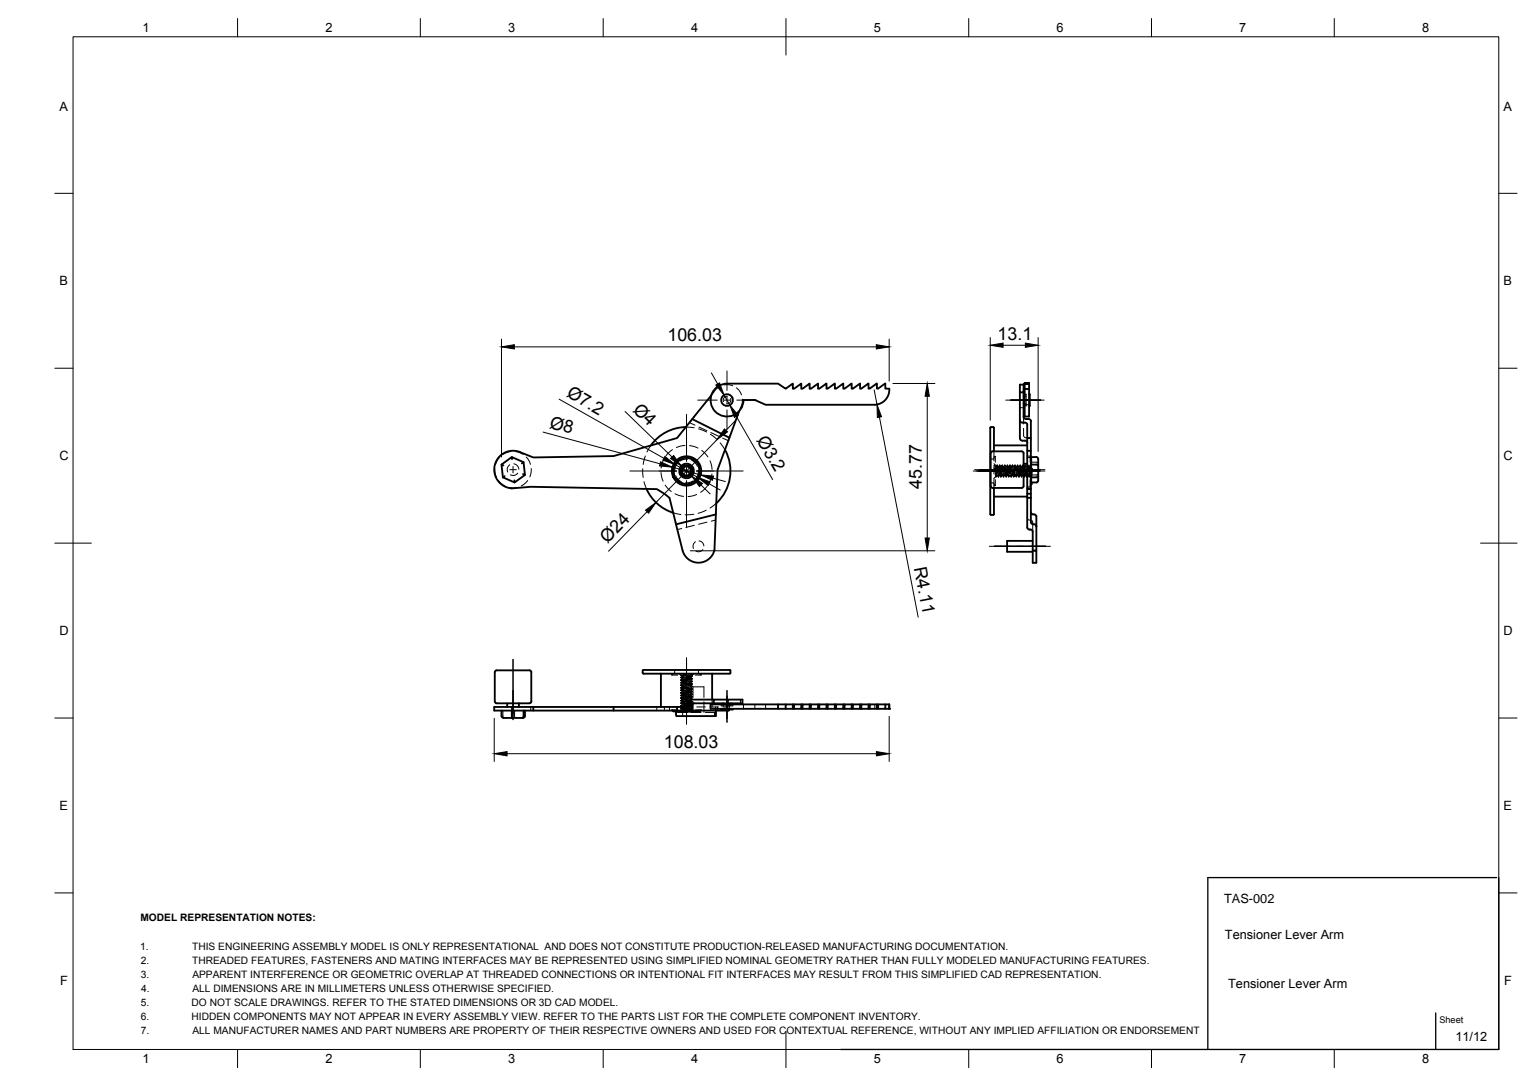
ISO-10303-21;
HEADER;
/* Generated by software containing ST-Developer
 * from STEP Tools, Inc. (www.steptools.com) 
 */

FILE_DESCRIPTION(
/* description */ ('STEP AP214'),
/* implementation_level */ '2;1');

FILE_NAME(
/* name */ 'Tensioner Lever Arm.step',
/* time_stamp */ '2026-11-04T19:38:14-08:00',
/* author */ (''),
/* organization */ (''),
/* preprocessor_version */ 'ST-DEVELOPER v20.2',
/* originating_system */ 'Autodesk Translation Framework v15.17.0.0',
/* authorisation */ '');

FILE_SCHEMA (('AUTOMOTIVE_DESIGN { 1 0 10303 214 3 1 1 }'));
ENDSEC;

DATA;
#10=MECHANICAL_DESIGN_GEOMETRIC_PRESENTATION_REPRESENTATION('',(#478),#36668);
#51=ORIENTED_CLOSED_SHELL('',*,#17801,.F.);
#52=BREP_WITH_VOIDS('Body1',#17802,(#51));
#136=(
BOUNDED_CURVE()
B_SPLINE_CURVE(2,(#34733,#34734,#34735,#34736,#34737,#34738,#34739),
 .UNSPECIFIED.,.F.,.F.)
B_SPLINE_CURVE_WITH_KNOTS((3,2,2,3),(0.964285714285714,0.976190476190476,
0.988095238095238,1.),.UNSPECIFIED.)
CURVE()
GEOMETRIC_REPRESENTATION_ITEM()
RATIONAL_B_SPLINE_CURVE((1.,0.866025403784439,1.,0.866025403784439,1.,0.866025403784439,
1.))
REPRESENTATION_ITEM('')
);
#137=(
BOUNDED_CURVE()
B_SPLINE_CURVE(2,(#34742,#34743,#34744,#34745,#34746,#34747,#34748),
 .UNSPECIFIED.,.F.,.F.)
B_SPLINE_CURVE_WITH_KNOTS((3,2,2,3),(0.964285714285714,0.976190476190476,
0.988095238095238,1.),.UNSPECIFIED.)
CURVE()
GEOMETRIC_REPRESENTATION_ITEM()
RATIONAL_B_SPLINE_CURVE((1.,0.866025403784439,1.,0.866025403784439,1.,0.866025403784439,
1.))
REPRESENTATION_ITEM('')
);
#138=(
BOUNDED_CURVE()
B_SPLINE_CURVE(2,(#34753,#34754,#34755,#34756,#34757,#34758,#34759,#34760,
#34761,#34762,#34763,#34764,#34765),.UNSPECIFIED.,.F.,.F.)
B_SPLINE_CURVE_WITH_KNOTS((3,2,2,2,2,2,3),(0.892857142857143,0.904761904761905,
0.916666666666667,0.928571428571429,0.94047619047619,0.952380952380952,
0.964285714285714),.UNSPECIFIED.)
CURVE()
GEOMETRIC_REPRESENTATION_ITEM()
RATIONAL_B_SPLINE_CURVE((1.,0.866025403784439,1.,0.866025403784439,1.,0.866025403784439,
1.,0.866025403784439,1.,0.866025403784439,1.,0.866025403784439,1.))
REPRESENTATION_ITEM('')
);
#139=(
BOUNDED_CURVE()
B_SPLINE_CURVE(2,(#34766,#34767,#34768,#34769,#34770,#34771,#34772,#34773,
#34774,#34775,#34776,#34777,#34778),.UNSPECIFIED.,.F.,.F.)
B_SPLINE_CURVE_WITH_KNOTS((3,2,2,2,2,2,3),(0.892857142857143,0.904761904761905,
0.916666666666667,0.928571428571429,0.94047619047619,0.952380952380952,
0.964285714285714),.UNSPECIFIED.)
CURVE()
GEOMETRIC_REPRESENTATION_ITEM()
RATIONAL_B_SPLINE_CURVE((1.,0.866025403784439,1.,0.866025403784439,1.,0.866025403784439,
1.,0.866025403784439,1.,0.866025403784439,1.,0.866025403784439,1.))
REPRESENTATION_ITEM('')
);
#140=(
BOUNDED_CURVE()
B_SPLINE_CURVE(2,(#34783,#34784,#34785,#34786,#34787,#34788,#34789,#34790,
#34791,#34792,#34793,#34794,#34795),.UNSPECIFIED.,.F.,.F.)
B_SPLINE_CURVE_WITH_KNOTS((3,2,2,2,2,2,3),(0.821428571428572,0.833333333333333,
0.845238095238095,0.857142857142857,0.869047619047619,0.880952380952381,
0.892857142857143),.UNSPECIFIED.)
CURVE()
GEOMETRIC_REPRESENTATION_ITEM()
RATIONAL_B_SPLINE_CURVE((1.,0.866025403784439,1.,0.866025403784439,1.,0.866025403784439,
1.,0.866025403784439,1.,0.866025403784439,1.,0.866025403784439,1.))
REPRESENTATION_ITEM('')
);
#141=(
BOUNDED_CURVE()
B_SPLINE_CURVE(2,(#34796,#34797,#34798,#34799,#34800,#34801,#34802,#34803,
#34804,#34805,#34806,#34807,#34808),.UNSPECIFIED.,.F.,.F.)
B_SPLINE_CURVE_WITH_KNOTS((3,2,2,2,2,2,3),(0.821428571428572,0.833333333333333,
0.845238095238095,0.857142857142857,0.869047619047619,0.880952380952381,
0.892857142857143),.UNSPECIFIED.)
CURVE()
GEOMETRIC_REPRESENTATION_ITEM()
RATIONAL_B_SPLINE_CURVE((1.,0.866025403784439,1.,0.866025403784439,1.,0.866025403784439,
1.,0.866025403784439,1.,0.866025403784439,1.,0.866025403784439,1.))
REPRESENTATION_ITEM('')
);
#142=(
BOUNDED_CURVE()
B_SPLINE_CURVE(2,(#34813,#34814,#34815,#34816,#34817,#34818,#34819,#34820,
#34821,#34822,#34823,#34824,#34825),.UNSPECIFIED.,.F.,.F.)
B_SPLINE_CURVE_WITH_KNOTS((3,2,2,2,2,2,3),(0.75,0.761904761904762,0.773809523809524,
0.785714285714286,0.797619047619048,0.809523809523809,0.821428571428572),
 .UNSPECIFIED.)
CURVE()
GEOMETRIC_REPRESENTATION_ITEM()
RATIONAL_B_SPLINE_CURVE((1.,0.866025403784439,1.,0.866025403784439,1.,0.866025403784439,
1.,0.866025403784439,1.,0.866025403784439,1.,0.866025403784439,1.))
REPRESENTATION_ITEM('')
);
#143=(
BOUNDED_CURVE()
B_SPLINE_CURVE(2,(#34826,#34827,#34828,#34829,#34830,#34831,#34832,#34833,
#34834,#34835,#34836,#34837,#34838),.UNSPECIFIED.,.F.,.F.)
B_SPLINE_CURVE_WITH_KNOTS((3,2,2,2,2,2,3),(0.75,0.761904761904762,0.773809523809524,
0.785714285714286,0.797619047619048,0.809523809523809,0.821428571428572),
 .UNSPECIFIED.)
CURVE()
GEOMETRIC_REPRESENTATION_ITEM()
RATIONAL_B_SPLINE_CURVE((1.,0.866025403784439,1.,0.866025403784439,1.,0.866025403784439,
1.,0.866025403784439,1.,0.866025403784439,1.,0.866025403784439,1.))
REPRESENTATION_ITEM('')
);
#144=(
BOUNDED_CURVE()
B_SPLINE_CURVE(2,(#34843,#34844,#34845,#34846,#34847,#34848,#34849,#34850,
#34851,#34852,#34853,#34854,#34855),.UNSPECIFIED.,.F.,.F.)
B_SPLINE_CURVE_WITH_KNOTS((3,2,2,2,2,2,3),(0.678571428571429,0.690476190476191,
0.702380952380952,0.714285714285714,0.726190476190476,0.738095238095238,
0.75),.UNSPECIFIED.)
CURVE()
GEOMETRIC_REPRESENTATION_ITEM()
RATIONAL_B_SPLINE_CURVE((1.,0.866025403784439,1.,0.866025403784439,1.,0.866025403784439,
1.,0.866025403784439,1.,0.866025403784439,1.,0.866025403784439,1.))
REPRESENTATION_ITEM('')
);
#145=(
BOUNDED_CURVE()
B_SPLINE_CURVE(2,(#34856,#34857,#34858,#34859,#34860,#34861,#34862,#34863,
#34864,#34865,#34866,#34867,#34868),.UNSPECIFIED.,.F.,.F.)
B_SPLINE_CURVE_WITH_KNOTS((3,2,2,2,2,2,3),(0.678571428571429,0.690476190476191,
0.702380952380952,0.714285714285714,0.726190476190476,0.738095238095238,
0.75),.UNSPECIFIED.)
CURVE()
GEOMETRIC_REPRESENTATION_ITEM()
RATIONAL_B_SPLINE_CURVE((1.,0.866025403784439,1.,0.866025403784439,1.,0.866025403784439,
1.,0.866025403784439,1.,0.866025403784439,1.,0.866025403784439,1.))
REPRESENTATION_ITEM('')
);
#146=(
BOUNDED_CURVE()
B_SPLINE_CURVE(2,(#34873,#34874,#34875,#34876,#34877,#34878,#34879,#34880,
#34881,#34882,#34883,#34884,#34885),.UNSPECIFIED.,.F.,.F.)
B_SPLINE_CURVE_WITH_KNOTS((3,2,2,2,2,2,3),(0.607142857142857,0.619047619047619,
0.630952380952381,0.642857142857143,0.654761904761905,0.666666666666667,
0.678571428571429),.UNSPECIFIED.)
CURVE()
GEOMETRIC_REPRESENTATION_ITEM()
RATIONAL_B_SPLINE_CURVE((1.,0.866025403784439,1.,0.866025403784439,1.,0.866025403784439,
1.,0.866025403784439,1.,0.866025403784439,1.,0.866025403784439,1.))
REPRESENTATION_ITEM('')
);
#147=(
BOUNDED_CURVE()
B_SPLINE_CURVE(2,(#34886,#34887,#34888,#34889,#34890,#34891,#34892,#34893,
#34894,#34895,#34896,#34897,#34898),.UNSPECIFIED.,.F.,.F.)
B_SPLINE_CURVE_WITH_KNOTS((3,2,2,2,2,2,3),(0.607142857142857,0.619047619047619,
0.630952380952381,0.642857142857143,0.654761904761905,0.666666666666667,
0.678571428571429),.UNSPECIFIED.)
CURVE()
GEOMETRIC_REPRESENTATION_ITEM()
RATIONAL_B_SPLINE_CURVE((1.,0.866025403784439,1.,0.866025403784439,1.,0.866025403784439,
1.,0.866025403784439,1.,0.866025403784439,1.,0.866025403784439,1.))
REPRESENTATION_ITEM('')
);
#148=(
BOUNDED_CURVE()
B_SPLINE_CURVE(2,(#34903,#34904,#34905,#34906,#34907,#34908,#34909,#34910,
#34911,#34912,#34913,#34914,#34915),.UNSPECIFIED.,.F.,.F.)
B_SPLINE_CURVE_WITH_KNOTS((3,2,2,2,2,2,3),(0.535714285714286,0.547619047619048,
0.55952380952381,0.571428571428571,0.583333333333333,0.595238095238095,
0.607142857142857),.UNSPECIFIED.)
CURVE()
GEOMETRIC_REPRESENTATION_ITEM()
RATIONAL_B_SPLINE_CURVE((1.,0.866025403784439,1.,0.866025403784439,1.,0.866025403784439,
1.,0.866025403784439,1.,0.866025403784439,1.,0.866025403784439,1.))
REPRESENTATION_ITEM('')
);
#149=(
BOUNDED_CURVE()
B_SPLINE_CURVE(2,(#34916,#34917,#34918,#34919,#34920,#34921,#34922,#34923,
#34924,#34925,#34926,#34927,#34928),.UNSPECIFIED.,.F.,.F.)
B_SPLINE_CURVE_WITH_KNOTS((3,2,2,2,2,2,3),(0.535714285714286,0.547619047619048,
0.55952380952381,0.571428571428571,0.583333333333333,0.595238095238095,
0.607142857142857),.UNSPECIFIED.)
CURVE()
GEOMETRIC_REPRESENTATION_ITEM()
RATIONAL_B_SPLINE_CURVE((1.,0.866025403784439,1.,0.866025403784439,1.,0.866025403784439,
1.,0.866025403784439,1.,0.866025403784439,1.,0.866025403784439,1.))
REPRESENTATION_ITEM('')
);
#150=(
BOUNDED_CURVE()
B_SPLINE_CURVE(2,(#34933,#34934,#34935,#34936,#34937,#34938,#34939,#34940,
#34941,#34942,#34943,#34944,#34945),.UNSPECIFIED.,.F.,.F.)
B_SPLINE_CURVE_WITH_KNOTS((3,2,2,2,2,2,3),(0.464285714285714,0.476190476190476,
0.488095238095238,0.5,0.511904761904762,0.523809523809524,0.535714285714286),
 .UNSPECIFIED.)
CURVE()
GEOMETRIC_REPRESENTATION_ITEM()
RATIONAL_B_SPLINE_CURVE((1.,0.866025403784439,1.,0.866025403784439,1.,0.866025403784439,
1.,0.866025403784439,1.,0.866025403784439,1.,0.866025403784439,1.))
REPRESENTATION_ITEM('')
);
#151=(
BOUNDED_CURVE()
B_SPLINE_CURVE(2,(#34946,#34947,#34948,#34949,#34950,#34951,#34952,#34953,
#34954,#34955,#34956,#34957,#34958),.UNSPECIFIED.,.F.,.F.)
B_SPLINE_CURVE_WITH_KNOTS((3,2,2,2,2,2,3),(0.464285714285714,0.476190476190476,
0.488095238095238,0.5,0.511904761904762,0.523809523809524,0.535714285714286),
 .UNSPECIFIED.)
CURVE()
GEOMETRIC_REPRESENTATION_ITEM()
RATIONAL_B_SPLINE_CURVE((1.,0.866025403784439,1.,0.866025403784439,1.,0.866025403784439,
1.,0.866025403784439,1.,0.866025403784439,1.,0.866025403784439,1.))
REPRESENTATION_ITEM('')
);
#152=(
BOUNDED_CURVE()
B_SPLINE_CURVE(2,(#34963,#34964,#34965,#34966,#34967,#34968,#34969,#34970,
#34971,#34972,#34973,#34974,#34975),.UNSPECIFIED.,.F.,.F.)
B_SPLINE_CURVE_WITH_KNOTS((3,2,2,2,2,2,3),(0.392857142857143,0.404761904761905,
0.416666666666667,0.428571428571428,0.44047619047619,0.452380952380952,
0.464285714285714),.UNSPECIFIED.)
CURVE()
GEOMETRIC_REPRESENTATION_ITEM()
RATIONAL_B_SPLINE_CURVE((1.,0.866025403784439,1.,0.866025403784439,1.,0.866025403784439,
1.,0.866025403784439,1.,0.866025403784439,1.,0.866025403784439,1.))
REPRESENTATION_ITEM('')
);
#153=(
BOUNDED_CURVE()
B_SPLINE_CURVE(2,(#34976,#34977,#34978,#34979,#34980,#34981,#34982,#34983,
#34984,#34985,#34986,#34987,#34988),.UNSPECIFIED.,.F.,.F.)
B_SPLINE_CURVE_WITH_KNOTS((3,2,2,2,2,2,3),(0.392857142857143,0.404761904761905,
0.416666666666667,0.428571428571428,0.44047619047619,0.452380952380952,
0.464285714285714),.UNSPECIFIED.)
CURVE()
GEOMETRIC_REPRESENTATION_ITEM()
RATIONAL_B_SPLINE_CURVE((1.,0.866025403784439,1.,0.866025403784439,1.,0.866025403784439,
1.,0.866025403784439,1.,0.866025403784439,1.,0.866025403784439,1.))
REPRESENTATION_ITEM('')
);
#154=(
BOUNDED_CURVE()
B_SPLINE_CURVE(2,(#34993,#34994,#34995,#34996,#34997,#34998,#34999,#35000,
#35001,#35002,#35003,#35004,#35005),.UNSPECIFIED.,.F.,.F.)
B_SPLINE_CURVE_WITH_KNOTS((3,2,2,2,2,2,3),(0.321428571428572,0.333333333333334,
0.345238095238096,0.357142857142857,0.369047619047619,0.380952380952381,
0.392857142857143),.UNSPECIFIED.)
CURVE()
GEOMETRIC_REPRESENTATION_ITEM()
RATIONAL_B_SPLINE_CURVE((1.,0.866025403784439,1.,0.866025403784439,1.,0.866025403784439,
1.,0.866025403784439,1.,0.866025403784439,1.,0.866025403784439,1.))
REPRESENTATION_ITEM('')
);
#155=(
BOUNDED_CURVE()
B_SPLINE_CURVE(2,(#35006,#35007,#35008,#35009,#35010,#35011,#35012,#35013,
#35014,#35015,#35016,#35017,#35018),.UNSPECIFIED.,.F.,.F.)
B_SPLINE_CURVE_WITH_KNOTS((3,2,2,2,2,2,3),(0.321428571428572,0.333333333333334,
0.345238095238096,0.357142857142857,0.369047619047619,0.380952380952381,
0.392857142857143),.UNSPECIFIED.)
CURVE()
GEOMETRIC_REPRESENTATION_ITEM()
RATIONAL_B_SPLINE_CURVE((1.,0.866025403784439,1.,0.866025403784439,1.,0.866025403784439,
1.,0.866025403784439,1.,0.866025403784439,1.,0.866025403784439,1.))
REPRESENTATION_ITEM('')
);
#156=(
BOUNDED_CURVE()
B_SPLINE_CURVE(2,(#35023,#35024,#35025,#35026,#35027,#35028,#35029,#35030,
#35031,#35032,#35033,#35034,#35035),.UNSPECIFIED.,.F.,.F.)
B_SPLINE_CURVE_WITH_KNOTS((3,2,2,2,2,2,3),(0.25,0.261904761904762,0.273809523809524,
0.285714285714286,0.297619047619048,0.309523809523809,0.321428571428572),
 .UNSPECIFIED.)
CURVE()
GEOMETRIC_REPRESENTATION_ITEM()
RATIONAL_B_SPLINE_CURVE((1.,0.866025403784439,1.,0.866025403784439,1.,0.866025403784439,
1.,0.866025403784439,1.,0.866025403784439,1.,0.866025403784439,1.))
REPRESENTATION_ITEM('')
);
#157=(
BOUNDED_CURVE()
B_SPLINE_CURVE(2,(#35036,#35037,#35038,#35039,#35040,#35041,#35042,#35043,
#35044,#35045,#35046,#35047,#35048),.UNSPECIFIED.,.F.,.F.)
B_SPLINE_CURVE_WITH_KNOTS((3,2,2,2,2,2,3),(0.25,0.261904761904762,0.273809523809524,
0.285714285714286,0.297619047619048,0.309523809523809,0.321428571428572),
 .UNSPECIFIED.)
CURVE()
GEOMETRIC_REPRESENTATION_ITEM()
RATIONAL_B_SPLINE_CURVE((1.,0.866025403784439,1.,0.866025403784439,1.,0.866025403784439,
1.,0.866025403784439,1.,0.866025403784439,1.,0.866025403784439,1.))
REPRESENTATION_ITEM('')
);
#158=(
BOUNDED_CURVE()
B_SPLINE_CURVE(2,(#35053,#35054,#35055,#35056,#35057,#35058,#35059,#35060,
#35061,#35062,#35063,#35064,#35065),.UNSPECIFIED.,.F.,.F.)
B_SPLINE_CURVE_WITH_KNOTS((3,2,2,2,2,2,3),(0.178571428571428,0.19047619047619,
0.202380952380952,0.214285714285714,0.226190476190476,0.238095238095238,
0.25),.UNSPECIFIED.)
CURVE()
GEOMETRIC_REPRESENTATION_ITEM()
RATIONAL_B_SPLINE_CURVE((1.,0.866025403784439,1.,0.866025403784439,1.,0.866025403784439,
1.,0.866025403784439,1.,0.866025403784439,1.,0.866025403784439,1.))
REPRESENTATION_ITEM('')
);
#159=(
BOUNDED_CURVE()
B_SPLINE_CURVE(2,(#35066,#35067,#35068,#35069,#35070,#35071,#35072,#35073,
#35074,#35075,#35076,#35077,#35078),.UNSPECIFIED.,.F.,.F.)
B_SPLINE_CURVE_WITH_KNOTS((3,2,2,2,2,2,3),(0.178571428571428,0.19047619047619,
0.202380952380952,0.214285714285714,0.226190476190476,0.238095238095238,
0.25),.UNSPECIFIED.)
CURVE()
GEOMETRIC_REPRESENTATION_ITEM()
RATIONAL_B_SPLINE_CURVE((1.,0.866025403784439,1.,0.866025403784439,1.,0.866025403784439,
1.,0.866025403784439,1.,0.866025403784439,1.,0.866025403784439,1.))
REPRESENTATION_ITEM('')
);
#160=(
BOUNDED_CURVE()
B_SPLINE_CURVE(2,(#35083,#35084,#35085,#35086,#35087,#35088,#35089,#35090,
#35091,#35092,#35093,#35094,#35095),.UNSPECIFIED.,.F.,.F.)
B_SPLINE_CURVE_WITH_KNOTS((3,2,2,2,2,2,3),(0.107142857142857,0.119047619047619,
0.130952380952381,0.142857142857143,0.154761904761905,0.166666666666667,
0.178571428571428),.UNSPECIFIED.)
CURVE()
GEOMETRIC_REPRESENTATION_ITEM()
RATIONAL_B_SPLINE_CURVE((1.,0.866025403784439,1.,0.866025403784439,1.,0.866025403784439,
1.,0.866025403784439,1.,0.866025403784439,1.,0.866025403784439,1.))
REPRESENTATION_ITEM('')
);
#161=(
BOUNDED_CURVE()
B_SPLINE_CURVE(2,(#35096,#35097,#35098,#35099,#35100,#35101,#35102,#35103,
#35104,#35105,#35106,#35107,#35108),.UNSPECIFIED.,.F.,.F.)
B_SPLINE_CURVE_WITH_KNOTS((3,2,2,2,2,2,3),(0.107142857142857,0.119047619047619,
0.130952380952381,0.142857142857143,0.154761904761905,0.166666666666667,
0.178571428571428),.UNSPECIFIED.)
CURVE()
GEOMETRIC_REPRESENTATION_ITEM()
RATIONAL_B_SPLINE_CURVE((1.,0.866025403784439,1.,0.866025403784439,1.,0.866025403784439,
1.,0.866025403784439,1.,0.866025403784439,1.,0.866025403784439,1.))
REPRESENTATION_ITEM('')
);
#162=(
BOUNDED_CURVE()
B_SPLINE_CURVE(2,(#35114,#35115,#35116,#35117,#35118,#35119,#35120),
 .UNSPECIFIED.,.F.,.F.)
B_SPLINE_CURVE_WITH_KNOTS((3,2,2,3),(0.,0.0119047619047619,0.0238095238095238,
0.0357142857142857),.UNSPECIFIED.)
CURVE()
GEOMETRIC_REPRESENTATION_ITEM()
RATIONAL_B_SPLINE_CURVE((1.,0.866025403784439,1.,0.866025403784439,1.,0.866025403784439,
1.))
REPRESENTATION_ITEM('')
);
#163=(
BOUNDED_CURVE()
B_SPLINE_CURVE(2,(#35123,#35124,#35125,#35126,#35127,#35128,#35129),
 .UNSPECIFIED.,.F.,.F.)
B_SPLINE_CURVE_WITH_KNOTS((3,2,2,3),(0.,0.0119047619047619,0.0238095238095238,
0.0357142857142857),.UNSPECIFIED.)
CURVE()
GEOMETRIC_REPRESENTATION_ITEM()
RATIONAL_B_SPLINE_CURVE((1.,0.866025403784439,1.,0.866025403784439,1.,0.866025403784439,
1.))
REPRESENTATION_ITEM('')
);
#164=(
BOUNDED_CURVE()
B_SPLINE_CURVE(2,(#35193,#35194,#35195,#35196,#35197,#35198,#35199,#35200,
#35201,#35202,#35203,#35204,#35205),.UNSPECIFIED.,.F.,.F.)
B_SPLINE_CURVE_WITH_KNOTS((3,2,2,2,2,2,3),(0.,0.0119047619047619,0.0238095238095238,
0.0357142857142857,0.0476190476190476,0.0595238095238095,0.0626545676342116),
 .UNSPECIFIED.)
CURVE()
GEOMETRIC_REPRESENTATION_ITEM()
RATIONAL_B_SPLINE_CURVE((1.,0.866025403784439,1.,0.866025403784439,1.,0.866025403784439,
1.,0.866025403784439,1.,0.866025403784439,1.,0.964766867490064,0.948065212760667))
REPRESENTATION_ITEM('')
);
#165=(
BOUNDED_CURVE()
B_SPLINE_CURVE(2,(#35549,#35550,#35551,#35552,#35553,#35554,#35555,#35556,
#35557,#35558,#35559,#35560,#35561),.UNSPECIFIED.,.F.,.F.)
B_SPLINE_CURVE_WITH_KNOTS((3,2,2,2,2,2,3),(0.0357142857142857,0.0476190476190476,
0.0595238095238095,0.0714285714285714,0.0833333333333333,0.0952380952380952,
0.107142857142857),.UNSPECIFIED.)
CURVE()
GEOMETRIC_REPRESENTATION_ITEM()
RATIONAL_B_SPLINE_CURVE((1.,0.866025403784439,1.,0.866025403784439,1.,0.866025403784439,
1.,0.866025403784439,1.,0.866025403784439,1.,0.866025403784439,1.))
REPRESENTATION_ITEM('')
);
#166=(
BOUNDED_CURVE()
B_SPLINE_CURVE(2,(#35600,#35601,#35602,#35603,#35604,#35605,#35606,#35607,
#35608,#35609,#35610,#35611,#35612),.UNSPECIFIED.,.F.,.F.)
B_SPLINE_CURVE_WITH_KNOTS((3,2,2,2,2,2,3),(0.0357142857142857,0.0476190476190476,
0.0595238095238095,0.0714285714285714,0.0833333333333333,0.0952380952380952,
0.107142857142857),.UNSPECIFIED.)
CURVE()
GEOMETRIC_REPRESENTATION_ITEM()
RATIONAL_B_SPLINE_CURVE((1.,0.866025403784439,1.,0.866025403784439,1.,0.866025403784439,
1.,0.866025403784439,1.,0.866025403784439,1.,0.866025403784439,1.))
REPRESENTATION_ITEM('')
);
#167=(
BOUNDED_CURVE()
B_SPLINE_CURVE(2,(#35989,#35990,#35991,#35992,#35993,#35994,#35995),
 .UNSPECIFIED.,.F.,.F.)
B_SPLINE_CURVE_WITH_KNOTS((3,2,2,3),(0.96944370253851,0.976190476190476,
0.988095238095238,1.),.UNSPECIFIED.)
CURVE()
GEOMETRIC_REPRESENTATION_ITEM()
RATIONAL_B_SPLINE_CURVE((0.934205814715249,0.924072712834481,1.,0.866025403784439,
1.,0.866025403784439,1.))
REPRESENTATION_ITEM('')
);
#189=CONICAL_SURFACE('',#19172,4.,0.785398163397449);
#190=CONICAL_SURFACE('',#19250,1.6,0.78539816339745);
#191=CONICAL_SURFACE('',#19252,2.,0.785398163397445);
#192=CONICAL_SURFACE('',#19253,3.6,0.785398163397445);
#230=TOROIDAL_SURFACE('',#19215,11.8,0.2);
#231=TOROIDAL_SURFACE('',#19220,11.8,0.2);
#232=TOROIDAL_SURFACE('',#19225,3.45,0.2);
#233=TOROIDAL_SURFACE('',#19230,3.45,0.2);
#234=TOROIDAL_SURFACE('',#19260,4.5,0.5);
#235=TOROIDAL_SURFACE('',#19264,4.5,0.5);
#357=B_SPLINE_CURVE_WITH_KNOTS('',3,(#33774,#33775,#33776,#33777,#33778,
#33779,#33780,#33781,#33782,#33783,#33784,#33785,#33786,#33787,#33788,#33789,
#33790,#33791,#33792,#33793,#33794,#33795),.UNSPECIFIED.,.F.,.F.,(4,2,2,
2,2,2,2,2,2,2,4),(13.142711462932,13.1579818167511,13.2217062873234,13.2838063508681,
13.3455231362043,13.4092932791525,13.4706620157354,13.5344323685447,13.5973377391588,
13.657787218639,13.7194997062356),.UNSPECIFIED.);
#358=B_SPLINE_CURVE_WITH_KNOTS('',3,(#33800,#33801,#33802,#33803,#33804,
#33805,#33806,#33807,#33808,#33809,#33810,#33811,#33812,#33813,#33814,#33815,
#33816,#33817,#33818,#33819,#33820,#33821,#33822,#33823,#33824,#33825,#33826,
#33827,#33828,#33829,#33830,#33831,#33832,#33833,#33834,#33835),
 .UNSPECIFIED.,.F.,.F.,(4,2,2,2,2,2,2,2,2,2,2,2,2,2,2,2,2,4),(0.,0.0359582530012615,
0.0731837666941684,0.137235112949865,0.198838631694034,0.261200010699037,
0.32504770195871,0.386000749088701,0.44904001871335,0.513045713500326,0.574549640221195,
0.638459422251555,0.700373110277162,0.762611164523284,0.826498988256686,
0.887523750164669,0.950449850339167,1.01090153686108),.UNSPECIFIED.);
#359=B_SPLINE_CURVE_WITH_KNOTS('',3,(#33836,#33837,#33838,#33839,#33840,
#33841,#33842,#33843,#33844,#33845,#33846,#33847,#33848,#33849,#33850,#33851,
#33852,#33853,#33854,#33855,#33856,#33857,#33858,#33859,#33860,#33861,#33862,
#33863,#33864,#33865,#33866,#33867,#33868,#33869,#33870,#33871),
 .UNSPECIFIED.,.F.,.F.,(4,2,2,2,2,2,2,2,2,2,2,2,2,2,2,2,2,4),(12.1323404141985,
12.1556573917594,12.2200847211504,12.2820653373017,12.3447227235141,12.4083318674643,
12.4695568071821,12.5333442349376,12.5960689705528,12.6570830861283,12.7215467187269,
12.7835529410482,12.8457066305132,12.9093617916751,12.9706262125415,13.0343352675459,
13.0971204251574,13.142711462932),.UNSPECIFIED.);
#360=B_SPLINE_CURVE_WITH_KNOTS('',3,(#33876,#33877,#33878,#33879,#33880,
#33881,#33882,#33883,#33884,#33885,#33886,#33887,#33888,#33889,#33890,#33891,
#33892,#33893,#33894,#33895,#33896,#33897,#33898,#33899,#33900,#33901,#33902,
#33903,#33904,#33905,#33906,#33907,#33908,#33909,#33910,#33911,#33912,#33913),
 .UNSPECIFIED.,.F.,.F.,(4,2,2,2,2,2,2,2,2,2,2,2,2,2,2,2,2,2,4),(1.01090153686108,
1.01432125508311,1.07572564016303,1.13952547317396,1.20189435909138,1.26404402197446,
1.32865534671711,1.38984758335372,1.45271798203398,1.51661625113869,1.57780436811715,
1.64131392739509,1.70396013741204,1.76584688882252,1.83017529548686,1.89140309254637,
1.95401157225196,2.01781915854794,2.02253426878796),.UNSPECIFIED.);
#361=B_SPLINE_CURVE_WITH_KNOTS('',3,(#33914,#33915,#33916,#33917,#33918,
#33919,#33920,#33921,#33922,#33923,#33924,#33925,#33926,#33927,#33928,#33929,
#33930,#33931,#33932,#33933,#33934,#33935,#33936,#33937,#33938,#33939,#33940,
#33941,#33942,#33943,#33944,#33945,#33946,#33947,#33948,#33949),
 .UNSPECIFIED.,.F.,.F.,(4,2,2,2,2,2,2,2,2,2,2,2,2,2,2,2,2,4),(11.1214864347725,
11.1534488115465,11.2174503566185,11.2790374548038,11.3425714444984,11.4057227010986,
11.4666734207028,11.5305054568745,11.5929885337885,11.6543942371259,11.7185819722754,
11.7803406867599,11.843382214289,11.9067390545548,11.9678030898047,12.0316809910961,
12.0943838071615,12.1323404141985),.UNSPECIFIED.);
#362=B_SPLINE_CURVE_WITH_KNOTS('',3,(#33954,#33955,#33956,#33957,#33958,
#33959,#33960,#33961,#33962,#33963,#33964,#33965,#33966,#33967,#33968,#33969,
#33970,#33971,#33972,#33973,#33974,#33975,#33976,#33977,#33978,#33979,#33980,
#33981,#33982,#33983,#33984,#33985,#33986,#33987,#33988,#33989),
 .UNSPECIFIED.,.F.,.F.,(4,2,2,2,2,2,2,2,2,2,2,2,2,2,2,2,2,4),(2.02253426878796,
2.07880223700639,2.14206634117737,2.20511331401215,2.26678551297205,2.33088212000521,
2.39225776527954,2.45465411191018,2.51842320109549,2.57930873182499,2.64237446317126,
2.70592714775301,2.76743537711405,2.83135393252775,2.89298050251894,2.95521750681276,
3.01899659602717,3.03218372263281),.UNSPECIFIED.);
#363=B_SPLINE_CURVE_WITH_KNOTS('',3,(#33990,#33991,#33992,#33993,#33994,
#33995,#33996,#33997,#33998,#33999,#34000,#34001,#34002,#34003,#34004,#34005,
#34006,#34007,#34008,#34009,#34010,#34011,#34012,#34013,#34014,#34015,#34016,
#34017,#34018,#34019,#34020,#34021,#34022,#34023,#34024,#34025),
 .UNSPECIFIED.,.F.,.F.,(4,2,2,2,2,2,2,2,2,2,2,2,2,2,2,2,2,4),(10.1102829969334,
10.1512710656532,10.2150405861368,10.2764168243332,10.3402833928885,10.4031768398644,
10.464210597169,10.5280949109509,10.5902986361653,10.6522671409988,10.716138589806,
10.7776067824405,10.8417158948343,10.9047115085251,10.9656552090866,11.0294904215152,
11.0918061543416,11.1214864347725),.UNSPECIFIED.);
#364=B_SPLINE_CURVE_WITH_KNOTS('',3,(#34030,#34031,#34032,#34033,#34034,
#34035,#34036,#34037,#34038,#34039,#34040,#34041,#34042,#34043,#34044,#34045,
#34046,#34047,#34048,#34049,#34050,#34051,#34052,#34053,#34054,#34055,#34056,
#34057,#34058,#34059,#34060,#34061,#34062,#34063,#34064,#34065),
 .UNSPECIFIED.,.F.,.F.,(4,2,2,2,2,2,2,2,2,2,2,2,2,2,2,2,2,4),(3.03218372263281,
3.07988992137784,3.14280768521512,3.20694447876217,3.26834173965761,3.33213864733873,
3.39410160796508,3.45623492856705,3.52006950765413,3.581065702496,3.643889407597,
3.70770538153846,3.76901632572646,3.83271726992244,3.89517799562774,3.95723784182379,
4.02175232938853,4.04294907391778),.UNSPECIFIED.);
#365=B_SPLINE_CURVE_WITH_KNOTS('',3,(#34066,#34067,#34068,#34069,#34070,
#34071,#34072,#34073,#34074,#34075,#34076,#34077,#34078,#34079,#34080,#34081,
#34082,#34083,#34084,#34085,#34086,#34087,#34088,#34089,#34090,#34091,#34092,
#34093,#34094,#34095,#34096,#34097,#34098,#34099,#34100,#34101),
 .UNSPECIFIED.,.F.,.F.,(4,2,2,2,2,2,2,2,2,2,2,2,2,2,2,2,2,4),(9.09888760056311,
9.1486061892843,9.21185845597294,9.27284452328484,9.3366736185903,9.39926683177369,
9.46054865914562,9.52485851951026,9.58672926579225,9.6494821976632,9.71297048300282,
9.77413960104805,9.8380482486443,9.90089339572085,9.96211589511406,10.0266983935914,
10.0888222946518,10.1102829969334),.UNSPECIFIED.);
#366=B_SPLINE_CURVE_WITH_KNOTS('',3,(#34106,#34107,#34108,#34109,#34110,
#34111,#34112,#34113,#34114,#34115,#34116,#34117,#34118,#34119,#34120,#34121,
#34122,#34123,#34124,#34125,#34126,#34127,#34128,#34129,#34130,#34131,#34132,
#34133,#34134,#34135,#34136,#34137,#34138,#34139,#34140,#34141),
 .UNSPECIFIED.,.F.,.F.,(4,2,2,2,2,2,2,2,2,2,2,2,2,2,2,2,2,4),(4.04294907391778,
4.08295248441981,4.14573340606041,4.20960220268779,4.27071419165295,4.33414048671887,
4.3969237015339,4.45873747459545,4.52298680052707,4.58426283261112,4.64679908242436,
4.71059608911083,4.77154071334328,4.83473784914837,4.89796160798484,4.95957841423839,
5.02361460467017,5.05338907499331),.UNSPECIFIED.);
#367=B_SPLINE_CURVE_WITH_KNOTS('',3,(#34142,#34143,#34144,#34145,#34146,
#34147,#34148,#34149,#34150,#34151,#34152,#34153,#34154,#34155,#34156,#34157,
#34158,#34159,#34160,#34161,#34162,#34163,#34164,#34165,#34166,#34167,#34168,
#34169,#34170,#34171,#34172,#34173,#34174,#34175,#34176,#34177),
 .UNSPECIFIED.,.F.,.F.,(4,2,2,2,2,2,2,2,2,2,2,2,2,2,2,2,2,4),(8.08870409001179,
8.14726255440374,8.21018942134961,8.27112892082392,8.33494956046087,8.3971931878043,
8.45891604108485,8.52283831070216,8.58435148775943,8.64805373114709,8.7111177098161,
8.77202855807641,8.83582950764207,8.89822120139655,8.9596733109505,9.02376220375112,
9.08542860886895,9.09888760056311),.UNSPECIFIED.);
#368=B_SPLINE_CURVE_WITH_KNOTS('',3,(#34182,#34183,#34184,#34185,#34186,
#34187,#34188,#34189,#34190,#34191,#34192,#34193,#34194,#34195,#34196,#34197,
#34198,#34199,#34200,#34201,#34202,#34203,#34204,#34205,#34206,#34207,#34208,
#34209,#34210,#34211,#34212,#34213,#34214,#34215,#34216,#34217),
 .UNSPECIFIED.,.F.,.F.,(4,2,2,2,2,2,2,2,2,2,2,2,2,2,2,2,2,4),(5.05338907499331,
5.08507620655147,5.14741861117407,5.21119465800221,5.27207967609426,5.33509582780477,
5.39885641679272,5.46032770589982,5.52420548109823,5.58595101557381,5.64815344503229,
5.71195588741959,5.77288385429669,5.83577070173323,5.90013604798391,5.96151561074328,
6.02529220384508,6.06339547208752),.UNSPECIFIED.);
#369=B_SPLINE_CURVE_WITH_KNOTS('',3,(#34218,#34219,#34220,#34221,#34222,
#34223,#34224,#34225,#34226,#34227,#34228,#34229,#34230,#34231,#34232,#34233,
#34234,#34235,#34236,#34237,#34238,#34239,#34240,#34241,#34242,#34243,#34244,
#34245,#34246,#34247,#34248,#34249,#34250,#34251,#34252,#34253,#34254,#34255),
 .UNSPECIFIED.,.F.,.F.,(4,2,2,2,2,2,2,2,2,2,2,2,2,2,2,2,2,2,4),(7.07669856726943,
7.07954003474363,7.1434735852899,7.20628315126754,7.26756956135512,7.33211069661312,
7.39419805791722,7.45679558005713,7.52052067995683,7.58185584046079,7.64572141384328,
7.70856576164337,7.76962609572472,7.83351139916469,7.89566314676714,7.95773731224237,
8.02154988815528,8.08296333620691,8.08870409001179),.UNSPECIFIED.);
#370=B_SPLINE_CURVE_WITH_KNOTS('',3,(#34260,#34261,#34262,#34263,#34264,
#34265,#34266,#34267,#34268,#34269,#34270,#34271,#34272,#34273,#34274,#34275,
#34276,#34277,#34278,#34279,#34280,#34281,#34282,#34283,#34284,#34285,#34286,
#34287,#34288,#34289,#34290,#34291,#34292,#34293,#34294,#34295),
 .UNSPECIFIED.,.F.,.F.,(4,2,2,2,2,2,2,2,2,2,2,2,2,2,2,2,2,4),(6.06339547208752,
6.08739865938769,6.14951759655391,6.21339102568026,6.27445189976627,6.3372644413378,
6.40111747590033,6.46242451331744,6.52611972557013,6.58876676321737,6.65082781566915,
6.71534028879468,6.77664248685867,6.83942599924069,6.90335733851185,6.96448924397403,
7.02753578823382,7.07536902408054),.UNSPECIFIED.);
#371=B_SPLINE_CURVE_WITH_KNOTS('',3,(#34296,#34297,#34298,#34299,#34300,
#34301,#34302,#34303,#34304,#34305,#34306,#34307,#34308,#34309,#34310,#34311,
#34312,#34313,#34314,#34315,#34316,#34317,#34318,#34319,#34320,#34321,#34322,
#34323,#34324,#34325,#34326,#34327,#34328,#34329,#34330,#34331),
 .UNSPECIFIED.,.F.,.F.,(4,2,2,2,2,2,2,2,2,2,2,2,2,2,2,2,2,4),(6.06541653120124,
6.07677442400661,6.140635558073,6.20302675441035,6.26461868394941,6.32870208754262,
6.39036582549154,6.45377413212297,6.5170133202156,6.57801697113455,6.64188924343672,
6.70446387260813,6.76584913304758,6.83013508929954,6.89198582955554,6.95493147688094,
7.01839062339183,7.07669856726943),.UNSPECIFIED.);
#372=B_SPLINE_CURVE_WITH_KNOTS('',3,(#34336,#34337,#34338,#34339,#34340,
#34341,#34342,#34343,#34344,#34345,#34346,#34347,#34348,#34349,#34350,#34351,
#34352,#34353,#34354,#34355,#34356,#34357,#34358,#34359,#34360,#34361,#34362,
#34363,#34364,#34365,#34366,#34367,#34368,#34369,#34370,#34371),
 .UNSPECIFIED.,.F.,.F.,(4,2,2,2,2,2,2,2,2,2,2,2,2,2,2,2,2,4),(7.07536902408054,
7.08855245102283,7.15246092273268,7.21482540085779,7.27657501529124,7.34062459821103,
7.402258864083,7.46593663852235,7.52913183820682,7.59014144323236,7.6540402424552,
7.7165647897316,7.77806368679493,7.84229209213344,7.90409104519249,7.96726276848113,
8.03065710497116,8.08707212644807),.UNSPECIFIED.);
#373=B_SPLINE_CURVE_WITH_KNOTS('',3,(#34372,#34373,#34374,#34375,#34376,
#34377,#34378,#34379,#34380,#34381,#34382,#34383,#34384,#34385,#34386,#34387,
#34388,#34389,#34390,#34391,#34392,#34393,#34394,#34395,#34396,#34397,#34398,
#34399,#34400,#34401,#34402,#34403,#34404,#34405,#34406,#34407),
 .UNSPECIFIED.,.F.,.F.,(4,2,2,2,2,2,2,2,2,2,2,2,2,2,2,2,2,4),(5.05358007064663,
5.07526698797775,5.13742262368034,5.20203867290101,5.26327685292802,5.32615387985161,
5.39008500223115,5.45128337214047,5.51423293972763,5.57526080610153,5.63915760440498,
5.70141990187991,5.76331389421934,5.82725008327323,5.88877883217346,5.95274084875297,
6.01580899199089,6.06541653120124),.UNSPECIFIED.);
#374=B_SPLINE_CURVE_WITH_KNOTS('',3,(#34412,#34413,#34414,#34415,#34416,
#34417,#34418,#34419,#34420,#34421,#34422,#34423,#34424,#34425,#34426,#34427,
#34428,#34429,#34430,#34431,#34432,#34433,#34434,#34435,#34436,#34437,#34438,
#34439,#34440,#34441,#34442,#34443,#34444,#34445,#34446,#34447,#34448,#34449),
 .UNSPECIFIED.,.F.,.F.,(4,2,2,2,2,2,2,2,2,2,2,2,2,2,2,2,2,2,4),(8.08707212644807,
8.09176525665677,8.15570300420656,8.2184404959072,8.27979205065832,8.34425311543039,
8.40626742353619,8.46903842955182,8.53267905944031,8.59399344981126,8.65802246642909,
8.72102276848788,8.78233953906217,8.84708446711847,8.90936257261165,8.97185664997878,
9.03578847048786,9.0973198504176,9.10077482354646),.UNSPECIFIED.);
#375=B_SPLINE_CURVE_WITH_KNOTS('',3,(#34450,#34451,#34452,#34453,#34454,
#34455,#34456,#34457,#34458,#34459,#34460,#34461,#34462,#34463,#34464,#34465,
#34466,#34467,#34468,#34469,#34470,#34471,#34472,#34473,#34474,#34475,#34476,
#34477,#34478,#34479,#34480,#34481,#34482,#34483,#34484,#34485),
 .UNSPECIFIED.,.F.,.F.,(4,2,2,2,2,2,2,2,2,2,2,2,2,2,2,2,2,4),(4.04194870124897,
4.07186646906384,4.1342195762872,4.19808356758159,4.25905380820392,4.32208652116032,
4.38619220152751,4.44769467094645,4.51160206611549,4.57357977415333,4.63581766762807,
4.69972829162907,4.76078357675388,4.82371100529867,4.88760423328709,4.94901258493515,
5.01281576269777,5.05358007064663),.UNSPECIFIED.);
#376=B_SPLINE_CURVE_WITH_KNOTS('',3,(#34490,#34491,#34492,#34493,#34494,
#34495,#34496,#34497,#34498,#34499,#34500,#34501,#34502,#34503,#34504,#34505,
#34506,#34507,#34508,#34509,#34510,#34511,#34512,#34513,#34514,#34515,#34516,
#34517,#34518,#34519,#34520,#34521,#34522,#34523,#34524,#34525),
 .UNSPECIFIED.,.F.,.F.,(4,2,2,2,2,2,2,2,2,2,2,2,2,2,2,2,2,4),(9.10077482354646,
9.16132248678141,9.22437885995756,9.28552855679668,9.34954759714026,9.41191457245069,
9.47395340314661,9.53799567643849,9.59962706543561,9.6637604846617,9.72693064242749,
9.78800913033544,9.85198827170404,9.91447921930853,9.97620780906414,10.0403923367931,
10.1021540483061,10.1138813028186),.UNSPECIFIED.);
#377=B_SPLINE_CURVE_WITH_KNOTS('',3,(#34526,#34527,#34528,#34529,#34530,
#34531,#34532,#34533,#34534,#34535,#34536,#34537,#34538,#34539,#34540,#34541,
#34542,#34543,#34544,#34545,#34546,#34547,#34548,#34549,#34550,#34551,#34552,
#34553,#34554,#34555,#34556,#34557,#34558,#34559,#34560,#34561),
 .UNSPECIFIED.,.F.,.F.,(4,2,2,2,2,2,2,2,2,2,2,2,2,2,2,2,2,4),(3.03058177228639,
3.06878888879999,3.13153509824144,3.19544728706079,3.25654971334623,3.31994938600095,
3.38299624598465,3.4447952445736,3.50902532068632,3.57044982999391,3.63297336418729,
3.69683682410905,3.75781984354876,3.821011153871,3.88454527977345,3.94616971252482,
4.01021045952113,4.04194870124897),.UNSPECIFIED.);
#378=B_SPLINE_CURVE_WITH_KNOTS('',3,(#34566,#34567,#34568,#34569,#34570,
#34571,#34572,#34573,#34574,#34575,#34576,#34577,#34578,#34579,#34580,#34581,
#34582,#34583,#34584,#34585,#34586,#34587,#34588,#34589,#34590,#34591,#34592,
#34593,#34594,#34595,#34596,#34597,#34598,#34599,#34600,#34601),
 .UNSPECIFIED.,.F.,.F.,(4,2,2,2,2,2,2,2,2,2,2,2,2,2,2,2,2,4),(10.1138813028186,
10.1657257783372,10.2290626094574,10.2901697019842,10.354155562403,10.416825378446,
10.4783374500112,10.5427199165038,10.6046642836855,10.6677630192165,10.7313158447778,
10.7925589963334,10.8566014704575,10.9195020342268,10.9809047381247,11.0455381116102,
11.1077150533666,11.1275070958942),.UNSPECIFIED.);
#379=B_SPLINE_CURVE_WITH_KNOTS('',3,(#34602,#34603,#34604,#34605,#34606,
#34607,#34608,#34609,#34610,#34611,#34612,#34613,#34614,#34615,#34616,#34617,
#34618,#34619,#34620,#34621,#34622,#34623,#34624,#34625,#34626,#34627,#34628,
#34629,#34630,#34631,#34632,#34633,#34634,#34635,#34636,#34637),
 .UNSPECIFIED.,.F.,.F.,(4,2,2,2,2,2,2,2,2,2,2,2,2,2,2,2,2,4),(2.01959218604488,
2.06541546347494,2.12825385027516,2.19265393585692,2.25399031389628,2.31772144326577,
2.37983677511548,2.44191320609392,2.50575994370993,2.5668051915514,2.62957581345711,
2.69340170507181,2.75467017069393,2.81832480001291,2.88099397655741,2.94301771886783,
3.00749040232631,3.03058177228639),.UNSPECIFIED.);
#380=B_SPLINE_CURVE_WITH_KNOTS('',3,(#34642,#34643,#34644,#34645,#34646,
#34647,#34648,#34649,#34650,#34651,#34652,#34653,#34654,#34655,#34656,#34657,
#34658,#34659,#34660,#34661,#34662,#34663,#34664,#34665,#34666,#34667,#34668,
#34669,#34670,#34671,#34672,#34673,#34674,#34675,#34676,#34677),
 .UNSPECIFIED.,.F.,.F.,(4,2,2,2,2,2,2,2,2,2,2,2,2,2,2,2,2,4),(11.1275070958942,
11.1704537304032,11.2342688483924,11.2956910839699,11.3596585420614,11.4225901153166,
11.4837561576735,11.5477438342631,11.6099809376208,11.6721838169566,11.7360824974812,
11.7975793132747,11.862033730474,11.9250424842215,11.9860793785899,12.0499980505855,
12.1123215932317,12.1402573446881),.UNSPECIFIED.);
#381=B_SPLINE_CURVE_WITH_KNOTS('',3,(#34678,#34679,#34680,#34681,#34682,
#34683,#34684,#34685,#34686,#34687,#34688,#34689,#34690,#34691,#34692,#34693,
#34694,#34695,#34696,#34697,#34698,#34699,#34700,#34701,#34702,#34703,#34704,
#34705,#34706,#34707,#34708,#34709,#34710,#34711,#34712,#34713),
 .UNSPECIFIED.,.F.,.F.,(4,2,2,2,2,2,2,2,2,2,2,2,2,2,2,2,2,4),(1.01041293968269,
1.06459532413738,1.12773186594428,1.1909758101729,1.25253688832545,1.31651426807939,
1.37796756271407,1.4402543169856,1.50399348106341,1.56484253694405,1.62780397062662,
1.69159377589592,1.75301550684636,1.81684104028362,1.87858830448784,1.94074155682194,
2.00451236612964,2.01959218604488),.UNSPECIFIED.);
#382=B_SPLINE_CURVE_WITH_KNOTS('',3,(#34720,#34721,#34722,#34723,#34724,
#34725,#34726,#34727),.UNSPECIFIED.,.F.,.F.,(4,2,2,4),(13.151979181519,
13.1772505756377,13.2268757105544,13.2769541484665),.UNSPECIFIED.);
#383=B_SPLINE_CURVE_WITH_KNOTS('',3,(#35563,#35564,#35565,#35566,#35567,
#35568,#35569,#35570,#35571,#35572,#35573,#35574,#35575,#35576,#35577,#35578,
#35579,#35580,#35581,#35582,#35583,#35584,#35585,#35586,#35587,#35588,#35589,
#35590,#35591,#35592,#35593,#35594,#35595,#35596,#35597,#35598),
 .UNSPECIFIED.,.F.,.F.,(4,2,2,2,2,2,2,2,2,2,2,2,2,2,2,2,2,4),(12.1402573446881,
12.1741660806478,12.2381689628595,12.2997603383981,12.3636114787066,12.4267523742039,
12.4877509879086,12.5516454501077,12.6141119167696,12.6756763354339,12.7398406522336,
12.8015803756614,12.8648977514758,12.9282223899383,12.9892859123381,13.0532037605178,
13.1158669759719,13.151979181519),.UNSPECIFIED.);
#384=B_SPLINE_CURVE_WITH_KNOTS('',3,(#35952,#35953,#35954,#35955,#35956,
#35957,#35958,#35959,#35960,#35961,#35962,#35963,#35964,#35965,#35966,#35967,
#35968,#35969,#35970,#35971,#35972,#35973,#35974,#35975,#35976,#35977,#35978,
#35979,#35980,#35981,#35982,#35983,#35984,#35985,#35986,#35987),
 .UNSPECIFIED.,.F.,.F.,(4,2,2,2,2,2,2,2,2,2,2,2,2,2,2,2,2,4),(0.,0.062854565099621,
0.126484087138076,0.188938677080355,0.250931183419829,0.315374552221337,
0.376541583571281,0.439254841233545,0.503075030045385,0.564126285197331,
0.62748646183889,0.690277756336167,0.752029883476157,0.8162141093586,0.877470009247812,
0.939944443819231,1.00369893667666,1.01041293968269),.UNSPECIFIED.);
#415=(
BOUNDED_SURFACE()
B_SPLINE_SURFACE(1,2,((#35210,#35211,#35212,#35213,#35214,#35215,#35216,
#35217,#35218,#35219,#35220,#35221,#35222,#35223,#35224,#35225,#35226,#35227,
#35228,#35229,#35230,#35231,#35232,#35233,#35234,#35235,#35236,#35237,#35238,
#35239,#35240,#35241,#35242,#35243,#35244,#35245,#35246,#35247,#35248,#35249,
#35250,#35251,#35252,#35253,#35254,#35255,#35256,#35257,#35258,#35259,#35260,
#35261,#35262,#35263,#35264,#35265,#35266,#35267,#35268,#35269,#35270,#35271,
#35272,#35273,#35274,#35275,#35276,#35277,#35278,#35279,#35280,#35281,#35282,
#35283,#35284,#35285,#35286,#35287,#35288,#35289,#35290,#35291,#35292,#35293,
#35294,#35295,#35296,#35297,#35298,#35299,#35300,#35301,#35302,#35303,#35304,
#35305,#35306,#35307,#35308,#35309,#35310,#35311,#35312,#35313,#35314,#35315,
#35316,#35317,#35318,#35319,#35320,#35321,#35322,#35323,#35324,#35325,#35326,
#35327,#35328,#35329,#35330,#35331,#35332,#35333,#35334,#35335,#35336,#35337,
#35338,#35339,#35340,#35341,#35342,#35343,#35344,#35345,#35346,#35347,#35348,
#35349,#35350,#35351,#35352,#35353,#35354,#35355,#35356,#35357,#35358,#35359,
#35360,#35361,#35362,#35363,#35364,#35365,#35366,#35367,#35368,#35369,#35370,
#35371,#35372,#35373,#35374,#35375,#35376,#35377,#35378),(#35379,#35380,
#35381,#35382,#35383,#35384,#35385,#35386,#35387,#35388,#35389,#35390,#35391,
#35392,#35393,#35394,#35395,#35396,#35397,#35398,#35399,#35400,#35401,#35402,
#35403,#35404,#35405,#35406,#35407,#35408,#35409,#35410,#35411,#35412,#35413,
#35414,#35415,#35416,#35417,#35418,#35419,#35420,#35421,#35422,#35423,#35424,
#35425,#35426,#35427,#35428,#35429,#35430,#35431,#35432,#35433,#35434,#35435,
#35436,#35437,#35438,#35439,#35440,#35441,#35442,#35443,#35444,#35445,#35446,
#35447,#35448,#35449,#35450,#35451,#35452,#35453,#35454,#35455,#35456,#35457,
#35458,#35459,#35460,#35461,#35462,#35463,#35464,#35465,#35466,#35467,#35468,
#35469,#35470,#35471,#35472,#35473,#35474,#35475,#35476,#35477,#35478,#35479,
#35480,#35481,#35482,#35483,#35484,#35485,#35486,#35487,#35488,#35489,#35490,
#35491,#35492,#35493,#35494,#35495,#35496,#35497,#35498,#35499,#35500,#35501,
#35502,#35503,#35504,#35505,#35506,#35507,#35508,#35509,#35510,#35511,#35512,
#35513,#35514,#35515,#35516,#35517,#35518,#35519,#35520,#35521,#35522,#35523,
#35524,#35525,#35526,#35527,#35528,#35529,#35530,#35531,#35532,#35533,#35534,
#35535,#35536,#35537,#35538,#35539,#35540,#35541,#35542,#35543,#35544,#35545,
#35546,#35547)),.UNSPECIFIED.,.F.,.F.,.F.)
B_SPLINE_SURFACE_WITH_KNOTS((2,2),(3,2,2,2,2,2,2,2,2,2,2,2,2,2,2,2,2,2,
2,2,2,2,2,2,2,2,2,2,2,2,2,2,2,2,2,2,2,2,2,2,2,2,2,2,2,2,2,2,2,2,2,2,2,2,
2,2,2,2,2,2,2,2,2,2,2,2,2,2,2,2,2,2,2,2,2,2,2,2,2,2,2,2,2,2,3),(0.,1.),
(0.,0.0119047619047619,0.0238095238095238,0.0357142857142857,0.0476190476190476,
0.0595238095238095,0.0714285714285714,0.0833333333333333,0.0952380952380952,
0.107142857142857,0.119047619047619,0.130952380952381,0.142857142857143,
0.154761904761905,0.166666666666667,0.178571428571428,0.19047619047619,
0.202380952380952,0.214285714285714,0.226190476190476,0.238095238095238,
0.25,0.261904761904762,0.273809523809524,0.285714285714286,0.297619047619048,
0.309523809523809,0.321428571428572,0.333333333333334,0.345238095238096,
0.357142857142857,0.369047619047619,0.380952380952381,0.392857142857143,
0.404761904761905,0.416666666666667,0.428571428571428,0.44047619047619,
0.452380952380952,0.464285714285714,0.476190476190476,0.488095238095238,
0.5,0.511904761904762,0.523809523809524,0.535714285714286,0.547619047619048,
0.55952380952381,0.571428571428571,0.583333333333333,0.595238095238095,
0.607142857142857,0.619047619047619,0.630952380952381,0.642857142857143,
0.654761904761905,0.666666666666667,0.678571428571429,0.690476190476191,
0.702380952380952,0.714285714285714,0.726190476190476,0.738095238095238,
0.75,0.761904761904762,0.773809523809524,0.785714285714286,0.797619047619048,
0.809523809523809,0.821428571428572,0.833333333333333,0.845238095238095,
0.857142857142857,0.869047619047619,0.880952380952381,0.892857142857143,
0.904761904761905,0.916666666666667,0.928571428571429,0.94047619047619,
0.952380952380952,0.964285714285714,0.976190476190476,0.988095238095238,
1.),.UNSPECIFIED.)
GEOMETRIC_REPRESENTATION_ITEM()
RATIONAL_B_SPLINE_SURFACE(((1.,0.866025403784439,1.,0.866025403784439,1.,
0.866025403784439,1.,0.866025403784439,1.,0.866025403784439,1.,0.866025403784439,
1.,0.866025403784439,1.,0.866025403784439,1.,0.866025403784439,1.,0.866025403784439,
1.,0.866025403784439,1.,0.866025403784439,1.,0.866025403784439,1.,0.866025403784439,
1.,0.866025403784439,1.,0.866025403784439,1.,0.866025403784439,1.,0.866025403784439,
1.,0.866025403784439,1.,0.866025403784439,1.,0.866025403784439,1.,0.866025403784439,
1.,0.866025403784439,1.,0.866025403784439,1.,0.866025403784439,1.,0.866025403784439,
1.,0.866025403784439,1.,0.866025403784439,1.,0.866025403784439,1.,0.866025403784439,
1.,0.866025403784439,1.,0.866025403784439,1.,0.866025403784439,1.,0.866025403784439,
1.,0.866025403784439,1.,0.866025403784439,1.,0.866025403784439,1.,0.866025403784439,
1.,0.866025403784439,1.,0.866025403784439,1.,0.866025403784439,1.,0.866025403784439,
1.,0.866025403784439,1.,0.866025403784439,1.,0.866025403784439,1.,0.866025403784439,
1.,0.866025403784439,1.,0.866025403784439,1.,0.866025403784439,1.,0.866025403784439,
1.,0.866025403784439,1.,0.866025403784439,1.,0.866025403784439,1.,0.866025403784439,
1.,0.866025403784439,1.,0.866025403784439,1.,0.866025403784439,1.,0.866025403784439,
1.,0.866025403784439,1.,0.866025403784439,1.,0.866025403784439,1.,0.866025403784439,
1.,0.866025403784439,1.,0.866025403784439,1.,0.866025403784439,1.,0.866025403784439,
1.,0.866025403784439,1.,0.866025403784439,1.,0.866025403784439,1.,0.866025403784439,
1.,0.866025403784439,1.,0.866025403784439,1.,0.866025403784439,1.,0.866025403784439,
1.,0.866025403784439,1.,0.866025403784439,1.,0.866025403784439,1.,0.866025403784439,
1.,0.866025403784439,1.,0.866025403784439,1.,0.866025403784439,1.,0.866025403784439,
1.,0.866025403784439,1.,0.866025403784439,1.),(1.,0.866025403784439,1.,
0.866025403784439,1.,0.866025403784439,1.,0.866025403784439,1.,0.866025403784439,
1.,0.866025403784439,1.,0.866025403784439,1.,0.866025403784439,1.,0.866025403784439,
1.,0.866025403784439,1.,0.866025403784439,1.,0.866025403784439,1.,0.866025403784439,
1.,0.866025403784439,1.,0.866025403784439,1.,0.866025403784439,1.,0.866025403784439,
1.,0.866025403784439,1.,0.866025403784439,1.,0.866025403784439,1.,0.866025403784439,
1.,0.866025403784439,1.,0.866025403784439,1.,0.866025403784439,1.,0.866025403784439,
1.,0.866025403784439,1.,0.866025403784439,1.,0.866025403784439,1.,0.866025403784439,
1.,0.866025403784439,1.,0.866025403784439,1.,0.866025403784439,1.,0.866025403784439,
1.,0.866025403784439,1.,0.866025403784439,1.,0.866025403784439,1.,0.866025403784439,
1.,0.866025403784439,1.,0.866025403784439,1.,0.866025403784439,1.,0.866025403784439,
1.,0.866025403784439,1.,0.866025403784439,1.,0.866025403784439,1.,0.866025403784439,
1.,0.866025403784439,1.,0.866025403784439,1.,0.866025403784439,1.,0.866025403784439,
1.,0.866025403784439,1.,0.866025403784439,1.,0.866025403784439,1.,0.866025403784439,
1.,0.866025403784439,1.,0.866025403784439,1.,0.866025403784439,1.,0.866025403784439,
1.,0.866025403784439,1.,0.866025403784439,1.,0.866025403784439,1.,0.866025403784439,
1.,0.866025403784439,1.,0.866025403784439,1.,0.866025403784439,1.,0.866025403784439,
1.,0.866025403784439,1.,0.866025403784439,1.,0.866025403784439,1.,0.866025403784439,
1.,0.866025403784439,1.,0.866025403784439,1.,0.866025403784439,1.,0.866025403784439,
1.,0.866025403784439,1.,0.866025403784439,1.,0.866025403784439,1.,0.866025403784439,
1.,0.866025403784439,1.,0.866025403784439,1.,0.866025403784439,1.,0.866025403784439,
1.,0.866025403784439,1.,0.866025403784439,1.,0.866025403784439,1.)))
REPRESENTATION_ITEM('')
SURFACE()
);
#416=(
BOUNDED_SURFACE()
B_SPLINE_SURFACE(1,2,((#35613,#35614,#35615,#35616,#35617,#35618,#35619,
#35620,#35621,#35622,#35623,#35624,#35625,#35626,#35627,#35628,#35629,#35630,
#35631,#35632,#35633,#35634,#35635,#35636,#35637,#35638,#35639,#35640,#35641,
#35642,#35643,#35644,#35645,#35646,#35647,#35648,#35649,#35650,#35651,#35652,
#35653,#35654,#35655,#35656,#35657,#35658,#35659,#35660,#35661,#35662,#35663,
#35664,#35665,#35666,#35667,#35668,#35669,#35670,#35671,#35672,#35673,#35674,
#35675,#35676,#35677,#35678,#35679,#35680,#35681,#35682,#35683,#35684,#35685,
#35686,#35687,#35688,#35689,#35690,#35691,#35692,#35693,#35694,#35695,#35696,
#35697,#35698,#35699,#35700,#35701,#35702,#35703,#35704,#35705,#35706,#35707,
#35708,#35709,#35710,#35711,#35712,#35713,#35714,#35715,#35716,#35717,#35718,
#35719,#35720,#35721,#35722,#35723,#35724,#35725,#35726,#35727,#35728,#35729,
#35730,#35731,#35732,#35733,#35734,#35735,#35736,#35737,#35738,#35739,#35740,
#35741,#35742,#35743,#35744,#35745,#35746,#35747,#35748,#35749,#35750,#35751,
#35752,#35753,#35754,#35755,#35756,#35757,#35758,#35759,#35760,#35761,#35762,
#35763,#35764,#35765,#35766,#35767,#35768,#35769,#35770,#35771,#35772,#35773,
#35774,#35775,#35776,#35777,#35778,#35779,#35780,#35781),(#35782,#35783,
#35784,#35785,#35786,#35787,#35788,#35789,#35790,#35791,#35792,#35793,#35794,
#35795,#35796,#35797,#35798,#35799,#35800,#35801,#35802,#35803,#35804,#35805,
#35806,#35807,#35808,#35809,#35810,#35811,#35812,#35813,#35814,#35815,#35816,
#35817,#35818,#35819,#35820,#35821,#35822,#35823,#35824,#35825,#35826,#35827,
#35828,#35829,#35830,#35831,#35832,#35833,#35834,#35835,#35836,#35837,#35838,
#35839,#35840,#35841,#35842,#35843,#35844,#35845,#35846,#35847,#35848,#35849,
#35850,#35851,#35852,#35853,#35854,#35855,#35856,#35857,#35858,#35859,#35860,
#35861,#35862,#35863,#35864,#35865,#35866,#35867,#35868,#35869,#35870,#35871,
#35872,#35873,#35874,#35875,#35876,#35877,#35878,#35879,#35880,#35881,#35882,
#35883,#35884,#35885,#35886,#35887,#35888,#35889,#35890,#35891,#35892,#35893,
#35894,#35895,#35896,#35897,#35898,#35899,#35900,#35901,#35902,#35903,#35904,
#35905,#35906,#35907,#35908,#35909,#35910,#35911,#35912,#35913,#35914,#35915,
#35916,#35917,#35918,#35919,#35920,#35921,#35922,#35923,#35924,#35925,#35926,
#35927,#35928,#35929,#35930,#35931,#35932,#35933,#35934,#35935,#35936,#35937,
#35938,#35939,#35940,#35941,#35942,#35943,#35944,#35945,#35946,#35947,#35948,
#35949,#35950)),.UNSPECIFIED.,.F.,.F.,.F.)
B_SPLINE_SURFACE_WITH_KNOTS((2,2),(3,2,2,2,2,2,2,2,2,2,2,2,2,2,2,2,2,2,
2,2,2,2,2,2,2,2,2,2,2,2,2,2,2,2,2,2,2,2,2,2,2,2,2,2,2,2,2,2,2,2,2,2,2,2,
2,2,2,2,2,2,2,2,2,2,2,2,2,2,2,2,2,2,2,2,2,2,2,2,2,2,2,2,2,2,3),(0.,1.),
(0.,0.0119047619047619,0.0238095238095238,0.0357142857142857,0.0476190476190476,
0.0595238095238095,0.0714285714285714,0.0833333333333333,0.0952380952380952,
0.107142857142857,0.119047619047619,0.130952380952381,0.142857142857143,
0.154761904761905,0.166666666666667,0.178571428571428,0.19047619047619,
0.202380952380952,0.214285714285714,0.226190476190476,0.238095238095238,
0.25,0.261904761904762,0.273809523809524,0.285714285714286,0.297619047619048,
0.309523809523809,0.321428571428572,0.333333333333334,0.345238095238096,
0.357142857142857,0.369047619047619,0.380952380952381,0.392857142857143,
0.404761904761905,0.416666666666667,0.428571428571428,0.44047619047619,
0.452380952380952,0.464285714285714,0.476190476190476,0.488095238095238,
0.5,0.511904761904762,0.523809523809524,0.535714285714286,0.547619047619048,
0.55952380952381,0.571428571428571,0.583333333333333,0.595238095238095,
0.607142857142857,0.619047619047619,0.630952380952381,0.642857142857143,
0.654761904761905,0.666666666666667,0.678571428571429,0.690476190476191,
0.702380952380952,0.714285714285714,0.726190476190476,0.738095238095238,
0.75,0.761904761904762,0.773809523809524,0.785714285714286,0.797619047619048,
0.809523809523809,0.821428571428572,0.833333333333333,0.845238095238095,
0.857142857142857,0.869047619047619,0.880952380952381,0.892857142857143,
0.904761904761905,0.916666666666667,0.928571428571429,0.94047619047619,
0.952380952380952,0.964285714285714,0.976190476190476,0.988095238095238,
1.),.UNSPECIFIED.)
GEOMETRIC_REPRESENTATION_ITEM()
RATIONAL_B_SPLINE_SURFACE(((1.,0.866025403784439,1.,0.866025403784439,1.,
0.866025403784439,1.,0.866025403784439,1.,0.866025403784439,1.,0.866025403784439,
1.,0.866025403784439,1.,0.866025403784439,1.,0.866025403784439,1.,0.866025403784439,
1.,0.866025403784439,1.,0.866025403784439,1.,0.866025403784439,1.,0.866025403784439,
1.,0.866025403784439,1.,0.866025403784439,1.,0.866025403784439,1.,0.866025403784439,
1.,0.866025403784439,1.,0.866025403784439,1.,0.866025403784439,1.,0.866025403784439,
1.,0.866025403784439,1.,0.866025403784439,1.,0.866025403784439,1.,0.866025403784439,
1.,0.866025403784439,1.,0.866025403784439,1.,0.866025403784439,1.,0.866025403784439,
1.,0.866025403784439,1.,0.866025403784439,1.,0.866025403784439,1.,0.866025403784439,
1.,0.866025403784439,1.,0.866025403784439,1.,0.866025403784439,1.,0.866025403784439,
1.,0.866025403784439,1.,0.866025403784439,1.,0.866025403784439,1.,0.866025403784439,
1.,0.866025403784439,1.,0.866025403784439,1.,0.866025403784439,1.,0.866025403784439,
1.,0.866025403784439,1.,0.866025403784439,1.,0.866025403784439,1.,0.866025403784439,
1.,0.866025403784439,1.,0.866025403784439,1.,0.866025403784439,1.,0.866025403784439,
1.,0.866025403784439,1.,0.866025403784439,1.,0.866025403784439,1.,0.866025403784439,
1.,0.866025403784439,1.,0.866025403784439,1.,0.866025403784439,1.,0.866025403784439,
1.,0.866025403784439,1.,0.866025403784439,1.,0.866025403784439,1.,0.866025403784439,
1.,0.866025403784439,1.,0.866025403784439,1.,0.866025403784439,1.,0.866025403784439,
1.,0.866025403784439,1.,0.866025403784439,1.,0.866025403784439,1.,0.866025403784439,
1.,0.866025403784439,1.,0.866025403784439,1.,0.866025403784439,1.,0.866025403784439,
1.,0.866025403784439,1.,0.866025403784439,1.,0.866025403784439,1.,0.866025403784439,
1.,0.866025403784439,1.,0.866025403784439,1.),(1.,0.866025403784439,1.,
0.866025403784439,1.,0.866025403784439,1.,0.866025403784439,1.,0.866025403784439,
1.,0.866025403784439,1.,0.866025403784439,1.,0.866025403784439,1.,0.866025403784439,
1.,0.866025403784439,1.,0.866025403784439,1.,0.866025403784439,1.,0.866025403784439,
1.,0.866025403784439,1.,0.866025403784439,1.,0.866025403784439,1.,0.866025403784439,
1.,0.866025403784439,1.,0.866025403784439,1.,0.866025403784439,1.,0.866025403784439,
1.,0.866025403784439,1.,0.866025403784439,1.,0.866025403784439,1.,0.866025403784439,
1.,0.866025403784439,1.,0.866025403784439,1.,0.866025403784439,1.,0.866025403784439,
1.,0.866025403784439,1.,0.866025403784439,1.,0.866025403784439,1.,0.866025403784439,
1.,0.866025403784439,1.,0.866025403784439,1.,0.866025403784439,1.,0.866025403784439,
1.,0.866025403784439,1.,0.866025403784439,1.,0.866025403784439,1.,0.866025403784439,
1.,0.866025403784439,1.,0.866025403784439,1.,0.866025403784439,1.,0.866025403784439,
1.,0.866025403784439,1.,0.866025403784439,1.,0.866025403784439,1.,0.866025403784439,
1.,0.866025403784439,1.,0.866025403784439,1.,0.866025403784439,1.,0.866025403784439,
1.,0.866025403784439,1.,0.866025403784439,1.,0.866025403784439,1.,0.866025403784439,
1.,0.866025403784439,1.,0.866025403784439,1.,0.866025403784439,1.,0.866025403784439,
1.,0.866025403784439,1.,0.866025403784439,1.,0.866025403784439,1.,0.866025403784439,
1.,0.866025403784439,1.,0.866025403784439,1.,0.866025403784439,1.,0.866025403784439,
1.,0.866025403784439,1.,0.866025403784439,1.,0.866025403784439,1.,0.866025403784439,
1.,0.866025403784439,1.,0.866025403784439,1.,0.866025403784439,1.,0.866025403784439,
1.,0.866025403784439,1.,0.866025403784439,1.,0.866025403784439,1.,0.866025403784439,
1.,0.866025403784439,1.,0.866025403784439,1.,0.866025403784439,1.)))
REPRESENTATION_ITEM('')
SURFACE()
);
#432=ELLIPSE('',#19299,0.715693849834519,0.699999999997075);
#433=ELLIPSE('',#19300,0.715693849836967,0.699999999999567);
#434=ELLIPSE('',#19301,0.720792014405194,0.700000000003498);
#435=ELLIPSE('',#19302,0.720792014401284,0.699999999999729);
#436=ELLIPSE('',#19304,0.704512458806093,0.699999999997662);
#437=ELLIPSE('',#19305,0.70237579871988,0.699999999997508);
#438=ELLIPSE('',#19306,0.702375798725131,0.700000000002555);
#439=ELLIPSE('',#19307,0.704512458813107,0.700000000004563);
#440=ELLIPSE('',#19309,0.624754966914843,0.599999999999018);
#441=ELLIPSE('',#19310,0.624754966916465,0.600000000000533);
#442=ELLIPSE('',#19311,0.624754966913492,0.599999999997754);
#443=ELLIPSE('',#19312,0.624754966919923,0.600000000003613);
#444=ELLIPSE('',#19339,0.577350269188758,0.49999999999938);
#445=ELLIPSE('',#19340,0.577350269187932,0.499999999998527);
#446=ELLIPSE('',#19342,0.577350269187005,0.499999999997962);
#447=ELLIPSE('',#19344,0.577350269188423,0.499999999999111);
#448=ELLIPSE('',#19346,0.577350269189091,0.499999999999555);
#449=ELLIPSE('',#19348,0.577350269191436,0.500000000001306);
#458=SHAPE_REPRESENTATION_RELATIONSHIP('SRR','None',#36714,#468);
#468=ADVANCED_BREP_SHAPE_REPRESENTATION('',(#52),#36666);
#478=STYLED_ITEM('',(#36770),#52);
#710=CYLINDRICAL_SURFACE('',#19175,4.);
#711=CYLINDRICAL_SURFACE('',#19176,1.6);
#712=CYLINDRICAL_SURFACE('',#19178,1.6);
#713=CYLINDRICAL_SURFACE('',#19179,1.6);
#714=CYLINDRICAL_SURFACE('',#19180,1.6);
#715=CYLINDRICAL_SURFACE('',#19181,1.6);
#716=CYLINDRICAL_SURFACE('',#19182,1.6);
#717=CYLINDRICAL_SURFACE('',#19183,1.6);
#718=CYLINDRICAL_SURFACE('',#19184,1.6);
#719=CYLINDRICAL_SURFACE('',#19185,1.6);
#720=CYLINDRICAL_SURFACE('',#19186,1.6);
#721=CYLINDRICAL_SURFACE('',#19187,1.6);
#722=CYLINDRICAL_SURFACE('',#19188,1.6);
#723=CYLINDRICAL_SURFACE('',#19189,1.6);
#724=CYLINDRICAL_SURFACE('',#19190,1.6);
#725=CYLINDRICAL_SURFACE('',#19192,1.22111388750008);
#726=CYLINDRICAL_SURFACE('',#19193,1.22111388750008);
#727=CYLINDRICAL_SURFACE('',#19194,1.22111388750008);
#728=CYLINDRICAL_SURFACE('',#19195,1.22111388750008);
#729=CYLINDRICAL_SURFACE('',#19196,1.22111388750008);
#730=CYLINDRICAL_SURFACE('',#19197,1.22111388750008);
#731=CYLINDRICAL_SURFACE('',#19198,1.22111388750008);
#732=CYLINDRICAL_SURFACE('',#19199,1.22111388750008);
#733=CYLINDRICAL_SURFACE('',#19200,1.22111388750008);
#734=CYLINDRICAL_SURFACE('',#19201,1.22111388750008);
#735=CYLINDRICAL_SURFACE('',#19202,1.22111388750008);
#736=CYLINDRICAL_SURFACE('',#19203,1.22111388750008);
#737=CYLINDRICAL_SURFACE('',#19204,1.22111388750008);
#738=CYLINDRICAL_SURFACE('',#19205,1.22111388750008);
#739=CYLINDRICAL_SURFACE('',#19206,1.60000000000001);
#740=CYLINDRICAL_SURFACE('',#19209,1.49172584788676);
#741=CYLINDRICAL_SURFACE('',#19212,1.04190416256385);
#742=CYLINDRICAL_SURFACE('',#19235,3.25);
#743=CYLINDRICAL_SURFACE('',#19236,12.);
#744=CYLINDRICAL_SURFACE('',#19242,1.59999999999981);
#745=CYLINDRICAL_SURFACE('',#19245,1.22111388750008);
#746=CYLINDRICAL_SURFACE('',#19248,1.59999999999981);
#747=CYLINDRICAL_SURFACE('',#19258,1.6);
#748=CYLINDRICAL_SURFACE('',#19268,5.);
#749=CYLINDRICAL_SURFACE('',#19269,7.);
#750=CYLINDRICAL_SURFACE('',#19271,4.22087352428905);
#751=CYLINDRICAL_SURFACE('',#19274,1.6);
#752=CYLINDRICAL_SURFACE('',#19279,4.5);
#753=CYLINDRICAL_SURFACE('',#19294,5.14310210370206);
#754=CYLINDRICAL_SURFACE('',#19317,0.699999999999999);
#755=CYLINDRICAL_SURFACE('',#19318,0.699999999999999);
#756=CYLINDRICAL_SURFACE('',#19319,0.7);
#757=CYLINDRICAL_SURFACE('',#19320,0.7);
#758=CYLINDRICAL_SURFACE('',#19325,0.599999999999998);
#759=CYLINDRICAL_SURFACE('',#19326,0.599999999999998);
#760=CYLINDRICAL_SURFACE('',#19327,0.599999999999998);
#761=CYLINDRICAL_SURFACE('',#19328,0.599999999999998);
#762=CYLINDRICAL_SURFACE('',#19338,0.499999999999999);
#763=CYLINDRICAL_SURFACE('',#19341,0.500000000000004);
#764=CYLINDRICAL_SURFACE('',#19343,0.500000000000005);
#765=CYLINDRICAL_SURFACE('',#19345,0.500000000000005);
#766=CYLINDRICAL_SURFACE('',#19347,0.500000000000004);
#767=CYLINDRICAL_SURFACE('',#19349,0.499999999999999);
#768=CYLINDRICAL_SURFACE('',#19350,4.);
#769=CYLINDRICAL_SURFACE('',#19353,1.6);
#770=CYLINDRICAL_SURFACE('',#19356,4.50000000000007);
#771=CYLINDRICAL_SURFACE('',#19397,4.11168229960152);
#956=FACE_BOUND('',#3399,.T.);
#957=FACE_BOUND('',#3440,.T.);
#958=FACE_BOUND('',#3442,.T.);
#959=FACE_BOUND('',#3444,.T.);
#960=FACE_BOUND('',#3456,.T.);
#961=FACE_BOUND('',#3466,.T.);
#962=FACE_BOUND('',#3467,.T.);
#963=FACE_BOUND('',#3470,.T.);
#964=FACE_BOUND('',#3471,.T.);
#965=FACE_BOUND('',#3488,.T.);
#966=FACE_BOUND('',#3497,.T.);
#967=FACE_BOUND('',#3503,.T.);
#968=FACE_BOUND('',#3520,.T.);
#969=FACE_BOUND('',#3566,.T.);
#970=FACE_BOUND('',#3568,.T.);
#1456=CIRCLE('',#19170,4.);
#1457=CIRCLE('',#19171,3.6);
#1458=CIRCLE('',#19173,4.);
#1459=CIRCLE('',#19174,4.);
#1460=CIRCLE('',#19177,1.6);
#1461=CIRCLE('',#19191,1.6);
#1462=CIRCLE('',#19207,1.60000000000001);
#1463=CIRCLE('',#19208,1.6);
#1464=CIRCLE('',#19210,1.49172584788676);
#1465=CIRCLE('',#19211,1.49172584788676);
#1466=CIRCLE('',#19213,1.04190416256385);
#1467=CIRCLE('',#19214,1.04190416256385);
#1468=CIRCLE('',#19216,11.8);
#1469=CIRCLE('',#19217,0.2);
#1470=CIRCLE('',#19218,12.);
#1471=CIRCLE('',#19219,12.);
#1472=CIRCLE('',#19221,12.);
#1473=CIRCLE('',#19222,12.);
#1474=CIRCLE('',#19223,0.2);
#1475=CIRCLE('',#19224,11.8);
#1476=CIRCLE('',#19226,3.25);
#1477=CIRCLE('',#19227,3.25);
#1478=CIRCLE('',#19228,0.2);
#1479=CIRCLE('',#19229,3.45);
#1480=CIRCLE('',#19231,3.45);
#1481=CIRCLE('',#19232,0.2);
#1482=CIRCLE('',#19233,3.25);
#1483=CIRCLE('',#19234,3.25);
#1484=CIRCLE('',#19239,7.);
#1485=CIRCLE('',#19241,2.);
#1486=CIRCLE('',#19243,1.6);
#1487=CIRCLE('',#19244,1.6);
#1488=CIRCLE('',#19249,1.6);
#1489=CIRCLE('',#19251,2.);
#1490=CIRCLE('',#19254,4.);
#1491=CIRCLE('',#19255,4.);
#1492=CIRCLE('',#19256,3.6);
#1493=CIRCLE('',#19261,5.);
#1494=CIRCLE('',#19262,0.5);
#1495=CIRCLE('',#19263,4.5);
#1496=CIRCLE('',#19265,4.5);
#1497=CIRCLE('',#19266,0.5);
#1498=CIRCLE('',#19267,5.);
#1499=CIRCLE('',#19270,7.);
#1500=CIRCLE('',#19272,4.22087352428905);
#1501=CIRCLE('',#19273,4.22087352428905);
#1502=CIRCLE('',#19275,1.6);
#1503=CIRCLE('',#19276,1.6);
#1504=CIRCLE('',#19278,5.14310210370206);
#1505=CIRCLE('',#19280,4.5);
#1506=CIRCLE('',#19281,4.5);
#1507=CIRCLE('',#19283,5.14310210370206);
#1508=CIRCLE('',#19284,4.);
#1509=CIRCLE('',#19286,0.599999999999998);
#1510=CIRCLE('',#19287,0.599999999999998);
#1511=CIRCLE('',#19288,0.599999999999998);
#1512=CIRCLE('',#19289,0.599999999999998);
#1513=CIRCLE('',#19352,1.60000000000001);
#1514=CIRCLE('',#19354,1.6);
#1515=CIRCLE('',#19357,4.50000000000007);
#1516=CIRCLE('',#19358,4.50000000000007);
#1517=CIRCLE('',#19398,4.11168229960152);
#1518=CIRCLE('',#19399,4.11168229960152);
#2287=FACE_OUTER_BOUND('',#3398,.T.);
#2288=FACE_OUTER_BOUND('',#3400,.T.);
#2289=FACE_OUTER_BOUND('',#3401,.T.);
#2290=FACE_OUTER_BOUND('',#3402,.T.);
#2291=FACE_OUTER_BOUND('',#3403,.T.);
#2292=FACE_OUTER_BOUND('',#3404,.T.);
#2293=FACE_OUTER_BOUND('',#3405,.T.);
#2294=FACE_OUTER_BOUND('',#3406,.T.);
#2295=FACE_OUTER_BOUND('',#3407,.T.);
#2296=FACE_OUTER_BOUND('',#3408,.T.);
#2297=FACE_OUTER_BOUND('',#3409,.T.);
#2298=FACE_OUTER_BOUND('',#3410,.T.);
#2299=FACE_OUTER_BOUND('',#3411,.T.);
#2300=FACE_OUTER_BOUND('',#3412,.T.);
#2301=FACE_OUTER_BOUND('',#3413,.T.);
#2302=FACE_OUTER_BOUND('',#3414,.T.);
#2303=FACE_OUTER_BOUND('',#3415,.T.);
#2304=FACE_OUTER_BOUND('',#3416,.T.);
#2305=FACE_OUTER_BOUND('',#3417,.T.);
#2306=FACE_OUTER_BOUND('',#3418,.T.);
#2307=FACE_OUTER_BOUND('',#3419,.T.);
#2308=FACE_OUTER_BOUND('',#3420,.T.);
#2309=FACE_OUTER_BOUND('',#3421,.T.);
#2310=FACE_OUTER_BOUND('',#3422,.T.);
#2311=FACE_OUTER_BOUND('',#3423,.T.);
#2312=FACE_OUTER_BOUND('',#3424,.T.);
#2313=FACE_OUTER_BOUND('',#3425,.T.);
#2314=FACE_OUTER_BOUND('',#3426,.T.);
#2315=FACE_OUTER_BOUND('',#3427,.T.);
#2316=FACE_OUTER_BOUND('',#3428,.T.);
#2317=FACE_OUTER_BOUND('',#3429,.T.);
#2318=FACE_OUTER_BOUND('',#3430,.T.);
#2319=FACE_OUTER_BOUND('',#3431,.T.);
#2320=FACE_OUTER_BOUND('',#3432,.T.);
#2321=FACE_OUTER_BOUND('',#3433,.T.);
#2322=FACE_OUTER_BOUND('',#3434,.T.);
#2323=FACE_OUTER_BOUND('',#3435,.T.);
#2324=FACE_OUTER_BOUND('',#3436,.T.);
#2325=FACE_OUTER_BOUND('',#3437,.T.);
#2326=FACE_OUTER_BOUND('',#3438,.T.);
#2327=FACE_OUTER_BOUND('',#3439,.T.);
#2328=FACE_OUTER_BOUND('',#3441,.T.);
#2329=FACE_OUTER_BOUND('',#3443,.T.);
#2330=FACE_OUTER_BOUND('',#3445,.T.);
#2331=FACE_OUTER_BOUND('',#3446,.T.);
#2332=FACE_OUTER_BOUND('',#3447,.T.);
#2333=FACE_OUTER_BOUND('',#3448,.T.);
#2334=FACE_OUTER_BOUND('',#3449,.T.);
#2335=FACE_OUTER_BOUND('',#3450,.T.);
#2336=FACE_OUTER_BOUND('',#3451,.T.);
#2337=FACE_OUTER_BOUND('',#3452,.T.);
#2338=FACE_OUTER_BOUND('',#3453,.T.);
#2339=FACE_OUTER_BOUND('',#3454,.T.);
#2340=FACE_OUTER_BOUND('',#3455,.T.);
#2341=FACE_OUTER_BOUND('',#3457,.T.);
#2342=FACE_OUTER_BOUND('',#3458,.T.);
#2343=FACE_OUTER_BOUND('',#3459,.T.);
#2344=FACE_OUTER_BOUND('',#3460,.T.);
#2345=FACE_OUTER_BOUND('',#3461,.T.);
#2346=FACE_OUTER_BOUND('',#3462,.T.);
#2347=FACE_OUTER_BOUND('',#3463,.T.);
#2348=FACE_OUTER_BOUND('',#3464,.T.);
#2349=FACE_OUTER_BOUND('',#3465,.T.);
#2350=FACE_OUTER_BOUND('',#3468,.T.);
#2351=FACE_OUTER_BOUND('',#3469,.T.);
#2352=FACE_OUTER_BOUND('',#3472,.T.);
#2353=FACE_OUTER_BOUND('',#3473,.T.);
#2354=FACE_OUTER_BOUND('',#3474,.T.);
#2355=FACE_OUTER_BOUND('',#3475,.T.);
#2356=FACE_OUTER_BOUND('',#3476,.T.);
#2357=FACE_OUTER_BOUND('',#3477,.T.);
#2358=FACE_OUTER_BOUND('',#3478,.T.);
#2359=FACE_OUTER_BOUND('',#3479,.T.);
#2360=FACE_OUTER_BOUND('',#3480,.T.);
#2361=FACE_OUTER_BOUND('',#3481,.T.);
#2362=FACE_OUTER_BOUND('',#3482,.T.);
#2363=FACE_OUTER_BOUND('',#3483,.T.);
#2364=FACE_OUTER_BOUND('',#3484,.T.);
#2365=FACE_OUTER_BOUND('',#3485,.T.);
#2366=FACE_OUTER_BOUND('',#3486,.T.);
#2367=FACE_OUTER_BOUND('',#3487,.T.);
#2368=FACE_OUTER_BOUND('',#3489,.T.);
#2369=FACE_OUTER_BOUND('',#3490,.T.);
#2370=FACE_OUTER_BOUND('',#3491,.T.);
#2371=FACE_OUTER_BOUND('',#3492,.T.);
#2372=FACE_OUTER_BOUND('',#3493,.T.);
#2373=FACE_OUTER_BOUND('',#3494,.T.);
#2374=FACE_OUTER_BOUND('',#3495,.T.);
#2375=FACE_OUTER_BOUND('',#3496,.T.);
#2376=FACE_OUTER_BOUND('',#3498,.T.);
#2377=FACE_OUTER_BOUND('',#3499,.T.);
#2378=FACE_OUTER_BOUND('',#3500,.T.);
#2379=FACE_OUTER_BOUND('',#3501,.T.);
#2380=FACE_OUTER_BOUND('',#3502,.T.);
#2381=FACE_OUTER_BOUND('',#3504,.T.);
#2382=FACE_OUTER_BOUND('',#3505,.T.);
#2383=FACE_OUTER_BOUND('',#3506,.T.);
#2384=FACE_OUTER_BOUND('',#3507,.T.);
#2385=FACE_OUTER_BOUND('',#3508,.T.);
#2386=FACE_OUTER_BOUND('',#3509,.T.);
#2387=FACE_OUTER_BOUND('',#3510,.T.);
#2388=FACE_OUTER_BOUND('',#3511,.T.);
#2389=FACE_OUTER_BOUND('',#3512,.T.);
#2390=FACE_OUTER_BOUND('',#3513,.T.);
#2391=FACE_OUTER_BOUND('',#3514,.T.);
#2392=FACE_OUTER_BOUND('',#3515,.T.);
#2393=FACE_OUTER_BOUND('',#3516,.T.);
#2394=FACE_OUTER_BOUND('',#3517,.T.);
#2395=FACE_OUTER_BOUND('',#3518,.T.);
#2396=FACE_OUTER_BOUND('',#3519,.T.);
#2397=FACE_OUTER_BOUND('',#3521,.T.);
#2398=FACE_OUTER_BOUND('',#3522,.T.);
#2399=FACE_OUTER_BOUND('',#3523,.T.);
#2400=FACE_OUTER_BOUND('',#3524,.T.);
#2401=FACE_OUTER_BOUND('',#3525,.T.);
#2402=FACE_OUTER_BOUND('',#3526,.T.);
#2403=FACE_OUTER_BOUND('',#3527,.T.);
#2404=FACE_OUTER_BOUND('',#3528,.T.);
#2405=FACE_OUTER_BOUND('',#3529,.T.);
#2406=FACE_OUTER_BOUND('',#3530,.T.);
#2407=FACE_OUTER_BOUND('',#3531,.T.);
#2408=FACE_OUTER_BOUND('',#3532,.T.);
#2409=FACE_OUTER_BOUND('',#3533,.T.);
#2410=FACE_OUTER_BOUND('',#3534,.T.);
#2411=FACE_OUTER_BOUND('',#3535,.T.);
#2412=FACE_OUTER_BOUND('',#3536,.T.);
#2413=FACE_OUTER_BOUND('',#3537,.T.);
#2414=FACE_OUTER_BOUND('',#3538,.T.);
#2415=FACE_OUTER_BOUND('',#3539,.T.);
#2416=FACE_OUTER_BOUND('',#3540,.T.);
#2417=FACE_OUTER_BOUND('',#3541,.T.);
#2418=FACE_OUTER_BOUND('',#3542,.T.);
#2419=FACE_OUTER_BOUND('',#3543,.T.);
#2420=FACE_OUTER_BOUND('',#3544,.T.);
#2421=FACE_OUTER_BOUND('',#3545,.T.);
#2422=FACE_OUTER_BOUND('',#3546,.T.);
#2423=FACE_OUTER_BOUND('',#3547,.T.);
#2424=FACE_OUTER_BOUND('',#3548,.T.);
#2425=FACE_OUTER_BOUND('',#3549,.T.);
#2426=FACE_OUTER_BOUND('',#3550,.T.);
#2427=FACE_OUTER_BOUND('',#3551,.T.);
#2428=FACE_OUTER_BOUND('',#3552,.T.);
#2429=FACE_OUTER_BOUND('',#3553,.T.);
#2430=FACE_OUTER_BOUND('',#3554,.T.);
#2431=FACE_OUTER_BOUND('',#3555,.T.);
#2432=FACE_OUTER_BOUND('',#3556,.T.);
#2433=FACE_OUTER_BOUND('',#3557,.T.);
#2434=FACE_OUTER_BOUND('',#3558,.T.);
#2435=FACE_OUTER_BOUND('',#3559,.T.);
#2436=FACE_OUTER_BOUND('',#3560,.T.);
#2437=FACE_OUTER_BOUND('',#3561,.T.);
#2438=FACE_OUTER_BOUND('',#3562,.T.);
#2439=FACE_OUTER_BOUND('',#3563,.T.);
#2440=FACE_OUTER_BOUND('',#3564,.T.);
#2441=FACE_OUTER_BOUND('',#3565,.T.);
#2442=FACE_OUTER_BOUND('',#3567,.T.);
#2443=FACE_OUTER_BOUND('',#3569,.T.);
#3398=EDGE_LOOP('',(#15432));
#3399=EDGE_LOOP('',(#15433));
#3400=EDGE_LOOP('',(#15434,#15435,#15436,#15437,#15438));
#3401=EDGE_LOOP('',(#15439,#15440,#15441,#15442,#15443));
#3402=EDGE_LOOP('',(#15444,#15445,#15446,#15447));
#3403=EDGE_LOOP('',(#15448,#15449,#15450,#15451));
#3404=EDGE_LOOP('',(#15452,#15453,#15454,#15455));
#3405=EDGE_LOOP('',(#15456,#15457,#15458,#15459));
#3406=EDGE_LOOP('',(#15460,#15461,#15462,#15463));
#3407=EDGE_LOOP('',(#15464,#15465,#15466,#15467));
#3408=EDGE_LOOP('',(#15468,#15469,#15470,#15471));
#3409=EDGE_LOOP('',(#15472,#15473,#15474,#15475));
#3410=EDGE_LOOP('',(#15476,#15477,#15478,#15479));
#3411=EDGE_LOOP('',(#15480,#15481,#15482,#15483));
#3412=EDGE_LOOP('',(#15484,#15485,#15486,#15487));
#3413=EDGE_LOOP('',(#15488,#15489,#15490,#15491));
#3414=EDGE_LOOP('',(#15492,#15493,#15494,#15495));
#3415=EDGE_LOOP('',(#15496,#15497,#15498));
#3416=EDGE_LOOP('',(#15499,#15500,#15501,#15502));
#3417=EDGE_LOOP('',(#15503,#15504,#15505,#15506));
#3418=EDGE_LOOP('',(#15507,#15508,#15509,#15510));
#3419=EDGE_LOOP('',(#15511,#15512,#15513,#15514));
#3420=EDGE_LOOP('',(#15515,#15516,#15517,#15518));
#3421=EDGE_LOOP('',(#15519,#15520,#15521,#15522));
#3422=EDGE_LOOP('',(#15523,#15524,#15525,#15526));
#3423=EDGE_LOOP('',(#15527,#15528,#15529,#15530));
#3424=EDGE_LOOP('',(#15531,#15532,#15533,#15534));
#3425=EDGE_LOOP('',(#15535,#15536,#15537,#15538));
#3426=EDGE_LOOP('',(#15539,#15540,#15541,#15542));
#3427=EDGE_LOOP('',(#15543,#15544,#15545,#15546));
#3428=EDGE_LOOP('',(#15547,#15548,#15549,#15550));
#3429=EDGE_LOOP('',(#15551,#15552,#15553,#15554));
#3430=EDGE_LOOP('',(#15555,#15556,#15557,#15558));
#3431=EDGE_LOOP('',(#15559,#15560,#15561,#15562));
#3432=EDGE_LOOP('',(#15563,#15564,#15565,#15566));
#3433=EDGE_LOOP('',(#15567,#15568,#15569,#15570,#15571));
#3434=EDGE_LOOP('',(#15572,#15573,#15574,#15575,#15576));
#3435=EDGE_LOOP('',(#15577,#15578,#15579,#15580,#15581));
#3436=EDGE_LOOP('',(#15582,#15583,#15584,#15585,#15586));
#3437=EDGE_LOOP('',(#15587,#15588,#15589,#15590,#15591,#15592));
#3438=EDGE_LOOP('',(#15593,#15594,#15595,#15596,#15597,#15598));
#3439=EDGE_LOOP('',(#15599));
#3440=EDGE_LOOP('',(#15600));
#3441=EDGE_LOOP('',(#15601));
#3442=EDGE_LOOP('',(#15602));
#3443=EDGE_LOOP('',(#15603));
#3444=EDGE_LOOP('',(#15604));
#3445=EDGE_LOOP('',(#15605,#15606,#15607,#15608));
#3446=EDGE_LOOP('',(#15609,#15610,#15611,#15612,#15613,#15614,#15615,#15616,
#15617,#15618,#15619,#15620,#15621,#15622,#15623,#15624,#15625,#15626,#15627,
#15628,#15629,#15630,#15631,#15632,#15633,#15634,#15635,#15636,#15637,#15638,
#15639,#15640));
#3447=EDGE_LOOP('',(#15641,#15642,#15643,#15644));
#3448=EDGE_LOOP('',(#15645,#15646,#15647,#15648,#15649,#15650,#15651,#15652,
#15653,#15654,#15655,#15656,#15657,#15658,#15659,#15660,#15661,#15662,#15663,
#15664,#15665,#15666,#15667,#15668,#15669,#15670,#15671,#15672,#15673,#15674,
#15675,#15676));
#3449=EDGE_LOOP('',(#15677,#15678,#15679,#15680,#15681));
#3450=EDGE_LOOP('',(#15682,#15683,#15684,#15685));
#3451=EDGE_LOOP('',(#15686,#15687,#15688));
#3452=EDGE_LOOP('',(#15689,#15690,#15691,#15692,#15693,#15694));
#3453=EDGE_LOOP('',(#15695,#15696,#15697,#15698,#15699));
#3454=EDGE_LOOP('',(#15700,#15701,#15702,#15703,#15704));
#3455=EDGE_LOOP('',(#15705));
#3456=EDGE_LOOP('',(#15706));
#3457=EDGE_LOOP('',(#15707,#15708,#15709,#15710));
#3458=EDGE_LOOP('',(#15711));
#3459=EDGE_LOOP('',(#15712,#15713,#15714,#15715));
#3460=EDGE_LOOP('',(#15716,#15717,#15718,#15719));
#3461=EDGE_LOOP('',(#15720,#15721,#15722,#15723));
#3462=EDGE_LOOP('',(#15724,#15725,#15726,#15727));
#3463=EDGE_LOOP('',(#15728,#15729,#15730,#15731));
#3464=EDGE_LOOP('',(#15732,#15733,#15734,#15735));
#3465=EDGE_LOOP('',(#15736,#15737,#15738,#15739,#15740,#15741,#15742,#15743,
#15744,#15745,#15746,#15747,#15748,#15749));
#3466=EDGE_LOOP('',(#15750));
#3467=EDGE_LOOP('',(#15751));
#3468=EDGE_LOOP('',(#15752,#15753,#15754,#15755));
#3469=EDGE_LOOP('',(#15756,#15757,#15758,#15759,#15760,#15761,#15762,#15763,
#15764,#15765,#15766,#15767,#15768,#15769));
#3470=EDGE_LOOP('',(#15770));
#3471=EDGE_LOOP('',(#15771,#15772,#15773,#15774,#15775,#15776));
#3472=EDGE_LOOP('',(#15777,#15778,#15779,#15780,#15781,#15782,#15783,#15784,
#15785,#15786,#15787,#15788));
#3473=EDGE_LOOP('',(#15789,#15790,#15791,#15792));
#3474=EDGE_LOOP('',(#15793,#15794,#15795,#15796));
#3475=EDGE_LOOP('',(#15797,#15798,#15799,#15800));
#3476=EDGE_LOOP('',(#15801,#15802,#15803,#15804));
#3477=EDGE_LOOP('',(#15805,#15806,#15807,#15808));
#3478=EDGE_LOOP('',(#15809,#15810,#15811,#15812));
#3479=EDGE_LOOP('',(#15813,#15814,#15815,#15816));
#3480=EDGE_LOOP('',(#15817,#15818,#15819,#15820));
#3481=EDGE_LOOP('',(#15821,#15822,#15823,#15824,#15825,#15826,#15827,#15828,
#15829,#15830,#15831,#15832));
#3482=EDGE_LOOP('',(#15833,#15834,#15835,#15836,#15837,#15838,#15839,#15840,
#15841,#15842,#15843,#15844));
#3483=EDGE_LOOP('',(#15845,#15846,#15847,#15848,#15849,#15850,#15851,#15852,
#15853,#15854,#15855,#15856));
#3484=EDGE_LOOP('',(#15857,#15858,#15859,#15860));
#3485=EDGE_LOOP('',(#15861,#15862,#15863,#15864));
#3486=EDGE_LOOP('',(#15865,#15866,#15867,#15868));
#3487=EDGE_LOOP('',(#15869,#15870,#15871,#15872));
#3488=EDGE_LOOP('',(#15873));
#3489=EDGE_LOOP('',(#15874,#15875,#15876,#15877));
#3490=EDGE_LOOP('',(#15878,#15879,#15880,#15881));
#3491=EDGE_LOOP('',(#15882,#15883,#15884,#15885));
#3492=EDGE_LOOP('',(#15886,#15887,#15888,#15889));
#3493=EDGE_LOOP('',(#15890,#15891,#15892,#15893));
#3494=EDGE_LOOP('',(#15894,#15895,#15896,#15897));
#3495=EDGE_LOOP('',(#15898,#15899,#15900,#15901));
#3496=EDGE_LOOP('',(#15902,#15903,#15904,#15905));
#3497=EDGE_LOOP('',(#15906));
#3498=EDGE_LOOP('',(#15907,#15908,#15909,#15910));
#3499=EDGE_LOOP('',(#15911,#15912,#15913,#15914));
#3500=EDGE_LOOP('',(#15915,#15916,#15917,#15918));
#3501=EDGE_LOOP('',(#15919,#15920,#15921,#15922));
#3502=EDGE_LOOP('',(#15923));
#3503=EDGE_LOOP('',(#15924));
#3504=EDGE_LOOP('',(#15925));
#3505=EDGE_LOOP('',(#15926,#15927,#15928,#15929));
#3506=EDGE_LOOP('',(#15930,#15931,#15932,#15933));
#3507=EDGE_LOOP('',(#15934,#15935,#15936,#15937));
#3508=EDGE_LOOP('',(#15938,#15939,#15940,#15941));
#3509=EDGE_LOOP('',(#15942,#15943,#15944,#15945));
#3510=EDGE_LOOP('',(#15946,#15947,#15948,#15949));
#3511=EDGE_LOOP('',(#15950,#15951,#15952,#15953,#15954,#15955));
#3512=EDGE_LOOP('',(#15956,#15957,#15958,#15959));
#3513=EDGE_LOOP('',(#15960,#15961,#15962,#15963));
#3514=EDGE_LOOP('',(#15964,#15965,#15966,#15967));
#3515=EDGE_LOOP('',(#15968,#15969,#15970,#15971));
#3516=EDGE_LOOP('',(#15972,#15973,#15974,#15975));
#3517=EDGE_LOOP('',(#15976,#15977,#15978,#15979));
#3518=EDGE_LOOP('',(#15980,#15981,#15982,#15983,#15984));
#3519=EDGE_LOOP('',(#15985));
#3520=EDGE_LOOP('',(#15986));
#3521=EDGE_LOOP('',(#15987,#15988,#15989,#15990));
#3522=EDGE_LOOP('',(#15991,#15992,#15993,#15994));
#3523=EDGE_LOOP('',(#15995,#15996,#15997,#15998));
#3524=EDGE_LOOP('',(#15999,#16000,#16001,#16002));
#3525=EDGE_LOOP('',(#16003,#16004,#16005,#16006));
#3526=EDGE_LOOP('',(#16007,#16008,#16009,#16010));
#3527=EDGE_LOOP('',(#16011,#16012,#16013,#16014));
#3528=EDGE_LOOP('',(#16015,#16016,#16017,#16018));
#3529=EDGE_LOOP('',(#16019,#16020,#16021,#16022));
#3530=EDGE_LOOP('',(#16023,#16024,#16025,#16026));
#3531=EDGE_LOOP('',(#16027,#16028,#16029,#16030));
#3532=EDGE_LOOP('',(#16031,#16032,#16033,#16034));
#3533=EDGE_LOOP('',(#16035,#16036,#16037,#16038));
#3534=EDGE_LOOP('',(#16039,#16040,#16041,#16042));
#3535=EDGE_LOOP('',(#16043,#16044,#16045,#16046));
#3536=EDGE_LOOP('',(#16047,#16048,#16049,#16050));
#3537=EDGE_LOOP('',(#16051,#16052,#16053,#16054));
#3538=EDGE_LOOP('',(#16055,#16056,#16057,#16058));
#3539=EDGE_LOOP('',(#16059,#16060,#16061,#16062));
#3540=EDGE_LOOP('',(#16063,#16064,#16065,#16066));
#3541=EDGE_LOOP('',(#16067,#16068,#16069,#16070));
#3542=EDGE_LOOP('',(#16071,#16072,#16073,#16074));
#3543=EDGE_LOOP('',(#16075,#16076,#16077,#16078));
#3544=EDGE_LOOP('',(#16079,#16080,#16081,#16082));
#3545=EDGE_LOOP('',(#16083,#16084,#16085,#16086));
#3546=EDGE_LOOP('',(#16087,#16088,#16089,#16090));
#3547=EDGE_LOOP('',(#16091,#16092,#16093,#16094));
#3548=EDGE_LOOP('',(#16095,#16096,#16097,#16098));
#3549=EDGE_LOOP('',(#16099,#16100,#16101,#16102));
#3550=EDGE_LOOP('',(#16103,#16104,#16105,#16106));
#3551=EDGE_LOOP('',(#16107,#16108,#16109,#16110));
#3552=EDGE_LOOP('',(#16111,#16112,#16113,#16114));
#3553=EDGE_LOOP('',(#16115,#16116,#16117,#16118));
#3554=EDGE_LOOP('',(#16119,#16120,#16121,#16122));
#3555=EDGE_LOOP('',(#16123,#16124,#16125,#16126));
#3556=EDGE_LOOP('',(#16127,#16128,#16129,#16130));
#3557=EDGE_LOOP('',(#16131,#16132,#16133,#16134));
#3558=EDGE_LOOP('',(#16135,#16136,#16137,#16138));
#3559=EDGE_LOOP('',(#16139,#16140,#16141,#16142));
#3560=EDGE_LOOP('',(#16143,#16144,#16145,#16146));
#3561=EDGE_LOOP('',(#16147,#16148,#16149,#16150));
#3562=EDGE_LOOP('',(#16151,#16152,#16153,#16154));
#3563=EDGE_LOOP('',(#16155,#16156,#16157,#16158));
#3564=EDGE_LOOP('',(#16159,#16160,#16161,#16162));
#3565=EDGE_LOOP('',(#16163,#16164,#16165,#16166,#16167,#16168,#16169,#16170,
#16171,#16172,#16173,#16174,#16175,#16176,#16177,#16178,#16179,#16180,#16181,
#16182,#16183,#16184,#16185,#16186,#16187,#16188,#16189,#16190,#16191,#16192,
#16193,#16194,#16195,#16196,#16197,#16198,#16199,#16200,#16201,#16202,#16203,
#16204,#16205));
#3566=EDGE_LOOP('',(#16206));
#3567=EDGE_LOOP('',(#16207,#16208,#16209,#16210,#16211,#16212,#16213,#16214,
#16215,#16216,#16217,#16218,#16219,#16220,#16221,#16222,#16223,#16224,#16225,
#16226,#16227,#16228,#16229,#16230,#16231,#16232,#16233,#16234,#16235,#16236,
#16237,#16238,#16239,#16240,#16241,#16242,#16243,#16244,#16245,#16246,#16247,
#16248,#16249));
#3568=EDGE_LOOP('',(#16250));
#3569=EDGE_LOOP('',(#16251));
#4999=LINE('',#33763,#6709);
#5000=LINE('',#33765,#6710);
#5001=LINE('',#33769,#6711);
#5002=LINE('',#33771,#6712);
#5003=LINE('',#33799,#6713);
#5004=LINE('',#33875,#6714);
#5005=LINE('',#33953,#6715);
#5006=LINE('',#34029,#6716);
#5007=LINE('',#34105,#6717);
#5008=LINE('',#34181,#6718);
#5009=LINE('',#34259,#6719);
#5010=LINE('',#34335,#6720);
#5011=LINE('',#34411,#6721);
#5012=LINE('',#34489,#6722);
#5013=LINE('',#34565,#6723);
#5014=LINE('',#34641,#6724);
#5015=LINE('',#34717,#6725);
#5016=LINE('',#34731,#6726);
#5017=LINE('',#34741,#6727);
#5018=LINE('',#34752,#6728);
#5019=LINE('',#34782,#6729);
#5020=LINE('',#34812,#6730);
#5021=LINE('',#34842,#6731);
#5022=LINE('',#34872,#6732);
#5023=LINE('',#34902,#6733);
#5024=LINE('',#34932,#6734);
#5025=LINE('',#34962,#6735);
#5026=LINE('',#34992,#6736);
#5027=LINE('',#35022,#6737);
#5028=LINE('',#35052,#6738);
#5029=LINE('',#35082,#6739);
#5030=LINE('',#35112,#6740);
#5031=LINE('',#35122,#6741);
#5032=LINE('',#35134,#6742);
#5033=LINE('',#35140,#6743);
#5034=LINE('',#35146,#6744);
#5035=LINE('',#35181,#6745);
#5036=LINE('',#35183,#6746);
#5037=LINE('',#35209,#6747);
#5038=LINE('',#35548,#6748);
#5039=LINE('',#35562,#6749);
#5040=LINE('',#35951,#6750);
#5041=LINE('',#35996,#6751);
#5042=LINE('',#35998,#6752);
#5043=LINE('',#36004,#6753);
#5044=LINE('',#36007,#6754);
#5045=LINE('',#36014,#6755);
#5046=LINE('',#36032,#6756);
#5047=LINE('',#36036,#6757);
#5048=LINE('',#36042,#6758);
#5049=LINE('',#36045,#6759);
#5050=LINE('',#36050,#6760);
#5051=LINE('',#36055,#6761);
#5052=LINE('',#36057,#6762);
#5053=LINE('',#36059,#6763);
#5054=LINE('',#36061,#6764);
#5055=LINE('',#36063,#6765);
#5056=LINE('',#36065,#6766);
#5057=LINE('',#36067,#6767);
#5058=LINE('',#36071,#6768);
#5059=LINE('',#36073,#6769);
#5060=LINE('',#36075,#6770);
#5061=LINE('',#36077,#6771);
#5062=LINE('',#36079,#6772);
#5063=LINE('',#36080,#6773);
#5064=LINE('',#36086,#6774);
#5065=LINE('',#36089,#6775);
#5066=LINE('',#36093,#6776);
#5067=LINE('',#36095,#6777);
#5068=LINE('',#36097,#6778);
#5069=LINE('',#36099,#6779);
#5070=LINE('',#36101,#6780);
#5071=LINE('',#36103,#6781);
#5072=LINE('',#36105,#6782);
#5073=LINE('',#36107,#6783);
#5074=LINE('',#36109,#6784);
#5075=LINE('',#36113,#6785);
#5076=LINE('',#36115,#6786);
#5077=LINE('',#36117,#6787);
#5078=LINE('',#36118,#6788);
#5079=LINE('',#36123,#6789);
#5080=LINE('',#36125,#6790);
#5081=LINE('',#36127,#6791);
#5082=LINE('',#36129,#6792);
#5083=LINE('',#36131,#6793);
#5084=LINE('',#36132,#6794);
#5085=LINE('',#36135,#6795);
#5086=LINE('',#36139,#6796);
#5087=LINE('',#36141,#6797);
#5088=LINE('',#36145,#6798);
#5089=LINE('',#36148,#6799);
#5090=LINE('',#36150,#6800);
#5091=LINE('',#36152,#6801);
#5092=LINE('',#36154,#6802);
#5093=LINE('',#36156,#6803);
#5094=LINE('',#36158,#6804);
#5095=LINE('',#36160,#6805);
#5096=LINE('',#36162,#6806);
#5097=LINE('',#36164,#6807);
#5098=LINE('',#36169,#6808);
#5099=LINE('',#36172,#6809);
#5100=LINE('',#36174,#6810);
#5101=LINE('',#36178,#6811);
#5102=LINE('',#36183,#6812);
#5103=LINE('',#36185,#6813);
#5104=LINE('',#36189,#6814);
#5105=LINE('',#36192,#6815);
#5106=LINE('',#36194,#6816);
#5107=LINE('',#36199,#6817);
#5108=LINE('',#36202,#6818);
#5109=LINE('',#36204,#6819);
#5110=LINE('',#36208,#6820);
#5111=LINE('',#36212,#6821);
#5112=LINE('',#36214,#6822);
#5113=LINE('',#36215,#6823);
#5114=LINE('',#36217,#6824);
#5115=LINE('',#36218,#6825);
#5116=LINE('',#36220,#6826);
#5117=LINE('',#36226,#6827);
#5118=LINE('',#36228,#6828);
#5119=LINE('',#36229,#6829);
#5120=LINE('',#36231,#6830);
#5121=LINE('',#36232,#6831);
#5122=LINE('',#36234,#6832);
#5123=LINE('',#36243,#6833);
#5124=LINE('',#36245,#6834);
#5125=LINE('',#36246,#6835);
#5126=LINE('',#36249,#6836);
#5127=LINE('',#36250,#6837);
#5128=LINE('',#36253,#6838);
#5129=LINE('',#36254,#6839);
#5130=LINE('',#36257,#6840);
#5131=LINE('',#36258,#6841);
#5132=LINE('',#36261,#6842);
#5133=LINE('',#36262,#6843);
#5134=LINE('',#36264,#6844);
#5135=LINE('',#36268,#6845);
#5136=LINE('',#36270,#6846);
#5137=LINE('',#36272,#6847);
#5138=LINE('',#36274,#6848);
#5139=LINE('',#36276,#6849);
#5140=LINE('',#36277,#6850);
#5141=LINE('',#36291,#6851);
#5142=LINE('',#36297,#6852);
#5143=LINE('',#36302,#6853);
#5144=LINE('',#36304,#6854);
#5145=LINE('',#36306,#6855);
#5146=LINE('',#36307,#6856);
#5147=LINE('',#36312,#6857);
#5148=LINE('',#36316,#6858);
#5149=LINE('',#36318,#6859);
#5150=LINE('',#36319,#6860);
#5151=LINE('',#36322,#6861);
#5152=LINE('',#36324,#6862);
#5153=LINE('',#36325,#6863);
#5154=LINE('',#36328,#6864);
#5155=LINE('',#36330,#6865);
#5156=LINE('',#36331,#6866);
#5157=LINE('',#36334,#6867);
#5158=LINE('',#36336,#6868);
#5159=LINE('',#36337,#6869);
#5160=LINE('',#36340,#6870);
#5161=LINE('',#36342,#6871);
#5162=LINE('',#36343,#6872);
#5163=LINE('',#36346,#6873);
#5164=LINE('',#36348,#6874);
#5165=LINE('',#36349,#6875);
#5166=LINE('',#36352,#6876);
#5167=LINE('',#36354,#6877);
#5168=LINE('',#36355,#6878);
#5169=LINE('',#36358,#6879);
#5170=LINE('',#36360,#6880);
#5171=LINE('',#36361,#6881);
#5172=LINE('',#36364,#6882);
#5173=LINE('',#36366,#6883);
#5174=LINE('',#36367,#6884);
#5175=LINE('',#36370,#6885);
#5176=LINE('',#36372,#6886);
#5177=LINE('',#36373,#6887);
#5178=LINE('',#36376,#6888);
#5179=LINE('',#36378,#6889);
#5180=LINE('',#36379,#6890);
#5181=LINE('',#36382,#6891);
#5182=LINE('',#36384,#6892);
#5183=LINE('',#36385,#6893);
#5184=LINE('',#36388,#6894);
#5185=LINE('',#36390,#6895);
#5186=LINE('',#36391,#6896);
#5187=LINE('',#36394,#6897);
#5188=LINE('',#36396,#6898);
#5189=LINE('',#36397,#6899);
#5190=LINE('',#36400,#6900);
#5191=LINE('',#36402,#6901);
#5192=LINE('',#36403,#6902);
#5193=LINE('',#36406,#6903);
#5194=LINE('',#36408,#6904);
#5195=LINE('',#36409,#6905);
#5196=LINE('',#36412,#6906);
#5197=LINE('',#36414,#6907);
#5198=LINE('',#36415,#6908);
#5199=LINE('',#36418,#6909);
#5200=LINE('',#36420,#6910);
#5201=LINE('',#36421,#6911);
#5202=LINE('',#36424,#6912);
#5203=LINE('',#36426,#6913);
#5204=LINE('',#36427,#6914);
#5205=LINE('',#36430,#6915);
#5206=LINE('',#36432,#6916);
#5207=LINE('',#36433,#6917);
#5208=LINE('',#36436,#6918);
#5209=LINE('',#36438,#6919);
#5210=LINE('',#36439,#6920);
#5211=LINE('',#36442,#6921);
#5212=LINE('',#36444,#6922);
#5213=LINE('',#36445,#6923);
#5214=LINE('',#36448,#6924);
#5215=LINE('',#36450,#6925);
#5216=LINE('',#36451,#6926);
#5217=LINE('',#36454,#6927);
#5218=LINE('',#36456,#6928);
#5219=LINE('',#36457,#6929);
#5220=LINE('',#36460,#6930);
#5221=LINE('',#36462,#6931);
#5222=LINE('',#36463,#6932);
#5223=LINE('',#36466,#6933);
#5224=LINE('',#36468,#6934);
#5225=LINE('',#36469,#6935);
#5226=LINE('',#36472,#6936);
#5227=LINE('',#36474,#6937);
#5228=LINE('',#36475,#6938);
#5229=LINE('',#36478,#6939);
#5230=LINE('',#36480,#6940);
#5231=LINE('',#36481,#6941);
#5232=LINE('',#36484,#6942);
#5233=LINE('',#36486,#6943);
#5234=LINE('',#36487,#6944);
#5235=LINE('',#36490,#6945);
#5236=LINE('',#36492,#6946);
#5237=LINE('',#36493,#6947);
#5238=LINE('',#36496,#6948);
#5239=LINE('',#36498,#6949);
#5240=LINE('',#36499,#6950);
#5241=LINE('',#36502,#6951);
#5242=LINE('',#36504,#6952);
#5243=LINE('',#36505,#6953);
#5244=LINE('',#36508,#6954);
#5245=LINE('',#36510,#6955);
#5246=LINE('',#36511,#6956);
#5247=LINE('',#36514,#6957);
#5248=LINE('',#36516,#6958);
#5249=LINE('',#36517,#6959);
#5250=LINE('',#36520,#6960);
#5251=LINE('',#36522,#6961);
#5252=LINE('',#36523,#6962);
#5253=LINE('',#36526,#6963);
#5254=LINE('',#36528,#6964);
#5255=LINE('',#36529,#6965);
#5256=LINE('',#36532,#6966);
#5257=LINE('',#36534,#6967);
#5258=LINE('',#36535,#6968);
#5259=LINE('',#36538,#6969);
#5260=LINE('',#36540,#6970);
#5261=LINE('',#36541,#6971);
#5262=LINE('',#36547,#6972);
#5263=LINE('',#36550,#6973);
#5264=LINE('',#36552,#6974);
#5265=LINE('',#36553,#6975);
#5266=LINE('',#36555,#6976);
#5267=LINE('',#36556,#6977);
#6709=VECTOR('',#23371,4.);
#6710=VECTOR('',#23374,4.);
#6711=VECTOR('',#23377,1.6);
#6712=VECTOR('',#23378,1000.);
#6713=VECTOR('',#23383,1.6);
#6714=VECTOR('',#23386,1.6);
#6715=VECTOR('',#23389,1.6);
#6716=VECTOR('',#23392,1.6);
#6717=VECTOR('',#23395,1.6);
#6718=VECTOR('',#23398,1.6);
#6719=VECTOR('',#23401,1.6);
#6720=VECTOR('',#23404,1.6);
#6721=VECTOR('',#23407,1.6);
#6722=VECTOR('',#23410,1.6);
#6723=VECTOR('',#23413,1.6);
#6724=VECTOR('',#23416,1.6);
#6725=VECTOR('',#23419,1.6);
#6726=VECTOR('',#23424,1.22111388750008);
#6727=VECTOR('',#23425,1000.);
#6728=VECTOR('',#23428,1.22111388750008);
#6729=VECTOR('',#23431,1.22111388750008);
#6730=VECTOR('',#23434,1.22111388750008);
#6731=VECTOR('',#23437,1.22111388750008);
#6732=VECTOR('',#23440,1.22111388750008);
#6733=VECTOR('',#23443,1.22111388750008);
#6734=VECTOR('',#23446,1.22111388750008);
#6735=VECTOR('',#23449,1.22111388750008);
#6736=VECTOR('',#23452,1.22111388750008);
#6737=VECTOR('',#23455,1.22111388750008);
#6738=VECTOR('',#23458,1.22111388750008);
#6739=VECTOR('',#23461,1.22111388750008);
#6740=VECTOR('',#23464,1.22111388750008);
#6741=VECTOR('',#23465,1000.);
#6742=VECTOR('',#23470,1.60000000000001);
#6743=VECTOR('',#23477,1.49172584788676);
#6744=VECTOR('',#23484,1.04190416256385);
#6745=VECTOR('',#23529,3.25);
#6746=VECTOR('',#23532,12.);
#6747=VECTOR('',#23549,1000.);
#6748=VECTOR('',#23550,1000.);
#6749=VECTOR('',#23551,1000.);
#6750=VECTOR('',#23554,1000.);
#6751=VECTOR('',#23555,1000.);
#6752=VECTOR('',#23558,1000.);
#6753=VECTOR('',#23567,1.6);
#6754=VECTOR('',#23572,2.);
#6755=VECTOR('',#23579,3.6);
#6756=VECTOR('',#23606,5.);
#6757=VECTOR('',#23611,7.);
#6758=VECTOR('',#23616,1000.);
#6759=VECTOR('',#23619,1000.);
#6760=VECTOR('',#23624,1.6);
#6761=VECTOR('',#23629,1000.);
#6762=VECTOR('',#23630,1000.);
#6763=VECTOR('',#23631,1000.);
#6764=VECTOR('',#23632,1000.);
#6765=VECTOR('',#23633,1000.);
#6766=VECTOR('',#23634,1000.);
#6767=VECTOR('',#23635,1000.);
#6768=VECTOR('',#23638,1000.);
#6769=VECTOR('',#23639,1000.);
#6770=VECTOR('',#23640,1000.);
#6771=VECTOR('',#23641,1000.);
#6772=VECTOR('',#23642,1000.);
#6773=VECTOR('',#23643,1000.);
#6774=VECTOR('',#23648,1000.);
#6775=VECTOR('',#23651,1000.);
#6776=VECTOR('',#23654,1000.);
#6777=VECTOR('',#23655,1000.);
#6778=VECTOR('',#23656,1000.);
#6779=VECTOR('',#23657,1000.);
#6780=VECTOR('',#23658,1000.);
#6781=VECTOR('',#23659,1000.);
#6782=VECTOR('',#23660,1000.);
#6783=VECTOR('',#23661,1000.);
#6784=VECTOR('',#23662,1000.);
#6785=VECTOR('',#23665,1000.);
#6786=VECTOR('',#23666,1000.);
#6787=VECTOR('',#23667,1000.);
#6788=VECTOR('',#23668,1000.);
#6789=VECTOR('',#23671,1000.);
#6790=VECTOR('',#23672,1000.);
#6791=VECTOR('',#23673,1000.);
#6792=VECTOR('',#23674,1000.);
#6793=VECTOR('',#23675,1000.);
#6794=VECTOR('',#23676,1000.);
#6795=VECTOR('',#23679,1000.);
#6796=VECTOR('',#23682,1000.);
#6797=VECTOR('',#23685,1000.);
#6798=VECTOR('',#23688,1000.);
#6799=VECTOR('',#23691,1000.);
#6800=VECTOR('',#23694,1000.);
#6801=VECTOR('',#23697,1000.);
#6802=VECTOR('',#23700,1000.);
#6803=VECTOR('',#23703,1000.);
#6804=VECTOR('',#23706,1000.);
#6805=VECTOR('',#23709,1000.);
#6806=VECTOR('',#23712,1000.);
#6807=VECTOR('',#23715,1000.);
#6808=VECTOR('',#23720,1000.);
#6809=VECTOR('',#23723,1000.);
#6810=VECTOR('',#23724,1000.);
#6811=VECTOR('',#23727,1000.);
#6812=VECTOR('',#23732,1000.);
#6813=VECTOR('',#23735,1000.);
#6814=VECTOR('',#23738,1000.);
#6815=VECTOR('',#23741,1000.);
#6816=VECTOR('',#23742,1000.);
#6817=VECTOR('',#23747,1000.);
#6818=VECTOR('',#23750,1000.);
#6819=VECTOR('',#23751,1000.);
#6820=VECTOR('',#23754,1000.);
#6821=VECTOR('',#23761,1000.);
#6822=VECTOR('',#23764,1000.);
#6823=VECTOR('',#23765,1000.);
#6824=VECTOR('',#23768,1000.);
#6825=VECTOR('',#23769,1000.);
#6826=VECTOR('',#23772,1000.);
#6827=VECTOR('',#23783,1000.);
#6828=VECTOR('',#23786,1000.);
#6829=VECTOR('',#23787,1000.);
#6830=VECTOR('',#23790,1000.);
#6831=VECTOR('',#23791,1000.);
#6832=VECTOR('',#23794,1000.);
#6833=VECTOR('',#23809,1000.);
#6834=VECTOR('',#23810,1000.);
#6835=VECTOR('',#23811,1000.);
#6836=VECTOR('',#23814,1000.);
#6837=VECTOR('',#23815,1000.);
#6838=VECTOR('',#23818,1000.);
#6839=VECTOR('',#23819,1000.);
#6840=VECTOR('',#23822,1000.);
#6841=VECTOR('',#23823,1000.);
#6842=VECTOR('',#23826,1000.);
#6843=VECTOR('',#23827,1000.);
#6844=VECTOR('',#23830,1000.);
#6845=VECTOR('',#23833,1000.);
#6846=VECTOR('',#23834,1000.);
#6847=VECTOR('',#23835,1000.);
#6848=VECTOR('',#23836,1000.);
#6849=VECTOR('',#23837,1000.);
#6850=VECTOR('',#23838,1000.);
#6851=VECTOR('',#23865,4.);
#6852=VECTOR('',#23872,1.6);
#6853=VECTOR('',#23877,1000.);
#6854=VECTOR('',#23878,1000.);
#6855=VECTOR('',#23879,1000.);
#6856=VECTOR('',#23880,1000.);
#6857=VECTOR('',#23885,1000.);
#6858=VECTOR('',#23890,1000.);
#6859=VECTOR('',#23891,1000.);
#6860=VECTOR('',#23892,1000.);
#6861=VECTOR('',#23895,1000.);
#6862=VECTOR('',#23896,1000.);
#6863=VECTOR('',#23897,1000.);
#6864=VECTOR('',#23900,1000.);
#6865=VECTOR('',#23901,1000.);
#6866=VECTOR('',#23902,1000.);
#6867=VECTOR('',#23905,1000.);
#6868=VECTOR('',#23906,1000.);
#6869=VECTOR('',#23907,1000.);
#6870=VECTOR('',#23910,1000.);
#6871=VECTOR('',#23911,1000.);
#6872=VECTOR('',#23912,1000.);
#6873=VECTOR('',#23915,1000.);
#6874=VECTOR('',#23916,1000.);
#6875=VECTOR('',#23917,1000.);
#6876=VECTOR('',#23920,1000.);
#6877=VECTOR('',#23921,1000.);
#6878=VECTOR('',#23922,1000.);
#6879=VECTOR('',#23925,1000.);
#6880=VECTOR('',#23926,1000.);
#6881=VECTOR('',#23927,1000.);
#6882=VECTOR('',#23930,1000.);
#6883=VECTOR('',#23931,1000.);
#6884=VECTOR('',#23932,1000.);
#6885=VECTOR('',#23935,1000.);
#6886=VECTOR('',#23936,1000.);
#6887=VECTOR('',#23937,1000.);
#6888=VECTOR('',#23940,1000.);
#6889=VECTOR('',#23941,1000.);
#6890=VECTOR('',#23942,1000.);
#6891=VECTOR('',#23945,1000.);
#6892=VECTOR('',#23946,1000.);
#6893=VECTOR('',#23947,1000.);
#6894=VECTOR('',#23950,1000.);
#6895=VECTOR('',#23951,1000.);
#6896=VECTOR('',#23952,1000.);
#6897=VECTOR('',#23955,1000.);
#6898=VECTOR('',#23956,1000.);
#6899=VECTOR('',#23957,1000.);
#6900=VECTOR('',#23960,1000.);
#6901=VECTOR('',#23961,1000.);
#6902=VECTOR('',#23962,1000.);
#6903=VECTOR('',#23965,1000.);
#6904=VECTOR('',#23966,1000.);
#6905=VECTOR('',#23967,1000.);
#6906=VECTOR('',#23970,1000.);
#6907=VECTOR('',#23971,1000.);
#6908=VECTOR('',#23972,1000.);
#6909=VECTOR('',#23975,1000.);
#6910=VECTOR('',#23976,1000.);
#6911=VECTOR('',#23977,1000.);
#6912=VECTOR('',#23980,1000.);
#6913=VECTOR('',#23981,1000.);
#6914=VECTOR('',#23982,1000.);
#6915=VECTOR('',#23985,1000.);
#6916=VECTOR('',#23986,1000.);
#6917=VECTOR('',#23987,1000.);
#6918=VECTOR('',#23990,1000.);
#6919=VECTOR('',#23991,1000.);
#6920=VECTOR('',#23992,1000.);
#6921=VECTOR('',#23995,1000.);
#6922=VECTOR('',#23996,1000.);
#6923=VECTOR('',#23997,1000.);
#6924=VECTOR('',#24000,1000.);
#6925=VECTOR('',#24001,1000.);
#6926=VECTOR('',#24002,1000.);
#6927=VECTOR('',#24005,1000.);
#6928=VECTOR('',#24006,1000.);
#6929=VECTOR('',#24007,1000.);
#6930=VECTOR('',#24010,1000.);
#6931=VECTOR('',#24011,1000.);
#6932=VECTOR('',#24012,1000.);
#6933=VECTOR('',#24015,1000.);
#6934=VECTOR('',#24016,1000.);
#6935=VECTOR('',#24017,1000.);
#6936=VECTOR('',#24020,1000.);
#6937=VECTOR('',#24021,1000.);
#6938=VECTOR('',#24022,1000.);
#6939=VECTOR('',#24025,1000.);
#6940=VECTOR('',#24026,1000.);
#6941=VECTOR('',#24027,1000.);
#6942=VECTOR('',#24030,1000.);
#6943=VECTOR('',#24031,1000.);
#6944=VECTOR('',#24032,1000.);
#6945=VECTOR('',#24035,1000.);
#6946=VECTOR('',#24036,1000.);
#6947=VECTOR('',#24037,1000.);
#6948=VECTOR('',#24040,1000.);
#6949=VECTOR('',#24041,1000.);
#6950=VECTOR('',#24042,1000.);
#6951=VECTOR('',#24045,1000.);
#6952=VECTOR('',#24046,1000.);
#6953=VECTOR('',#24047,1000.);
#6954=VECTOR('',#24050,1000.);
#6955=VECTOR('',#24051,1000.);
#6956=VECTOR('',#24052,1000.);
#6957=VECTOR('',#24055,1000.);
#6958=VECTOR('',#24056,1000.);
#6959=VECTOR('',#24057,1000.);
#6960=VECTOR('',#24060,1000.);
#6961=VECTOR('',#24061,1000.);
#6962=VECTOR('',#24062,1000.);
#6963=VECTOR('',#24065,1000.);
#6964=VECTOR('',#24066,1000.);
#6965=VECTOR('',#24067,1000.);
#6966=VECTOR('',#24070,1000.);
#6967=VECTOR('',#24071,1000.);
#6968=VECTOR('',#24072,1000.);
#6969=VECTOR('',#24075,1000.);
#6970=VECTOR('',#24076,1000.);
#6971=VECTOR('',#24077,1000.);
#6972=VECTOR('',#24084,1000.);
#6973=VECTOR('',#24087,1000.);
#6974=VECTOR('',#24088,1000.);
#6975=VECTOR('',#24089,1000.);
#6976=VECTOR('',#24092,1000.);
#6977=VECTOR('',#24093,1000.);
#8367=VERTEX_POINT('',#33754);
#8368=VERTEX_POINT('',#33756);
#8369=VERTEX_POINT('',#33759);
#8370=VERTEX_POINT('',#33760);
#8371=VERTEX_POINT('',#33767);
#8372=VERTEX_POINT('',#33768);
#8373=VERTEX_POINT('',#33770);
#8374=VERTEX_POINT('',#33772);
#8375=VERTEX_POINT('',#33797);
#8376=VERTEX_POINT('',#33798);
#8377=VERTEX_POINT('',#33873);
#8378=VERTEX_POINT('',#33874);
#8379=VERTEX_POINT('',#33951);
#8380=VERTEX_POINT('',#33952);
#8381=VERTEX_POINT('',#34027);
#8382=VERTEX_POINT('',#34028);
#8383=VERTEX_POINT('',#34103);
#8384=VERTEX_POINT('',#34104);
#8385=VERTEX_POINT('',#34179);
#8386=VERTEX_POINT('',#34180);
#8387=VERTEX_POINT('',#34257);
#8388=VERTEX_POINT('',#34258);
#8389=VERTEX_POINT('',#34333);
#8390=VERTEX_POINT('',#34334);
#8391=VERTEX_POINT('',#34409);
#8392=VERTEX_POINT('',#34410);
#8393=VERTEX_POINT('',#34487);
#8394=VERTEX_POINT('',#34488);
#8395=VERTEX_POINT('',#34563);
#8396=VERTEX_POINT('',#34564);
#8397=VERTEX_POINT('',#34639);
#8398=VERTEX_POINT('',#34640);
#8399=VERTEX_POINT('',#34715);
#8400=VERTEX_POINT('',#34716);
#8401=VERTEX_POINT('',#34718);
#8402=VERTEX_POINT('',#34729);
#8403=VERTEX_POINT('',#34730);
#8404=VERTEX_POINT('',#34732);
#8405=VERTEX_POINT('',#34740);
#8406=VERTEX_POINT('',#34750);
#8407=VERTEX_POINT('',#34751);
#8408=VERTEX_POINT('',#34780);
#8409=VERTEX_POINT('',#34781);
#8410=VERTEX_POINT('',#34810);
#8411=VERTEX_POINT('',#34811);
#8412=VERTEX_POINT('',#34840);
#8413=VERTEX_POINT('',#34841);
#8414=VERTEX_POINT('',#34870);
#8415=VERTEX_POINT('',#34871);
#8416=VERTEX_POINT('',#34900);
#8417=VERTEX_POINT('',#34901);
#8418=VERTEX_POINT('',#34930);
#8419=VERTEX_POINT('',#34931);
#8420=VERTEX_POINT('',#34960);
#8421=VERTEX_POINT('',#34961);
#8422=VERTEX_POINT('',#34990);
#8423=VERTEX_POINT('',#34991);
#8424=VERTEX_POINT('',#35020);
#8425=VERTEX_POINT('',#35021);
#8426=VERTEX_POINT('',#35050);
#8427=VERTEX_POINT('',#35051);
#8428=VERTEX_POINT('',#35080);
#8429=VERTEX_POINT('',#35081);
#8430=VERTEX_POINT('',#35110);
#8431=VERTEX_POINT('',#35111);
#8432=VERTEX_POINT('',#35113);
#8433=VERTEX_POINT('',#35121);
#8434=VERTEX_POINT('',#35131);
#8435=VERTEX_POINT('',#35133);
#8436=VERTEX_POINT('',#35137);
#8437=VERTEX_POINT('',#35139);
#8438=VERTEX_POINT('',#35143);
#8439=VERTEX_POINT('',#35145);
#8440=VERTEX_POINT('',#35149);
#8441=VERTEX_POINT('',#35151);
#8442=VERTEX_POINT('',#35153);
#8443=VERTEX_POINT('',#35157);
#8444=VERTEX_POINT('',#35158);
#8445=VERTEX_POINT('',#35161);
#8446=VERTEX_POINT('',#35165);
#8447=VERTEX_POINT('',#35166);
#8448=VERTEX_POINT('',#35169);
#8449=VERTEX_POINT('',#35173);
#8450=VERTEX_POINT('',#35175);
#8451=VERTEX_POINT('',#35177);
#8452=VERTEX_POINT('',#35186);
#8453=VERTEX_POINT('',#35189);
#8454=VERTEX_POINT('',#35192);
#8455=VERTEX_POINT('',#35206);
#8456=VERTEX_POINT('',#35988);
#8457=VERTEX_POINT('',#36003);
#8458=VERTEX_POINT('',#36009);
#8459=VERTEX_POINT('',#36010);
#8460=VERTEX_POINT('',#36013);
#8461=VERTEX_POINT('',#36020);
#8462=VERTEX_POINT('',#36022);
#8463=VERTEX_POINT('',#36026);
#8464=VERTEX_POINT('',#36028);
#8465=VERTEX_POINT('',#36034);
#8466=VERTEX_POINT('',#36038);
#8467=VERTEX_POINT('',#36039);
#8468=VERTEX_POINT('',#36041);
#8469=VERTEX_POINT('',#36043);
#8470=VERTEX_POINT('',#36047);
#8471=VERTEX_POINT('',#36049);
#8472=VERTEX_POINT('',#36053);
#8473=VERTEX_POINT('',#36054);
#8474=VERTEX_POINT('',#36056);
#8475=VERTEX_POINT('',#36058);
#8476=VERTEX_POINT('',#36060);
#8477=VERTEX_POINT('',#36062);
#8478=VERTEX_POINT('',#36064);
#8479=VERTEX_POINT('',#36066);
#8480=VERTEX_POINT('',#36068);
#8481=VERTEX_POINT('',#36070);
#8482=VERTEX_POINT('',#36072);
#8483=VERTEX_POINT('',#36074);
#8484=VERTEX_POINT('',#36076);
#8485=VERTEX_POINT('',#36078);
#8486=VERTEX_POINT('',#36082);
#8487=VERTEX_POINT('',#36083);
#8488=VERTEX_POINT('',#36085);
#8489=VERTEX_POINT('',#36087);
#8490=VERTEX_POINT('',#36091);
#8491=VERTEX_POINT('',#36092);
#8492=VERTEX_POINT('',#36094);
#8493=VERTEX_POINT('',#36096);
#8494=VERTEX_POINT('',#36098);
#8495=VERTEX_POINT('',#36100);
#8496=VERTEX_POINT('',#36102);
#8497=VERTEX_POINT('',#36104);
#8498=VERTEX_POINT('',#36106);
#8499=VERTEX_POINT('',#36108);
#8500=VERTEX_POINT('',#36110);
#8501=VERTEX_POINT('',#36112);
#8502=VERTEX_POINT('',#36114);
#8503=VERTEX_POINT('',#36116);
#8504=VERTEX_POINT('',#36119);
#8505=VERTEX_POINT('',#36121);
#8506=VERTEX_POINT('',#36122);
#8507=VERTEX_POINT('',#36124);
#8508=VERTEX_POINT('',#36126);
#8509=VERTEX_POINT('',#36128);
#8510=VERTEX_POINT('',#36130);
#8511=VERTEX_POINT('',#36134);
#8512=VERTEX_POINT('',#36136);
#8513=VERTEX_POINT('',#36138);
#8514=VERTEX_POINT('',#36142);
#8515=VERTEX_POINT('',#36144);
#8516=VERTEX_POINT('',#36146);
#8517=VERTEX_POINT('',#36166);
#8518=VERTEX_POINT('',#36168);
#8519=VERTEX_POINT('',#36170);
#8520=VERTEX_POINT('',#36173);
#8521=VERTEX_POINT('',#36175);
#8522=VERTEX_POINT('',#36177);
#8523=VERTEX_POINT('',#36181);
#8524=VERTEX_POINT('',#36182);
#8525=VERTEX_POINT('',#36186);
#8526=VERTEX_POINT('',#36188);
#8527=VERTEX_POINT('',#36190);
#8528=VERTEX_POINT('',#36193);
#8529=VERTEX_POINT('',#36197);
#8530=VERTEX_POINT('',#36198);
#8531=VERTEX_POINT('',#36200);
#8532=VERTEX_POINT('',#36203);
#8533=VERTEX_POINT('',#36205);
#8534=VERTEX_POINT('',#36207);
#8535=VERTEX_POINT('',#36242);
#8536=VERTEX_POINT('',#36244);
#8537=VERTEX_POINT('',#36248);
#8538=VERTEX_POINT('',#36252);
#8539=VERTEX_POINT('',#36256);
#8540=VERTEX_POINT('',#36260);
#8541=VERTEX_POINT('',#36266);
#8542=VERTEX_POINT('',#36267);
#8543=VERTEX_POINT('',#36269);
#8544=VERTEX_POINT('',#36271);
#8545=VERTEX_POINT('',#36273);
#8546=VERTEX_POINT('',#36275);
#8547=VERTEX_POINT('',#36293);
#8548=VERTEX_POINT('',#36296);
#8549=VERTEX_POINT('',#36300);
#8550=VERTEX_POINT('',#36301);
#8551=VERTEX_POINT('',#36303);
#8552=VERTEX_POINT('',#36305);
#8553=VERTEX_POINT('',#36309);
#8554=VERTEX_POINT('',#36311);
#8555=VERTEX_POINT('',#36315);
#8556=VERTEX_POINT('',#36317);
#8557=VERTEX_POINT('',#36321);
#8558=VERTEX_POINT('',#36323);
#8559=VERTEX_POINT('',#36327);
#8560=VERTEX_POINT('',#36329);
#8561=VERTEX_POINT('',#36333);
#8562=VERTEX_POINT('',#36335);
#8563=VERTEX_POINT('',#36339);
#8564=VERTEX_POINT('',#36341);
#8565=VERTEX_POINT('',#36345);
#8566=VERTEX_POINT('',#36347);
#8567=VERTEX_POINT('',#36351);
#8568=VERTEX_POINT('',#36353);
#8569=VERTEX_POINT('',#36357);
#8570=VERTEX_POINT('',#36359);
#8571=VERTEX_POINT('',#36363);
#8572=VERTEX_POINT('',#36365);
#8573=VERTEX_POINT('',#36369);
#8574=VERTEX_POINT('',#36371);
#8575=VERTEX_POINT('',#36375);
#8576=VERTEX_POINT('',#36377);
#8577=VERTEX_POINT('',#36381);
#8578=VERTEX_POINT('',#36383);
#8579=VERTEX_POINT('',#36387);
#8580=VERTEX_POINT('',#36389);
#8581=VERTEX_POINT('',#36393);
#8582=VERTEX_POINT('',#36395);
#8583=VERTEX_POINT('',#36399);
#8584=VERTEX_POINT('',#36401);
#8585=VERTEX_POINT('',#36405);
#8586=VERTEX_POINT('',#36407);
#8587=VERTEX_POINT('',#36411);
#8588=VERTEX_POINT('',#36413);
#8589=VERTEX_POINT('',#36417);
#8590=VERTEX_POINT('',#36419);
#8591=VERTEX_POINT('',#36423);
#8592=VERTEX_POINT('',#36425);
#8593=VERTEX_POINT('',#36429);
#8594=VERTEX_POINT('',#36431);
#8595=VERTEX_POINT('',#36435);
#8596=VERTEX_POINT('',#36437);
#8597=VERTEX_POINT('',#36441);
#8598=VERTEX_POINT('',#36443);
#8599=VERTEX_POINT('',#36447);
#8600=VERTEX_POINT('',#36449);
#8601=VERTEX_POINT('',#36453);
#8602=VERTEX_POINT('',#36455);
#8603=VERTEX_POINT('',#36459);
#8604=VERTEX_POINT('',#36461);
#8605=VERTEX_POINT('',#36465);
#8606=VERTEX_POINT('',#36467);
#8607=VERTEX_POINT('',#36471);
#8608=VERTEX_POINT('',#36473);
#8609=VERTEX_POINT('',#36477);
#8610=VERTEX_POINT('',#36479);
#8611=VERTEX_POINT('',#36483);
#8612=VERTEX_POINT('',#36485);
#8613=VERTEX_POINT('',#36489);
#8614=VERTEX_POINT('',#36491);
#8615=VERTEX_POINT('',#36495);
#8616=VERTEX_POINT('',#36497);
#8617=VERTEX_POINT('',#36501);
#8618=VERTEX_POINT('',#36503);
#8619=VERTEX_POINT('',#36507);
#8620=VERTEX_POINT('',#36509);
#8621=VERTEX_POINT('',#36513);
#8622=VERTEX_POINT('',#36515);
#8623=VERTEX_POINT('',#36519);
#8624=VERTEX_POINT('',#36521);
#8625=VERTEX_POINT('',#36525);
#8626=VERTEX_POINT('',#36527);
#8627=VERTEX_POINT('',#36531);
#8628=VERTEX_POINT('',#36533);
#8629=VERTEX_POINT('',#36537);
#8630=VERTEX_POINT('',#36539);
#8631=VERTEX_POINT('',#36543);
#8632=VERTEX_POINT('',#36545);
#8633=VERTEX_POINT('',#36549);
#8634=VERTEX_POINT('',#36551);
#10768=EDGE_CURVE('',#8367,#8367,#1456,.T.);
#10769=EDGE_CURVE('',#8368,#8368,#1457,.T.);
#10770=EDGE_CURVE('',#8369,#8370,#1458,.T.);
#10771=EDGE_CURVE('',#8370,#8369,#1459,.T.);
#10772=EDGE_CURVE('',#8370,#8368,#4999,.T.);
#10773=EDGE_CURVE('',#8367,#8369,#5000,.T.);
#10774=EDGE_CURVE('',#8371,#8372,#5001,.T.);
#10775=EDGE_CURVE('',#8372,#8373,#5002,.T.);
#10776=EDGE_CURVE('',#8373,#8374,#1460,.T.);
#10777=EDGE_CURVE('',#8371,#8374,#357,.T.);
#10778=EDGE_CURVE('',#8375,#8376,#5003,.T.);
#10779=EDGE_CURVE('',#8376,#8372,#358,.F.);
#10780=EDGE_CURVE('',#8375,#8371,#359,.T.);
#10781=EDGE_CURVE('',#8377,#8378,#5004,.T.);
#10782=EDGE_CURVE('',#8378,#8376,#360,.F.);
#10783=EDGE_CURVE('',#8377,#8375,#361,.T.);
#10784=EDGE_CURVE('',#8379,#8380,#5005,.T.);
#10785=EDGE_CURVE('',#8380,#8378,#362,.F.);
#10786=EDGE_CURVE('',#8379,#8377,#363,.T.);
#10787=EDGE_CURVE('',#8381,#8382,#5006,.T.);
#10788=EDGE_CURVE('',#8382,#8380,#364,.F.);
#10789=EDGE_CURVE('',#8381,#8379,#365,.T.);
#10790=EDGE_CURVE('',#8383,#8384,#5007,.T.);
#10791=EDGE_CURVE('',#8384,#8382,#366,.F.);
#10792=EDGE_CURVE('',#8383,#8381,#367,.T.);
#10793=EDGE_CURVE('',#8385,#8386,#5008,.T.);
#10794=EDGE_CURVE('',#8386,#8384,#368,.F.);
#10795=EDGE_CURVE('',#8385,#8383,#369,.T.);
#10796=EDGE_CURVE('',#8387,#8388,#5009,.T.);
#10797=EDGE_CURVE('',#8388,#8386,#370,.F.);
#10798=EDGE_CURVE('',#8387,#8385,#371,.T.);
#10799=EDGE_CURVE('',#8389,#8390,#5010,.T.);
#10800=EDGE_CURVE('',#8390,#8388,#372,.F.);
#10801=EDGE_CURVE('',#8389,#8387,#373,.T.);
#10802=EDGE_CURVE('',#8391,#8392,#5011,.T.);
#10803=EDGE_CURVE('',#8392,#8390,#374,.F.);
#10804=EDGE_CURVE('',#8391,#8389,#375,.T.);
#10805=EDGE_CURVE('',#8393,#8394,#5012,.T.);
#10806=EDGE_CURVE('',#8394,#8392,#376,.F.);
#10807=EDGE_CURVE('',#8393,#8391,#377,.T.);
#10808=EDGE_CURVE('',#8395,#8396,#5013,.T.);
#10809=EDGE_CURVE('',#8396,#8394,#378,.F.);
#10810=EDGE_CURVE('',#8395,#8393,#379,.T.);
#10811=EDGE_CURVE('',#8397,#8398,#5014,.T.);
#10812=EDGE_CURVE('',#8398,#8396,#380,.F.);
#10813=EDGE_CURVE('',#8397,#8395,#381,.T.);
#10814=EDGE_CURVE('',#8399,#8400,#5015,.T.);
#10815=EDGE_CURVE('',#8399,#8401,#1461,.T.);
#10816=EDGE_CURVE('',#8401,#8400,#382,.F.);
#10817=EDGE_CURVE('',#8402,#8403,#5016,.T.);
#10818=EDGE_CURVE('',#8403,#8404,#136,.T.);
#10819=EDGE_CURVE('',#8404,#8405,#5017,.T.);
#10820=EDGE_CURVE('',#8402,#8405,#137,.T.);
#10821=EDGE_CURVE('',#8406,#8407,#5018,.T.);
#10822=EDGE_CURVE('',#8407,#8403,#138,.T.);
#10823=EDGE_CURVE('',#8406,#8402,#139,.T.);
#10824=EDGE_CURVE('',#8408,#8409,#5019,.T.);
#10825=EDGE_CURVE('',#8409,#8407,#140,.T.);
#10826=EDGE_CURVE('',#8408,#8406,#141,.T.);
#10827=EDGE_CURVE('',#8410,#8411,#5020,.T.);
#10828=EDGE_CURVE('',#8411,#8409,#142,.T.);
#10829=EDGE_CURVE('',#8410,#8408,#143,.T.);
#10830=EDGE_CURVE('',#8412,#8413,#5021,.T.);
#10831=EDGE_CURVE('',#8413,#8411,#144,.T.);
#10832=EDGE_CURVE('',#8412,#8410,#145,.T.);
#10833=EDGE_CURVE('',#8414,#8415,#5022,.T.);
#10834=EDGE_CURVE('',#8415,#8413,#146,.T.);
#10835=EDGE_CURVE('',#8414,#8412,#147,.T.);
#10836=EDGE_CURVE('',#8416,#8417,#5023,.T.);
#10837=EDGE_CURVE('',#8417,#8415,#148,.T.);
#10838=EDGE_CURVE('',#8416,#8414,#149,.T.);
#10839=EDGE_CURVE('',#8418,#8419,#5024,.T.);
#10840=EDGE_CURVE('',#8419,#8417,#150,.T.);
#10841=EDGE_CURVE('',#8418,#8416,#151,.T.);
#10842=EDGE_CURVE('',#8420,#8421,#5025,.T.);
#10843=EDGE_CURVE('',#8421,#8419,#152,.T.);
#10844=EDGE_CURVE('',#8420,#8418,#153,.T.);
#10845=EDGE_CURVE('',#8422,#8423,#5026,.T.);
#10846=EDGE_CURVE('',#8423,#8421,#154,.T.);
#10847=EDGE_CURVE('',#8422,#8420,#155,.T.);
#10848=EDGE_CURVE('',#8424,#8425,#5027,.T.);
#10849=EDGE_CURVE('',#8425,#8423,#156,.T.);
#10850=EDGE_CURVE('',#8424,#8422,#157,.T.);
#10851=EDGE_CURVE('',#8426,#8427,#5028,.T.);
#10852=EDGE_CURVE('',#8427,#8425,#158,.T.);
#10853=EDGE_CURVE('',#8426,#8424,#159,.T.);
#10854=EDGE_CURVE('',#8428,#8429,#5029,.T.);
#10855=EDGE_CURVE('',#8429,#8427,#160,.T.);
#10856=EDGE_CURVE('',#8428,#8426,#161,.T.);
#10857=EDGE_CURVE('',#8430,#8431,#5030,.T.);
#10858=EDGE_CURVE('',#8432,#8430,#162,.T.);
#10859=EDGE_CURVE('',#8432,#8433,#5031,.T.);
#10860=EDGE_CURVE('',#8433,#8431,#163,.T.);
#10861=EDGE_CURVE('',#8434,#8434,#1462,.T.);
#10862=EDGE_CURVE('',#8434,#8435,#5032,.T.);
#10863=EDGE_CURVE('',#8435,#8435,#1463,.T.);
#10864=EDGE_CURVE('',#8436,#8436,#1464,.T.);
#10865=EDGE_CURVE('',#8436,#8437,#5033,.T.);
#10866=EDGE_CURVE('',#8437,#8437,#1465,.T.);
#10867=EDGE_CURVE('',#8438,#8438,#1466,.T.);
#10868=EDGE_CURVE('',#8438,#8439,#5034,.T.);
#10869=EDGE_CURVE('',#8439,#8439,#1467,.T.);
#10870=EDGE_CURVE('',#8440,#8440,#1468,.T.);
#10871=EDGE_CURVE('',#8440,#8441,#1469,.T.);
#10872=EDGE_CURVE('',#8442,#8441,#1470,.T.);
#10873=EDGE_CURVE('',#8441,#8442,#1471,.T.);
#10874=EDGE_CURVE('',#8443,#8444,#1472,.T.);
#10875=EDGE_CURVE('',#8444,#8443,#1473,.T.);
#10876=EDGE_CURVE('',#8444,#8445,#1474,.T.);
#10877=EDGE_CURVE('',#8445,#8445,#1475,.T.);
#10878=EDGE_CURVE('',#8446,#8447,#1476,.T.);
#10879=EDGE_CURVE('',#8447,#8446,#1477,.T.);
#10880=EDGE_CURVE('',#8447,#8448,#1478,.T.);
#10881=EDGE_CURVE('',#8448,#8448,#1479,.T.);
#10882=EDGE_CURVE('',#8449,#8449,#1480,.T.);
#10883=EDGE_CURVE('',#8449,#8450,#1481,.T.);
#10884=EDGE_CURVE('',#8451,#8450,#1482,.T.);
#10885=EDGE_CURVE('',#8450,#8451,#1483,.T.);
#10886=EDGE_CURVE('',#8446,#8451,#5035,.T.);
#10887=EDGE_CURVE('',#8443,#8442,#5036,.T.);
#10888=EDGE_CURVE('',#8452,#8452,#1484,.T.);
#10889=EDGE_CURVE('',#8453,#8453,#1485,.T.);
#10890=EDGE_CURVE('',#8454,#8401,#164,.T.);
#10891=EDGE_CURVE('',#8401,#8455,#1486,.T.);
#10892=EDGE_CURVE('',#8455,#8399,#1487,.T.);
#10893=EDGE_CURVE('',#8399,#8454,#5037,.T.);
#10894=EDGE_CURVE('',#8454,#8432,#5038,.T.);
#10895=EDGE_CURVE('',#8430,#8428,#165,.T.);
#10896=EDGE_CURVE('',#8405,#8372,#5039,.T.);
#10897=EDGE_CURVE('',#8400,#8398,#383,.F.);
#10898=EDGE_CURVE('',#8431,#8429,#166,.T.);
#10899=EDGE_CURVE('',#8433,#8399,#5040,.T.);
#10900=EDGE_CURVE('',#8399,#8397,#384,.T.);
#10901=EDGE_CURVE('',#8374,#8456,#167,.T.);
#10902=EDGE_CURVE('',#8456,#8404,#5041,.T.);
#10903=EDGE_CURVE('',#8373,#8456,#5042,.T.);
#10904=EDGE_CURVE('',#8374,#8373,#1488,.T.);
#10905=EDGE_CURVE('',#8455,#8457,#5043,.T.);
#10906=EDGE_CURVE('',#8457,#8457,#1489,.T.);
#10907=EDGE_CURVE('',#8373,#8453,#5044,.T.);
#10908=EDGE_CURVE('',#8458,#8459,#1490,.T.);
#10909=EDGE_CURVE('',#8459,#8458,#1491,.T.);
#10910=EDGE_CURVE('',#8459,#8460,#5045,.T.);
#10911=EDGE_CURVE('',#8460,#8460,#1492,.T.);
#10912=EDGE_CURVE('',#8461,#8461,#1493,.T.);
#10913=EDGE_CURVE('',#8461,#8462,#1494,.T.);
#10914=EDGE_CURVE('',#8462,#8462,#1495,.T.);
#10915=EDGE_CURVE('',#8463,#8463,#1496,.T.);
#10916=EDGE_CURVE('',#8463,#8464,#1497,.T.);
#10917=EDGE_CURVE('',#8464,#8464,#1498,.T.);
#10918=EDGE_CURVE('',#8464,#8461,#5046,.T.);
#10919=EDGE_CURVE('',#8465,#8465,#1499,.T.);
#10920=EDGE_CURVE('',#8465,#8452,#5047,.T.);
#10921=EDGE_CURVE('',#8466,#8467,#1500,.T.);
#10922=EDGE_CURVE('',#8466,#8468,#5048,.T.);
#10923=EDGE_CURVE('',#8469,#8468,#1501,.T.);
#10924=EDGE_CURVE('',#8467,#8469,#5049,.T.);
#10925=EDGE_CURVE('',#8470,#8470,#1502,.T.);
#10926=EDGE_CURVE('',#8470,#8471,#5050,.T.);
#10927=EDGE_CURVE('',#8471,#8471,#1503,.T.);
#10928=EDGE_CURVE('',#8472,#8473,#5051,.T.);
#10929=EDGE_CURVE('',#8473,#8474,#5052,.T.);
#10930=EDGE_CURVE('',#8474,#8475,#5053,.T.);
#10931=EDGE_CURVE('',#8475,#8476,#5054,.T.);
#10932=EDGE_CURVE('',#8476,#8477,#5055,.T.);
#10933=EDGE_CURVE('',#8477,#8478,#5056,.T.);
#10934=EDGE_CURVE('',#8478,#8479,#5057,.T.);
#10935=EDGE_CURVE('',#8479,#8480,#1504,.T.);
#10936=EDGE_CURVE('',#8480,#8481,#5058,.T.);
#10937=EDGE_CURVE('',#8481,#8482,#5059,.T.);
#10938=EDGE_CURVE('',#8482,#8483,#5060,.T.);
#10939=EDGE_CURVE('',#8483,#8484,#5061,.T.);
#10940=EDGE_CURVE('',#8484,#8485,#5062,.T.);
#10941=EDGE_CURVE('',#8485,#8472,#5063,.T.);
#10942=EDGE_CURVE('',#8486,#8487,#1505,.T.);
#10943=EDGE_CURVE('',#8486,#8488,#5064,.T.);
#10944=EDGE_CURVE('',#8489,#8488,#1506,.T.);
#10945=EDGE_CURVE('',#8487,#8489,#5065,.T.);
#10946=EDGE_CURVE('',#8490,#8491,#5066,.T.);
#10947=EDGE_CURVE('',#8490,#8492,#5067,.T.);
#10948=EDGE_CURVE('',#8493,#8492,#5068,.T.);
#10949=EDGE_CURVE('',#8494,#8493,#5069,.T.);
#10950=EDGE_CURVE('',#8494,#8495,#5070,.T.);
#10951=EDGE_CURVE('',#8496,#8495,#5071,.T.);
#10952=EDGE_CURVE('',#8497,#8496,#5072,.T.);
#10953=EDGE_CURVE('',#8498,#8497,#5073,.T.);
#10954=EDGE_CURVE('',#8499,#8498,#5074,.T.);
#10955=EDGE_CURVE('',#8500,#8499,#1507,.T.);
#10956=EDGE_CURVE('',#8501,#8500,#5075,.T.);
#10957=EDGE_CURVE('',#8502,#8501,#5076,.T.);
#10958=EDGE_CURVE('',#8503,#8502,#5077,.T.);
#10959=EDGE_CURVE('',#8491,#8503,#5078,.T.);
#10960=EDGE_CURVE('',#8504,#8504,#1508,.T.);
#10961=EDGE_CURVE('',#8505,#8506,#5079,.T.);
#10962=EDGE_CURVE('',#8507,#8505,#5080,.T.);
#10963=EDGE_CURVE('',#8508,#8507,#5081,.T.);
#10964=EDGE_CURVE('',#8509,#8508,#5082,.T.);
#10965=EDGE_CURVE('',#8510,#8509,#5083,.T.);
#10966=EDGE_CURVE('',#8506,#8510,#5084,.T.);
#10967=EDGE_CURVE('',#8511,#8489,#5085,.T.);
#10968=EDGE_CURVE('',#8511,#8512,#1509,.T.);
#10969=EDGE_CURVE('',#8512,#8513,#5086,.T.);
#10970=EDGE_CURVE('',#8513,#8490,#1510,.T.);
#10971=EDGE_CURVE('',#8475,#8491,#5087,.T.);
#10972=EDGE_CURVE('',#8474,#8514,#1511,.T.);
#10973=EDGE_CURVE('',#8515,#8514,#5088,.T.);
#10974=EDGE_CURVE('',#8515,#8516,#1512,.T.);
#10975=EDGE_CURVE('',#8487,#8516,#5089,.T.);
#10976=EDGE_CURVE('',#8476,#8503,#5090,.T.);
#10977=EDGE_CURVE('',#8477,#8502,#5091,.T.);
#10978=EDGE_CURVE('',#8478,#8501,#5092,.T.);
#10979=EDGE_CURVE('',#8479,#8500,#5093,.T.);
#10980=EDGE_CURVE('',#8480,#8499,#5094,.T.);
#10981=EDGE_CURVE('',#8481,#8498,#5095,.T.);
#10982=EDGE_CURVE('',#8482,#8497,#5096,.T.);
#10983=EDGE_CURVE('',#8483,#8496,#5097,.T.);
#10984=EDGE_CURVE('',#8495,#8517,#432,.T.);
#10985=EDGE_CURVE('',#8518,#8517,#5098,.T.);
#10986=EDGE_CURVE('',#8518,#8519,#433,.T.);
#10987=EDGE_CURVE('',#8468,#8519,#5099,.T.);
#10988=EDGE_CURVE('',#8520,#8466,#5100,.T.);
#10989=EDGE_CURVE('',#8520,#8521,#434,.T.);
#10990=EDGE_CURVE('',#8521,#8522,#5101,.T.);
#10991=EDGE_CURVE('',#8522,#8484,#435,.T.);
#10992=EDGE_CURVE('',#8523,#8524,#5102,.T.);
#10993=EDGE_CURVE('',#8524,#8494,#436,.T.);
#10994=EDGE_CURVE('',#8472,#8493,#5103,.T.);
#10995=EDGE_CURVE('',#8485,#8525,#437,.T.);
#10996=EDGE_CURVE('',#8526,#8525,#5104,.T.);
#10997=EDGE_CURVE('',#8526,#8527,#438,.T.);
#10998=EDGE_CURVE('',#8467,#8527,#5105,.T.);
#10999=EDGE_CURVE('',#8528,#8469,#5106,.T.);
#11000=EDGE_CURVE('',#8528,#8523,#439,.T.);
#11001=EDGE_CURVE('',#8529,#8530,#5107,.T.);
#11002=EDGE_CURVE('',#8529,#8531,#440,.T.);
#11003=EDGE_CURVE('',#8488,#8531,#5108,.T.);
#11004=EDGE_CURVE('',#8532,#8486,#5109,.T.);
#11005=EDGE_CURVE('',#8532,#8533,#441,.T.);
#11006=EDGE_CURVE('',#8533,#8534,#5110,.T.);
#11007=EDGE_CURVE('',#8534,#8473,#442,.T.);
#11008=EDGE_CURVE('',#8492,#8530,#443,.T.);
#11009=EDGE_CURVE('',#8527,#8520,#5111,.T.);
#11010=EDGE_CURVE('',#8525,#8522,#5112,.T.);
#11011=EDGE_CURVE('',#8521,#8526,#5113,.T.);
#11012=EDGE_CURVE('',#8523,#8518,#5114,.T.);
#11013=EDGE_CURVE('',#8517,#8524,#5115,.T.);
#11014=EDGE_CURVE('',#8519,#8528,#5116,.T.);
#11015=EDGE_CURVE('',#8531,#8511,#5117,.T.);
#11016=EDGE_CURVE('',#8512,#8529,#5118,.T.);
#11017=EDGE_CURVE('',#8530,#8513,#5119,.T.);
#11018=EDGE_CURVE('',#8533,#8515,#5120,.T.);
#11019=EDGE_CURVE('',#8514,#8534,#5121,.T.);
#11020=EDGE_CURVE('',#8516,#8532,#5122,.T.);
#11021=EDGE_CURVE('',#8505,#8535,#5123,.T.);
#11022=EDGE_CURVE('',#8535,#8536,#5124,.T.);
#11023=EDGE_CURVE('',#8507,#8536,#5125,.T.);
#11024=EDGE_CURVE('',#8506,#8537,#5126,.T.);
#11025=EDGE_CURVE('',#8537,#8535,#5127,.T.);
#11026=EDGE_CURVE('',#8510,#8538,#5128,.T.);
#11027=EDGE_CURVE('',#8538,#8537,#5129,.T.);
#11028=EDGE_CURVE('',#8509,#8539,#5130,.T.);
#11029=EDGE_CURVE('',#8539,#8538,#5131,.T.);
#11030=EDGE_CURVE('',#8508,#8540,#5132,.T.);
#11031=EDGE_CURVE('',#8540,#8539,#5133,.T.);
#11032=EDGE_CURVE('',#8536,#8540,#5134,.T.);
#11033=EDGE_CURVE('',#8541,#8542,#5135,.T.);
#11034=EDGE_CURVE('',#8542,#8543,#5136,.T.);
#11035=EDGE_CURVE('',#8543,#8544,#5137,.T.);
#11036=EDGE_CURVE('',#8544,#8545,#5138,.T.);
#11037=EDGE_CURVE('',#8545,#8546,#5139,.T.);
#11038=EDGE_CURVE('',#8546,#8541,#5140,.T.);
#11039=EDGE_CURVE('',#8535,#8545,#444,.T.);
#11040=EDGE_CURVE('',#8546,#8537,#445,.T.);
#11041=EDGE_CURVE('',#8541,#8538,#446,.T.);
#11042=EDGE_CURVE('',#8536,#8544,#447,.T.);
#11043=EDGE_CURVE('',#8542,#8539,#448,.T.);
#11044=EDGE_CURVE('',#8540,#8543,#449,.T.);
#11045=EDGE_CURVE('',#8458,#8504,#5141,.T.);
#11046=EDGE_CURVE('',#8547,#8547,#1513,.T.);
#11047=EDGE_CURVE('',#8547,#8548,#5142,.T.);
#11048=EDGE_CURVE('',#8548,#8548,#1514,.T.);
#11049=EDGE_CURVE('',#8549,#8550,#5143,.T.);
#11050=EDGE_CURVE('',#8551,#8550,#5144,.T.);
#11051=EDGE_CURVE('',#8552,#8551,#5145,.T.);
#11052=EDGE_CURVE('',#8552,#8549,#5146,.T.);
#11053=EDGE_CURVE('',#8553,#8552,#1515,.T.);
#11054=EDGE_CURVE('',#8553,#8554,#5147,.T.);
#11055=EDGE_CURVE('',#8554,#8549,#1516,.T.);
#11056=EDGE_CURVE('',#8555,#8554,#5148,.T.);
#11057=EDGE_CURVE('',#8556,#8553,#5149,.T.);
#11058=EDGE_CURVE('',#8556,#8555,#5150,.T.);
#11059=EDGE_CURVE('',#8557,#8555,#5151,.T.);
#11060=EDGE_CURVE('',#8558,#8556,#5152,.T.);
#11061=EDGE_CURVE('',#8558,#8557,#5153,.T.);
#11062=EDGE_CURVE('',#8559,#8557,#5154,.T.);
#11063=EDGE_CURVE('',#8560,#8558,#5155,.T.);
#11064=EDGE_CURVE('',#8560,#8559,#5156,.T.);
#11065=EDGE_CURVE('',#8561,#8559,#5157,.T.);
#11066=EDGE_CURVE('',#8562,#8560,#5158,.T.);
#11067=EDGE_CURVE('',#8562,#8561,#5159,.T.);
#11068=EDGE_CURVE('',#8563,#8561,#5160,.T.);
#11069=EDGE_CURVE('',#8564,#8562,#5161,.T.);
#11070=EDGE_CURVE('',#8564,#8563,#5162,.T.);
#11071=EDGE_CURVE('',#8565,#8563,#5163,.T.);
#11072=EDGE_CURVE('',#8566,#8564,#5164,.T.);
#11073=EDGE_CURVE('',#8566,#8565,#5165,.T.);
#11074=EDGE_CURVE('',#8567,#8565,#5166,.T.);
#11075=EDGE_CURVE('',#8568,#8566,#5167,.T.);
#11076=EDGE_CURVE('',#8568,#8567,#5168,.T.);
#11077=EDGE_CURVE('',#8569,#8567,#5169,.T.);
#11078=EDGE_CURVE('',#8570,#8568,#5170,.T.);
#11079=EDGE_CURVE('',#8570,#8569,#5171,.T.);
#11080=EDGE_CURVE('',#8571,#8569,#5172,.T.);
#11081=EDGE_CURVE('',#8572,#8570,#5173,.T.);
#11082=EDGE_CURVE('',#8572,#8571,#5174,.T.);
#11083=EDGE_CURVE('',#8573,#8571,#5175,.T.);
#11084=EDGE_CURVE('',#8574,#8572,#5176,.T.);
#11085=EDGE_CURVE('',#8574,#8573,#5177,.T.);
#11086=EDGE_CURVE('',#8575,#8573,#5178,.T.);
#11087=EDGE_CURVE('',#8576,#8574,#5179,.T.);
#11088=EDGE_CURVE('',#8576,#8575,#5180,.T.);
#11089=EDGE_CURVE('',#8577,#8575,#5181,.T.);
#11090=EDGE_CURVE('',#8578,#8576,#5182,.T.);
#11091=EDGE_CURVE('',#8578,#8577,#5183,.T.);
#11092=EDGE_CURVE('',#8579,#8577,#5184,.T.);
#11093=EDGE_CURVE('',#8580,#8578,#5185,.T.);
#11094=EDGE_CURVE('',#8580,#8579,#5186,.T.);
#11095=EDGE_CURVE('',#8581,#8579,#5187,.T.);
#11096=EDGE_CURVE('',#8582,#8580,#5188,.T.);
#11097=EDGE_CURVE('',#8582,#8581,#5189,.T.);
#11098=EDGE_CURVE('',#8583,#8581,#5190,.T.);
#11099=EDGE_CURVE('',#8584,#8582,#5191,.T.);
#11100=EDGE_CURVE('',#8584,#8583,#5192,.T.);
#11101=EDGE_CURVE('',#8585,#8583,#5193,.T.);
#11102=EDGE_CURVE('',#8586,#8584,#5194,.T.);
#11103=EDGE_CURVE('',#8586,#8585,#5195,.T.);
#11104=EDGE_CURVE('',#8587,#8585,#5196,.T.);
#11105=EDGE_CURVE('',#8588,#8586,#5197,.T.);
#11106=EDGE_CURVE('',#8588,#8587,#5198,.T.);
#11107=EDGE_CURVE('',#8589,#8587,#5199,.T.);
#11108=EDGE_CURVE('',#8590,#8588,#5200,.T.);
#11109=EDGE_CURVE('',#8590,#8589,#5201,.T.);
#11110=EDGE_CURVE('',#8591,#8589,#5202,.T.);
#11111=EDGE_CURVE('',#8592,#8590,#5203,.T.);
#11112=EDGE_CURVE('',#8592,#8591,#5204,.T.);
#11113=EDGE_CURVE('',#8593,#8591,#5205,.T.);
#11114=EDGE_CURVE('',#8594,#8592,#5206,.T.);
#11115=EDGE_CURVE('',#8594,#8593,#5207,.T.);
#11116=EDGE_CURVE('',#8595,#8593,#5208,.T.);
#11117=EDGE_CURVE('',#8596,#8594,#5209,.T.);
#11118=EDGE_CURVE('',#8596,#8595,#5210,.T.);
#11119=EDGE_CURVE('',#8597,#8595,#5211,.T.);
#11120=EDGE_CURVE('',#8598,#8596,#5212,.T.);
#11121=EDGE_CURVE('',#8598,#8597,#5213,.T.);
#11122=EDGE_CURVE('',#8599,#8597,#5214,.T.);
#11123=EDGE_CURVE('',#8600,#8598,#5215,.T.);
#11124=EDGE_CURVE('',#8600,#8599,#5216,.T.);
#11125=EDGE_CURVE('',#8601,#8599,#5217,.T.);
#11126=EDGE_CURVE('',#8602,#8600,#5218,.T.);
#11127=EDGE_CURVE('',#8602,#8601,#5219,.T.);
#11128=EDGE_CURVE('',#8603,#8601,#5220,.T.);
#11129=EDGE_CURVE('',#8604,#8602,#5221,.T.);
#11130=EDGE_CURVE('',#8604,#8603,#5222,.T.);
#11131=EDGE_CURVE('',#8605,#8603,#5223,.T.);
#11132=EDGE_CURVE('',#8606,#8604,#5224,.T.);
#11133=EDGE_CURVE('',#8606,#8605,#5225,.T.);
#11134=EDGE_CURVE('',#8607,#8605,#5226,.T.);
#11135=EDGE_CURVE('',#8608,#8606,#5227,.T.);
#11136=EDGE_CURVE('',#8608,#8607,#5228,.T.);
#11137=EDGE_CURVE('',#8609,#8607,#5229,.T.);
#11138=EDGE_CURVE('',#8610,#8608,#5230,.T.);
#11139=EDGE_CURVE('',#8610,#8609,#5231,.T.);
#11140=EDGE_CURVE('',#8611,#8609,#5232,.T.);
#11141=EDGE_CURVE('',#8612,#8610,#5233,.T.);
#11142=EDGE_CURVE('',#8612,#8611,#5234,.T.);
#11143=EDGE_CURVE('',#8613,#8611,#5235,.T.);
#11144=EDGE_CURVE('',#8614,#8612,#5236,.T.);
#11145=EDGE_CURVE('',#8614,#8613,#5237,.T.);
#11146=EDGE_CURVE('',#8615,#8613,#5238,.T.);
#11147=EDGE_CURVE('',#8616,#8614,#5239,.T.);
#11148=EDGE_CURVE('',#8616,#8615,#5240,.T.);
#11149=EDGE_CURVE('',#8617,#8615,#5241,.T.);
#11150=EDGE_CURVE('',#8618,#8616,#5242,.T.);
#11151=EDGE_CURVE('',#8618,#8617,#5243,.T.);
#11152=EDGE_CURVE('',#8619,#8617,#5244,.T.);
#11153=EDGE_CURVE('',#8620,#8618,#5245,.T.);
#11154=EDGE_CURVE('',#8620,#8619,#5246,.T.);
#11155=EDGE_CURVE('',#8621,#8619,#5247,.T.);
#11156=EDGE_CURVE('',#8622,#8620,#5248,.T.);
#11157=EDGE_CURVE('',#8622,#8621,#5249,.T.);
#11158=EDGE_CURVE('',#8623,#8621,#5250,.T.);
#11159=EDGE_CURVE('',#8624,#8622,#5251,.T.);
#11160=EDGE_CURVE('',#8624,#8623,#5252,.T.);
#11161=EDGE_CURVE('',#8625,#8623,#5253,.T.);
#11162=EDGE_CURVE('',#8626,#8624,#5254,.T.);
#11163=EDGE_CURVE('',#8626,#8625,#5255,.T.);
#11164=EDGE_CURVE('',#8627,#8625,#5256,.T.);
#11165=EDGE_CURVE('',#8628,#8626,#5257,.T.);
#11166=EDGE_CURVE('',#8628,#8627,#5258,.T.);
#11167=EDGE_CURVE('',#8629,#8627,#5259,.T.);
#11168=EDGE_CURVE('',#8630,#8628,#5260,.T.);
#11169=EDGE_CURVE('',#8630,#8629,#5261,.T.);
#11170=EDGE_CURVE('',#8631,#8629,#1517,.T.);
#11171=EDGE_CURVE('',#8632,#8630,#1518,.T.);
#11172=EDGE_CURVE('',#8632,#8631,#5262,.T.);
#11173=EDGE_CURVE('',#8633,#8631,#5263,.T.);
#11174=EDGE_CURVE('',#8634,#8632,#5264,.T.);
#11175=EDGE_CURVE('',#8634,#8633,#5265,.T.);
#11176=EDGE_CURVE('',#8550,#8633,#5266,.T.);
#11177=EDGE_CURVE('',#8551,#8634,#5267,.T.);
#15432=ORIENTED_EDGE('',*,*,#10768,.T.);
#15433=ORIENTED_EDGE('',*,*,#10769,.T.);
#15434=ORIENTED_EDGE('',*,*,#10770,.F.);
#15435=ORIENTED_EDGE('',*,*,#10771,.F.);
#15436=ORIENTED_EDGE('',*,*,#10772,.T.);
#15437=ORIENTED_EDGE('',*,*,#10769,.F.);
#15438=ORIENTED_EDGE('',*,*,#10772,.F.);
#15439=ORIENTED_EDGE('',*,*,#10768,.F.);
#15440=ORIENTED_EDGE('',*,*,#10773,.T.);
#15441=ORIENTED_EDGE('',*,*,#10770,.T.);
#15442=ORIENTED_EDGE('',*,*,#10771,.T.);
#15443=ORIENTED_EDGE('',*,*,#10773,.F.);
#15444=ORIENTED_EDGE('',*,*,#10774,.T.);
#15445=ORIENTED_EDGE('',*,*,#10775,.T.);
#15446=ORIENTED_EDGE('',*,*,#10776,.T.);
#15447=ORIENTED_EDGE('',*,*,#10777,.F.);
#15448=ORIENTED_EDGE('',*,*,#10778,.T.);
#15449=ORIENTED_EDGE('',*,*,#10779,.T.);
#15450=ORIENTED_EDGE('',*,*,#10774,.F.);
#15451=ORIENTED_EDGE('',*,*,#10780,.F.);
#15452=ORIENTED_EDGE('',*,*,#10781,.T.);
#15453=ORIENTED_EDGE('',*,*,#10782,.T.);
#15454=ORIENTED_EDGE('',*,*,#10778,.F.);
#15455=ORIENTED_EDGE('',*,*,#10783,.F.);
#15456=ORIENTED_EDGE('',*,*,#10784,.T.);
#15457=ORIENTED_EDGE('',*,*,#10785,.T.);
#15458=ORIENTED_EDGE('',*,*,#10781,.F.);
#15459=ORIENTED_EDGE('',*,*,#10786,.F.);
#15460=ORIENTED_EDGE('',*,*,#10787,.T.);
#15461=ORIENTED_EDGE('',*,*,#10788,.T.);
#15462=ORIENTED_EDGE('',*,*,#10784,.F.);
#15463=ORIENTED_EDGE('',*,*,#10789,.F.);
#15464=ORIENTED_EDGE('',*,*,#10790,.T.);
#15465=ORIENTED_EDGE('',*,*,#10791,.T.);
#15466=ORIENTED_EDGE('',*,*,#10787,.F.);
#15467=ORIENTED_EDGE('',*,*,#10792,.F.);
#15468=ORIENTED_EDGE('',*,*,#10793,.T.);
#15469=ORIENTED_EDGE('',*,*,#10794,.T.);
#15470=ORIENTED_EDGE('',*,*,#10790,.F.);
#15471=ORIENTED_EDGE('',*,*,#10795,.F.);
#15472=ORIENTED_EDGE('',*,*,#10796,.T.);
#15473=ORIENTED_EDGE('',*,*,#10797,.T.);
#15474=ORIENTED_EDGE('',*,*,#10793,.F.);
#15475=ORIENTED_EDGE('',*,*,#10798,.F.);
#15476=ORIENTED_EDGE('',*,*,#10799,.T.);
#15477=ORIENTED_EDGE('',*,*,#10800,.T.);
#15478=ORIENTED_EDGE('',*,*,#10796,.F.);
#15479=ORIENTED_EDGE('',*,*,#10801,.F.);
#15480=ORIENTED_EDGE('',*,*,#10802,.T.);
#15481=ORIENTED_EDGE('',*,*,#10803,.T.);
#15482=ORIENTED_EDGE('',*,*,#10799,.F.);
#15483=ORIENTED_EDGE('',*,*,#10804,.F.);
#15484=ORIENTED_EDGE('',*,*,#10805,.T.);
#15485=ORIENTED_EDGE('',*,*,#10806,.T.);
#15486=ORIENTED_EDGE('',*,*,#10802,.F.);
#15487=ORIENTED_EDGE('',*,*,#10807,.F.);
#15488=ORIENTED_EDGE('',*,*,#10808,.T.);
#15489=ORIENTED_EDGE('',*,*,#10809,.T.);
#15490=ORIENTED_EDGE('',*,*,#10805,.F.);
#15491=ORIENTED_EDGE('',*,*,#10810,.F.);
#15492=ORIENTED_EDGE('',*,*,#10811,.T.);
#15493=ORIENTED_EDGE('',*,*,#10812,.T.);
#15494=ORIENTED_EDGE('',*,*,#10808,.F.);
#15495=ORIENTED_EDGE('',*,*,#10813,.F.);
#15496=ORIENTED_EDGE('',*,*,#10814,.F.);
#15497=ORIENTED_EDGE('',*,*,#10815,.T.);
#15498=ORIENTED_EDGE('',*,*,#10816,.T.);
#15499=ORIENTED_EDGE('',*,*,#10817,.T.);
#15500=ORIENTED_EDGE('',*,*,#10818,.T.);
#15501=ORIENTED_EDGE('',*,*,#10819,.T.);
#15502=ORIENTED_EDGE('',*,*,#10820,.F.);
#15503=ORIENTED_EDGE('',*,*,#10821,.T.);
#15504=ORIENTED_EDGE('',*,*,#10822,.T.);
#15505=ORIENTED_EDGE('',*,*,#10817,.F.);
#15506=ORIENTED_EDGE('',*,*,#10823,.F.);
#15507=ORIENTED_EDGE('',*,*,#10824,.T.);
#15508=ORIENTED_EDGE('',*,*,#10825,.T.);
#15509=ORIENTED_EDGE('',*,*,#10821,.F.);
#15510=ORIENTED_EDGE('',*,*,#10826,.F.);
#15511=ORIENTED_EDGE('',*,*,#10827,.T.);
#15512=ORIENTED_EDGE('',*,*,#10828,.T.);
#15513=ORIENTED_EDGE('',*,*,#10824,.F.);
#15514=ORIENTED_EDGE('',*,*,#10829,.F.);
#15515=ORIENTED_EDGE('',*,*,#10830,.T.);
#15516=ORIENTED_EDGE('',*,*,#10831,.T.);
#15517=ORIENTED_EDGE('',*,*,#10827,.F.);
#15518=ORIENTED_EDGE('',*,*,#10832,.F.);
#15519=ORIENTED_EDGE('',*,*,#10833,.T.);
#15520=ORIENTED_EDGE('',*,*,#10834,.T.);
#15521=ORIENTED_EDGE('',*,*,#10830,.F.);
#15522=ORIENTED_EDGE('',*,*,#10835,.F.);
#15523=ORIENTED_EDGE('',*,*,#10836,.T.);
#15524=ORIENTED_EDGE('',*,*,#10837,.T.);
#15525=ORIENTED_EDGE('',*,*,#10833,.F.);
#15526=ORIENTED_EDGE('',*,*,#10838,.F.);
#15527=ORIENTED_EDGE('',*,*,#10839,.T.);
#15528=ORIENTED_EDGE('',*,*,#10840,.T.);
#15529=ORIENTED_EDGE('',*,*,#10836,.F.);
#15530=ORIENTED_EDGE('',*,*,#10841,.F.);
#15531=ORIENTED_EDGE('',*,*,#10842,.T.);
#15532=ORIENTED_EDGE('',*,*,#10843,.T.);
#15533=ORIENTED_EDGE('',*,*,#10839,.F.);
#15534=ORIENTED_EDGE('',*,*,#10844,.F.);
#15535=ORIENTED_EDGE('',*,*,#10845,.T.);
#15536=ORIENTED_EDGE('',*,*,#10846,.T.);
#15537=ORIENTED_EDGE('',*,*,#10842,.F.);
#15538=ORIENTED_EDGE('',*,*,#10847,.F.);
#15539=ORIENTED_EDGE('',*,*,#10848,.T.);
#15540=ORIENTED_EDGE('',*,*,#10849,.T.);
#15541=ORIENTED_EDGE('',*,*,#10845,.F.);
#15542=ORIENTED_EDGE('',*,*,#10850,.F.);
#15543=ORIENTED_EDGE('',*,*,#10851,.T.);
#15544=ORIENTED_EDGE('',*,*,#10852,.T.);
#15545=ORIENTED_EDGE('',*,*,#10848,.F.);
#15546=ORIENTED_EDGE('',*,*,#10853,.F.);
#15547=ORIENTED_EDGE('',*,*,#10854,.T.);
#15548=ORIENTED_EDGE('',*,*,#10855,.T.);
#15549=ORIENTED_EDGE('',*,*,#10851,.F.);
#15550=ORIENTED_EDGE('',*,*,#10856,.F.);
#15551=ORIENTED_EDGE('',*,*,#10857,.F.);
#15552=ORIENTED_EDGE('',*,*,#10858,.F.);
#15553=ORIENTED_EDGE('',*,*,#10859,.T.);
#15554=ORIENTED_EDGE('',*,*,#10860,.T.);
#15555=ORIENTED_EDGE('',*,*,#10861,.F.);
#15556=ORIENTED_EDGE('',*,*,#10862,.T.);
#15557=ORIENTED_EDGE('',*,*,#10863,.T.);
#15558=ORIENTED_EDGE('',*,*,#10862,.F.);
#15559=ORIENTED_EDGE('',*,*,#10864,.T.);
#15560=ORIENTED_EDGE('',*,*,#10865,.T.);
#15561=ORIENTED_EDGE('',*,*,#10866,.T.);
#15562=ORIENTED_EDGE('',*,*,#10865,.F.);
#15563=ORIENTED_EDGE('',*,*,#10867,.T.);
#15564=ORIENTED_EDGE('',*,*,#10868,.T.);
#15565=ORIENTED_EDGE('',*,*,#10869,.T.);
#15566=ORIENTED_EDGE('',*,*,#10868,.F.);
#15567=ORIENTED_EDGE('',*,*,#10870,.F.);
#15568=ORIENTED_EDGE('',*,*,#10871,.T.);
#15569=ORIENTED_EDGE('',*,*,#10872,.F.);
#15570=ORIENTED_EDGE('',*,*,#10873,.F.);
#15571=ORIENTED_EDGE('',*,*,#10871,.F.);
#15572=ORIENTED_EDGE('',*,*,#10874,.F.);
#15573=ORIENTED_EDGE('',*,*,#10875,.F.);
#15574=ORIENTED_EDGE('',*,*,#10876,.T.);
#15575=ORIENTED_EDGE('',*,*,#10877,.F.);
#15576=ORIENTED_EDGE('',*,*,#10876,.F.);
#15577=ORIENTED_EDGE('',*,*,#10878,.F.);
#15578=ORIENTED_EDGE('',*,*,#10879,.F.);
#15579=ORIENTED_EDGE('',*,*,#10880,.T.);
#15580=ORIENTED_EDGE('',*,*,#10881,.F.);
#15581=ORIENTED_EDGE('',*,*,#10880,.F.);
#15582=ORIENTED_EDGE('',*,*,#10882,.F.);
#15583=ORIENTED_EDGE('',*,*,#10883,.T.);
#15584=ORIENTED_EDGE('',*,*,#10884,.F.);
#15585=ORIENTED_EDGE('',*,*,#10885,.F.);
#15586=ORIENTED_EDGE('',*,*,#10883,.F.);
#15587=ORIENTED_EDGE('',*,*,#10878,.T.);
#15588=ORIENTED_EDGE('',*,*,#10879,.T.);
#15589=ORIENTED_EDGE('',*,*,#10886,.T.);
#15590=ORIENTED_EDGE('',*,*,#10884,.T.);
#15591=ORIENTED_EDGE('',*,*,#10885,.T.);
#15592=ORIENTED_EDGE('',*,*,#10886,.F.);
#15593=ORIENTED_EDGE('',*,*,#10874,.T.);
#15594=ORIENTED_EDGE('',*,*,#10875,.T.);
#15595=ORIENTED_EDGE('',*,*,#10887,.T.);
#15596=ORIENTED_EDGE('',*,*,#10872,.T.);
#15597=ORIENTED_EDGE('',*,*,#10873,.T.);
#15598=ORIENTED_EDGE('',*,*,#10887,.F.);
#15599=ORIENTED_EDGE('',*,*,#10877,.T.);
#15600=ORIENTED_EDGE('',*,*,#10882,.T.);
#15601=ORIENTED_EDGE('',*,*,#10870,.T.);
#15602=ORIENTED_EDGE('',*,*,#10888,.F.);
#15603=ORIENTED_EDGE('',*,*,#10881,.T.);
#15604=ORIENTED_EDGE('',*,*,#10889,.T.);
#15605=ORIENTED_EDGE('',*,*,#10890,.T.);
#15606=ORIENTED_EDGE('',*,*,#10891,.T.);
#15607=ORIENTED_EDGE('',*,*,#10892,.T.);
#15608=ORIENTED_EDGE('',*,*,#10893,.T.);
#15609=ORIENTED_EDGE('',*,*,#10894,.T.);
#15610=ORIENTED_EDGE('',*,*,#10858,.T.);
#15611=ORIENTED_EDGE('',*,*,#10895,.T.);
#15612=ORIENTED_EDGE('',*,*,#10856,.T.);
#15613=ORIENTED_EDGE('',*,*,#10853,.T.);
#15614=ORIENTED_EDGE('',*,*,#10850,.T.);
#15615=ORIENTED_EDGE('',*,*,#10847,.T.);
#15616=ORIENTED_EDGE('',*,*,#10844,.T.);
#15617=ORIENTED_EDGE('',*,*,#10841,.T.);
#15618=ORIENTED_EDGE('',*,*,#10838,.T.);
#15619=ORIENTED_EDGE('',*,*,#10835,.T.);
#15620=ORIENTED_EDGE('',*,*,#10832,.T.);
#15621=ORIENTED_EDGE('',*,*,#10829,.T.);
#15622=ORIENTED_EDGE('',*,*,#10826,.T.);
#15623=ORIENTED_EDGE('',*,*,#10823,.T.);
#15624=ORIENTED_EDGE('',*,*,#10820,.T.);
#15625=ORIENTED_EDGE('',*,*,#10896,.T.);
#15626=ORIENTED_EDGE('',*,*,#10779,.F.);
#15627=ORIENTED_EDGE('',*,*,#10782,.F.);
#15628=ORIENTED_EDGE('',*,*,#10785,.F.);
#15629=ORIENTED_EDGE('',*,*,#10788,.F.);
#15630=ORIENTED_EDGE('',*,*,#10791,.F.);
#15631=ORIENTED_EDGE('',*,*,#10794,.F.);
#15632=ORIENTED_EDGE('',*,*,#10797,.F.);
#15633=ORIENTED_EDGE('',*,*,#10800,.F.);
#15634=ORIENTED_EDGE('',*,*,#10803,.F.);
#15635=ORIENTED_EDGE('',*,*,#10806,.F.);
#15636=ORIENTED_EDGE('',*,*,#10809,.F.);
#15637=ORIENTED_EDGE('',*,*,#10812,.F.);
#15638=ORIENTED_EDGE('',*,*,#10897,.F.);
#15639=ORIENTED_EDGE('',*,*,#10816,.F.);
#15640=ORIENTED_EDGE('',*,*,#10890,.F.);
#15641=ORIENTED_EDGE('',*,*,#10857,.T.);
#15642=ORIENTED_EDGE('',*,*,#10898,.T.);
#15643=ORIENTED_EDGE('',*,*,#10854,.F.);
#15644=ORIENTED_EDGE('',*,*,#10895,.F.);
#15645=ORIENTED_EDGE('',*,*,#10899,.T.);
#15646=ORIENTED_EDGE('',*,*,#10900,.T.);
#15647=ORIENTED_EDGE('',*,*,#10813,.T.);
#15648=ORIENTED_EDGE('',*,*,#10810,.T.);
#15649=ORIENTED_EDGE('',*,*,#10807,.T.);
#15650=ORIENTED_EDGE('',*,*,#10804,.T.);
#15651=ORIENTED_EDGE('',*,*,#10801,.T.);
#15652=ORIENTED_EDGE('',*,*,#10798,.T.);
#15653=ORIENTED_EDGE('',*,*,#10795,.T.);
#15654=ORIENTED_EDGE('',*,*,#10792,.T.);
#15655=ORIENTED_EDGE('',*,*,#10789,.T.);
#15656=ORIENTED_EDGE('',*,*,#10786,.T.);
#15657=ORIENTED_EDGE('',*,*,#10783,.T.);
#15658=ORIENTED_EDGE('',*,*,#10780,.T.);
#15659=ORIENTED_EDGE('',*,*,#10777,.T.);
#15660=ORIENTED_EDGE('',*,*,#10901,.T.);
#15661=ORIENTED_EDGE('',*,*,#10902,.T.);
#15662=ORIENTED_EDGE('',*,*,#10818,.F.);
#15663=ORIENTED_EDGE('',*,*,#10822,.F.);
#15664=ORIENTED_EDGE('',*,*,#10825,.F.);
#15665=ORIENTED_EDGE('',*,*,#10828,.F.);
#15666=ORIENTED_EDGE('',*,*,#10831,.F.);
#15667=ORIENTED_EDGE('',*,*,#10834,.F.);
#15668=ORIENTED_EDGE('',*,*,#10837,.F.);
#15669=ORIENTED_EDGE('',*,*,#10840,.F.);
#15670=ORIENTED_EDGE('',*,*,#10843,.F.);
#15671=ORIENTED_EDGE('',*,*,#10846,.F.);
#15672=ORIENTED_EDGE('',*,*,#10849,.F.);
#15673=ORIENTED_EDGE('',*,*,#10852,.F.);
#15674=ORIENTED_EDGE('',*,*,#10855,.F.);
#15675=ORIENTED_EDGE('',*,*,#10898,.F.);
#15676=ORIENTED_EDGE('',*,*,#10860,.F.);
#15677=ORIENTED_EDGE('',*,*,#10902,.F.);
#15678=ORIENTED_EDGE('',*,*,#10903,.F.);
#15679=ORIENTED_EDGE('',*,*,#10775,.F.);
#15680=ORIENTED_EDGE('',*,*,#10896,.F.);
#15681=ORIENTED_EDGE('',*,*,#10819,.F.);
#15682=ORIENTED_EDGE('',*,*,#10899,.F.);
#15683=ORIENTED_EDGE('',*,*,#10859,.F.);
#15684=ORIENTED_EDGE('',*,*,#10894,.F.);
#15685=ORIENTED_EDGE('',*,*,#10893,.F.);
#15686=ORIENTED_EDGE('',*,*,#10901,.F.);
#15687=ORIENTED_EDGE('',*,*,#10904,.T.);
#15688=ORIENTED_EDGE('',*,*,#10903,.T.);
#15689=ORIENTED_EDGE('',*,*,#10891,.F.);
#15690=ORIENTED_EDGE('',*,*,#10815,.F.);
#15691=ORIENTED_EDGE('',*,*,#10892,.F.);
#15692=ORIENTED_EDGE('',*,*,#10905,.T.);
#15693=ORIENTED_EDGE('',*,*,#10906,.F.);
#15694=ORIENTED_EDGE('',*,*,#10905,.F.);
#15695=ORIENTED_EDGE('',*,*,#10776,.F.);
#15696=ORIENTED_EDGE('',*,*,#10907,.T.);
#15697=ORIENTED_EDGE('',*,*,#10889,.F.);
#15698=ORIENTED_EDGE('',*,*,#10907,.F.);
#15699=ORIENTED_EDGE('',*,*,#10904,.F.);
#15700=ORIENTED_EDGE('',*,*,#10908,.F.);
#15701=ORIENTED_EDGE('',*,*,#10909,.F.);
#15702=ORIENTED_EDGE('',*,*,#10910,.T.);
#15703=ORIENTED_EDGE('',*,*,#10911,.F.);
#15704=ORIENTED_EDGE('',*,*,#10910,.F.);
#15705=ORIENTED_EDGE('',*,*,#10911,.T.);
#15706=ORIENTED_EDGE('',*,*,#10906,.T.);
#15707=ORIENTED_EDGE('',*,*,#10814,.T.);
#15708=ORIENTED_EDGE('',*,*,#10897,.T.);
#15709=ORIENTED_EDGE('',*,*,#10811,.F.);
#15710=ORIENTED_EDGE('',*,*,#10900,.F.);
#15711=ORIENTED_EDGE('',*,*,#10866,.F.);
#15712=ORIENTED_EDGE('',*,*,#10912,.F.);
#15713=ORIENTED_EDGE('',*,*,#10913,.T.);
#15714=ORIENTED_EDGE('',*,*,#10914,.F.);
#15715=ORIENTED_EDGE('',*,*,#10913,.F.);
#15716=ORIENTED_EDGE('',*,*,#10915,.F.);
#15717=ORIENTED_EDGE('',*,*,#10916,.T.);
#15718=ORIENTED_EDGE('',*,*,#10917,.F.);
#15719=ORIENTED_EDGE('',*,*,#10916,.F.);
#15720=ORIENTED_EDGE('',*,*,#10917,.T.);
#15721=ORIENTED_EDGE('',*,*,#10918,.T.);
#15722=ORIENTED_EDGE('',*,*,#10912,.T.);
#15723=ORIENTED_EDGE('',*,*,#10918,.F.);
#15724=ORIENTED_EDGE('',*,*,#10919,.T.);
#15725=ORIENTED_EDGE('',*,*,#10920,.T.);
#15726=ORIENTED_EDGE('',*,*,#10888,.T.);
#15727=ORIENTED_EDGE('',*,*,#10920,.F.);
#15728=ORIENTED_EDGE('',*,*,#10921,.F.);
#15729=ORIENTED_EDGE('',*,*,#10922,.T.);
#15730=ORIENTED_EDGE('',*,*,#10923,.F.);
#15731=ORIENTED_EDGE('',*,*,#10924,.F.);
#15732=ORIENTED_EDGE('',*,*,#10925,.T.);
#15733=ORIENTED_EDGE('',*,*,#10926,.T.);
#15734=ORIENTED_EDGE('',*,*,#10927,.T.);
#15735=ORIENTED_EDGE('',*,*,#10926,.F.);
#15736=ORIENTED_EDGE('',*,*,#10928,.T.);
#15737=ORIENTED_EDGE('',*,*,#10929,.T.);
#15738=ORIENTED_EDGE('',*,*,#10930,.T.);
#15739=ORIENTED_EDGE('',*,*,#10931,.T.);
#15740=ORIENTED_EDGE('',*,*,#10932,.T.);
#15741=ORIENTED_EDGE('',*,*,#10933,.T.);
#15742=ORIENTED_EDGE('',*,*,#10934,.T.);
#15743=ORIENTED_EDGE('',*,*,#10935,.T.);
#15744=ORIENTED_EDGE('',*,*,#10936,.T.);
#15745=ORIENTED_EDGE('',*,*,#10937,.T.);
#15746=ORIENTED_EDGE('',*,*,#10938,.T.);
#15747=ORIENTED_EDGE('',*,*,#10939,.T.);
#15748=ORIENTED_EDGE('',*,*,#10940,.T.);
#15749=ORIENTED_EDGE('',*,*,#10941,.T.);
#15750=ORIENTED_EDGE('',*,*,#10919,.F.);
#15751=ORIENTED_EDGE('',*,*,#10927,.F.);
#15752=ORIENTED_EDGE('',*,*,#10942,.F.);
#15753=ORIENTED_EDGE('',*,*,#10943,.T.);
#15754=ORIENTED_EDGE('',*,*,#10944,.F.);
#15755=ORIENTED_EDGE('',*,*,#10945,.F.);
#15756=ORIENTED_EDGE('',*,*,#10946,.F.);
#15757=ORIENTED_EDGE('',*,*,#10947,.T.);
#15758=ORIENTED_EDGE('',*,*,#10948,.F.);
#15759=ORIENTED_EDGE('',*,*,#10949,.F.);
#15760=ORIENTED_EDGE('',*,*,#10950,.T.);
#15761=ORIENTED_EDGE('',*,*,#10951,.F.);
#15762=ORIENTED_EDGE('',*,*,#10952,.F.);
#15763=ORIENTED_EDGE('',*,*,#10953,.F.);
#15764=ORIENTED_EDGE('',*,*,#10954,.F.);
#15765=ORIENTED_EDGE('',*,*,#10955,.F.);
#15766=ORIENTED_EDGE('',*,*,#10956,.F.);
#15767=ORIENTED_EDGE('',*,*,#10957,.F.);
#15768=ORIENTED_EDGE('',*,*,#10958,.F.);
#15769=ORIENTED_EDGE('',*,*,#10959,.F.);
#15770=ORIENTED_EDGE('',*,*,#10960,.T.);
#15771=ORIENTED_EDGE('',*,*,#10961,.F.);
#15772=ORIENTED_EDGE('',*,*,#10962,.F.);
#15773=ORIENTED_EDGE('',*,*,#10963,.F.);
#15774=ORIENTED_EDGE('',*,*,#10964,.F.);
#15775=ORIENTED_EDGE('',*,*,#10965,.F.);
#15776=ORIENTED_EDGE('',*,*,#10966,.F.);
#15777=ORIENTED_EDGE('',*,*,#10967,.F.);
#15778=ORIENTED_EDGE('',*,*,#10968,.T.);
#15779=ORIENTED_EDGE('',*,*,#10969,.T.);
#15780=ORIENTED_EDGE('',*,*,#10970,.T.);
#15781=ORIENTED_EDGE('',*,*,#10946,.T.);
#15782=ORIENTED_EDGE('',*,*,#10971,.F.);
#15783=ORIENTED_EDGE('',*,*,#10930,.F.);
#15784=ORIENTED_EDGE('',*,*,#10972,.T.);
#15785=ORIENTED_EDGE('',*,*,#10973,.F.);
#15786=ORIENTED_EDGE('',*,*,#10974,.T.);
#15787=ORIENTED_EDGE('',*,*,#10975,.F.);
#15788=ORIENTED_EDGE('',*,*,#10945,.T.);
#15789=ORIENTED_EDGE('',*,*,#10959,.T.);
#15790=ORIENTED_EDGE('',*,*,#10976,.F.);
#15791=ORIENTED_EDGE('',*,*,#10931,.F.);
#15792=ORIENTED_EDGE('',*,*,#10971,.T.);
#15793=ORIENTED_EDGE('',*,*,#10958,.T.);
#15794=ORIENTED_EDGE('',*,*,#10977,.F.);
#15795=ORIENTED_EDGE('',*,*,#10932,.F.);
#15796=ORIENTED_EDGE('',*,*,#10976,.T.);
#15797=ORIENTED_EDGE('',*,*,#10957,.T.);
#15798=ORIENTED_EDGE('',*,*,#10978,.F.);
#15799=ORIENTED_EDGE('',*,*,#10933,.F.);
#15800=ORIENTED_EDGE('',*,*,#10977,.T.);
#15801=ORIENTED_EDGE('',*,*,#10956,.T.);
#15802=ORIENTED_EDGE('',*,*,#10979,.F.);
#15803=ORIENTED_EDGE('',*,*,#10934,.F.);
#15804=ORIENTED_EDGE('',*,*,#10978,.T.);
#15805=ORIENTED_EDGE('',*,*,#10955,.T.);
#15806=ORIENTED_EDGE('',*,*,#10980,.F.);
#15807=ORIENTED_EDGE('',*,*,#10935,.F.);
#15808=ORIENTED_EDGE('',*,*,#10979,.T.);
#15809=ORIENTED_EDGE('',*,*,#10954,.T.);
#15810=ORIENTED_EDGE('',*,*,#10981,.F.);
#15811=ORIENTED_EDGE('',*,*,#10936,.F.);
#15812=ORIENTED_EDGE('',*,*,#10980,.T.);
#15813=ORIENTED_EDGE('',*,*,#10953,.T.);
#15814=ORIENTED_EDGE('',*,*,#10982,.F.);
#15815=ORIENTED_EDGE('',*,*,#10937,.F.);
#15816=ORIENTED_EDGE('',*,*,#10981,.T.);
#15817=ORIENTED_EDGE('',*,*,#10952,.T.);
#15818=ORIENTED_EDGE('',*,*,#10983,.F.);
#15819=ORIENTED_EDGE('',*,*,#10938,.F.);
#15820=ORIENTED_EDGE('',*,*,#10982,.T.);
#15821=ORIENTED_EDGE('',*,*,#10951,.T.);
#15822=ORIENTED_EDGE('',*,*,#10984,.T.);
#15823=ORIENTED_EDGE('',*,*,#10985,.F.);
#15824=ORIENTED_EDGE('',*,*,#10986,.T.);
#15825=ORIENTED_EDGE('',*,*,#10987,.F.);
#15826=ORIENTED_EDGE('',*,*,#10922,.F.);
#15827=ORIENTED_EDGE('',*,*,#10988,.F.);
#15828=ORIENTED_EDGE('',*,*,#10989,.T.);
#15829=ORIENTED_EDGE('',*,*,#10990,.T.);
#15830=ORIENTED_EDGE('',*,*,#10991,.T.);
#15831=ORIENTED_EDGE('',*,*,#10939,.F.);
#15832=ORIENTED_EDGE('',*,*,#10983,.T.);
#15833=ORIENTED_EDGE('',*,*,#10992,.T.);
#15834=ORIENTED_EDGE('',*,*,#10993,.T.);
#15835=ORIENTED_EDGE('',*,*,#10949,.T.);
#15836=ORIENTED_EDGE('',*,*,#10994,.F.);
#15837=ORIENTED_EDGE('',*,*,#10941,.F.);
#15838=ORIENTED_EDGE('',*,*,#10995,.T.);
#15839=ORIENTED_EDGE('',*,*,#10996,.F.);
#15840=ORIENTED_EDGE('',*,*,#10997,.T.);
#15841=ORIENTED_EDGE('',*,*,#10998,.F.);
#15842=ORIENTED_EDGE('',*,*,#10924,.T.);
#15843=ORIENTED_EDGE('',*,*,#10999,.F.);
#15844=ORIENTED_EDGE('',*,*,#11000,.T.);
#15845=ORIENTED_EDGE('',*,*,#11001,.F.);
#15846=ORIENTED_EDGE('',*,*,#11002,.T.);
#15847=ORIENTED_EDGE('',*,*,#11003,.F.);
#15848=ORIENTED_EDGE('',*,*,#10943,.F.);
#15849=ORIENTED_EDGE('',*,*,#11004,.F.);
#15850=ORIENTED_EDGE('',*,*,#11005,.T.);
#15851=ORIENTED_EDGE('',*,*,#11006,.T.);
#15852=ORIENTED_EDGE('',*,*,#11007,.T.);
#15853=ORIENTED_EDGE('',*,*,#10928,.F.);
#15854=ORIENTED_EDGE('',*,*,#10994,.T.);
#15855=ORIENTED_EDGE('',*,*,#10948,.T.);
#15856=ORIENTED_EDGE('',*,*,#11008,.T.);
#15857=ORIENTED_EDGE('',*,*,#10998,.T.);
#15858=ORIENTED_EDGE('',*,*,#11009,.T.);
#15859=ORIENTED_EDGE('',*,*,#10988,.T.);
#15860=ORIENTED_EDGE('',*,*,#10921,.T.);
#15861=ORIENTED_EDGE('',*,*,#10996,.T.);
#15862=ORIENTED_EDGE('',*,*,#11010,.T.);
#15863=ORIENTED_EDGE('',*,*,#10990,.F.);
#15864=ORIENTED_EDGE('',*,*,#11011,.T.);
#15865=ORIENTED_EDGE('',*,*,#10992,.F.);
#15866=ORIENTED_EDGE('',*,*,#11012,.T.);
#15867=ORIENTED_EDGE('',*,*,#10985,.T.);
#15868=ORIENTED_EDGE('',*,*,#11013,.T.);
#15869=ORIENTED_EDGE('',*,*,#10987,.T.);
#15870=ORIENTED_EDGE('',*,*,#11014,.T.);
#15871=ORIENTED_EDGE('',*,*,#10999,.T.);
#15872=ORIENTED_EDGE('',*,*,#10923,.T.);
#15873=ORIENTED_EDGE('',*,*,#10867,.F.);
#15874=ORIENTED_EDGE('',*,*,#10986,.F.);
#15875=ORIENTED_EDGE('',*,*,#11012,.F.);
#15876=ORIENTED_EDGE('',*,*,#11000,.F.);
#15877=ORIENTED_EDGE('',*,*,#11014,.F.);
#15878=ORIENTED_EDGE('',*,*,#10984,.F.);
#15879=ORIENTED_EDGE('',*,*,#10950,.F.);
#15880=ORIENTED_EDGE('',*,*,#10993,.F.);
#15881=ORIENTED_EDGE('',*,*,#11013,.F.);
#15882=ORIENTED_EDGE('',*,*,#10995,.F.);
#15883=ORIENTED_EDGE('',*,*,#10940,.F.);
#15884=ORIENTED_EDGE('',*,*,#10991,.F.);
#15885=ORIENTED_EDGE('',*,*,#11010,.F.);
#15886=ORIENTED_EDGE('',*,*,#10997,.F.);
#15887=ORIENTED_EDGE('',*,*,#11011,.F.);
#15888=ORIENTED_EDGE('',*,*,#10989,.F.);
#15889=ORIENTED_EDGE('',*,*,#11009,.F.);
#15890=ORIENTED_EDGE('',*,*,#11003,.T.);
#15891=ORIENTED_EDGE('',*,*,#11015,.T.);
#15892=ORIENTED_EDGE('',*,*,#10967,.T.);
#15893=ORIENTED_EDGE('',*,*,#10944,.T.);
#15894=ORIENTED_EDGE('',*,*,#10969,.F.);
#15895=ORIENTED_EDGE('',*,*,#11016,.T.);
#15896=ORIENTED_EDGE('',*,*,#11001,.T.);
#15897=ORIENTED_EDGE('',*,*,#11017,.T.);
#15898=ORIENTED_EDGE('',*,*,#11006,.F.);
#15899=ORIENTED_EDGE('',*,*,#11018,.T.);
#15900=ORIENTED_EDGE('',*,*,#10973,.T.);
#15901=ORIENTED_EDGE('',*,*,#11019,.T.);
#15902=ORIENTED_EDGE('',*,*,#10975,.T.);
#15903=ORIENTED_EDGE('',*,*,#11020,.T.);
#15904=ORIENTED_EDGE('',*,*,#11004,.T.);
#15905=ORIENTED_EDGE('',*,*,#10942,.T.);
#15906=ORIENTED_EDGE('',*,*,#10864,.F.);
#15907=ORIENTED_EDGE('',*,*,#11002,.F.);
#15908=ORIENTED_EDGE('',*,*,#11016,.F.);
#15909=ORIENTED_EDGE('',*,*,#10968,.F.);
#15910=ORIENTED_EDGE('',*,*,#11015,.F.);
#15911=ORIENTED_EDGE('',*,*,#11008,.F.);
#15912=ORIENTED_EDGE('',*,*,#10947,.F.);
#15913=ORIENTED_EDGE('',*,*,#10970,.F.);
#15914=ORIENTED_EDGE('',*,*,#11017,.F.);
#15915=ORIENTED_EDGE('',*,*,#10974,.F.);
#15916=ORIENTED_EDGE('',*,*,#11018,.F.);
#15917=ORIENTED_EDGE('',*,*,#11005,.F.);
#15918=ORIENTED_EDGE('',*,*,#11020,.F.);
#15919=ORIENTED_EDGE('',*,*,#10972,.F.);
#15920=ORIENTED_EDGE('',*,*,#10929,.F.);
#15921=ORIENTED_EDGE('',*,*,#11007,.F.);
#15922=ORIENTED_EDGE('',*,*,#11019,.F.);
#15923=ORIENTED_EDGE('',*,*,#10914,.T.);
#15924=ORIENTED_EDGE('',*,*,#10925,.F.);
#15925=ORIENTED_EDGE('',*,*,#10915,.T.);
#15926=ORIENTED_EDGE('',*,*,#11021,.T.);
#15927=ORIENTED_EDGE('',*,*,#11022,.T.);
#15928=ORIENTED_EDGE('',*,*,#11023,.F.);
#15929=ORIENTED_EDGE('',*,*,#10962,.T.);
#15930=ORIENTED_EDGE('',*,*,#11024,.T.);
#15931=ORIENTED_EDGE('',*,*,#11025,.T.);
#15932=ORIENTED_EDGE('',*,*,#11021,.F.);
#15933=ORIENTED_EDGE('',*,*,#10961,.T.);
#15934=ORIENTED_EDGE('',*,*,#11026,.T.);
#15935=ORIENTED_EDGE('',*,*,#11027,.T.);
#15936=ORIENTED_EDGE('',*,*,#11024,.F.);
#15937=ORIENTED_EDGE('',*,*,#10966,.T.);
#15938=ORIENTED_EDGE('',*,*,#11028,.T.);
#15939=ORIENTED_EDGE('',*,*,#11029,.T.);
#15940=ORIENTED_EDGE('',*,*,#11026,.F.);
#15941=ORIENTED_EDGE('',*,*,#10965,.T.);
#15942=ORIENTED_EDGE('',*,*,#11030,.T.);
#15943=ORIENTED_EDGE('',*,*,#11031,.T.);
#15944=ORIENTED_EDGE('',*,*,#11028,.F.);
#15945=ORIENTED_EDGE('',*,*,#10964,.T.);
#15946=ORIENTED_EDGE('',*,*,#11023,.T.);
#15947=ORIENTED_EDGE('',*,*,#11032,.T.);
#15948=ORIENTED_EDGE('',*,*,#11030,.F.);
#15949=ORIENTED_EDGE('',*,*,#10963,.T.);
#15950=ORIENTED_EDGE('',*,*,#11033,.T.);
#15951=ORIENTED_EDGE('',*,*,#11034,.T.);
#15952=ORIENTED_EDGE('',*,*,#11035,.T.);
#15953=ORIENTED_EDGE('',*,*,#11036,.T.);
#15954=ORIENTED_EDGE('',*,*,#11037,.T.);
#15955=ORIENTED_EDGE('',*,*,#11038,.T.);
#15956=ORIENTED_EDGE('',*,*,#11039,.F.);
#15957=ORIENTED_EDGE('',*,*,#11025,.F.);
#15958=ORIENTED_EDGE('',*,*,#11040,.F.);
#15959=ORIENTED_EDGE('',*,*,#11037,.F.);
#15960=ORIENTED_EDGE('',*,*,#11040,.T.);
#15961=ORIENTED_EDGE('',*,*,#11027,.F.);
#15962=ORIENTED_EDGE('',*,*,#11041,.F.);
#15963=ORIENTED_EDGE('',*,*,#11038,.F.);
#15964=ORIENTED_EDGE('',*,*,#11039,.T.);
#15965=ORIENTED_EDGE('',*,*,#11036,.F.);
#15966=ORIENTED_EDGE('',*,*,#11042,.F.);
#15967=ORIENTED_EDGE('',*,*,#11022,.F.);
#15968=ORIENTED_EDGE('',*,*,#11041,.T.);
#15969=ORIENTED_EDGE('',*,*,#11029,.F.);
#15970=ORIENTED_EDGE('',*,*,#11043,.F.);
#15971=ORIENTED_EDGE('',*,*,#11033,.F.);
#15972=ORIENTED_EDGE('',*,*,#11042,.T.);
#15973=ORIENTED_EDGE('',*,*,#11035,.F.);
#15974=ORIENTED_EDGE('',*,*,#11044,.F.);
#15975=ORIENTED_EDGE('',*,*,#11032,.F.);
#15976=ORIENTED_EDGE('',*,*,#11043,.T.);
#15977=ORIENTED_EDGE('',*,*,#11031,.F.);
#15978=ORIENTED_EDGE('',*,*,#11044,.T.);
#15979=ORIENTED_EDGE('',*,*,#11034,.F.);
#15980=ORIENTED_EDGE('',*,*,#10908,.T.);
#15981=ORIENTED_EDGE('',*,*,#10909,.T.);
#15982=ORIENTED_EDGE('',*,*,#11045,.T.);
#15983=ORIENTED_EDGE('',*,*,#10960,.F.);
#15984=ORIENTED_EDGE('',*,*,#11045,.F.);
#15985=ORIENTED_EDGE('',*,*,#11046,.F.);
#15986=ORIENTED_EDGE('',*,*,#10869,.F.);
#15987=ORIENTED_EDGE('',*,*,#11046,.T.);
#15988=ORIENTED_EDGE('',*,*,#11047,.T.);
#15989=ORIENTED_EDGE('',*,*,#11048,.F.);
#15990=ORIENTED_EDGE('',*,*,#11047,.F.);
#15991=ORIENTED_EDGE('',*,*,#11049,.T.);
#15992=ORIENTED_EDGE('',*,*,#11050,.F.);
#15993=ORIENTED_EDGE('',*,*,#11051,.F.);
#15994=ORIENTED_EDGE('',*,*,#11052,.T.);
#15995=ORIENTED_EDGE('',*,*,#11053,.F.);
#15996=ORIENTED_EDGE('',*,*,#11054,.T.);
#15997=ORIENTED_EDGE('',*,*,#11055,.T.);
#15998=ORIENTED_EDGE('',*,*,#11052,.F.);
#15999=ORIENTED_EDGE('',*,*,#11056,.T.);
#16000=ORIENTED_EDGE('',*,*,#11054,.F.);
#16001=ORIENTED_EDGE('',*,*,#11057,.F.);
#16002=ORIENTED_EDGE('',*,*,#11058,.T.);
#16003=ORIENTED_EDGE('',*,*,#11059,.T.);
#16004=ORIENTED_EDGE('',*,*,#11058,.F.);
#16005=ORIENTED_EDGE('',*,*,#11060,.F.);
#16006=ORIENTED_EDGE('',*,*,#11061,.T.);
#16007=ORIENTED_EDGE('',*,*,#11062,.T.);
#16008=ORIENTED_EDGE('',*,*,#11061,.F.);
#16009=ORIENTED_EDGE('',*,*,#11063,.F.);
#16010=ORIENTED_EDGE('',*,*,#11064,.T.);
#16011=ORIENTED_EDGE('',*,*,#11065,.T.);
#16012=ORIENTED_EDGE('',*,*,#11064,.F.);
#16013=ORIENTED_EDGE('',*,*,#11066,.F.);
#16014=ORIENTED_EDGE('',*,*,#11067,.T.);
#16015=ORIENTED_EDGE('',*,*,#11068,.T.);
#16016=ORIENTED_EDGE('',*,*,#11067,.F.);
#16017=ORIENTED_EDGE('',*,*,#11069,.F.);
#16018=ORIENTED_EDGE('',*,*,#11070,.T.);
#16019=ORIENTED_EDGE('',*,*,#11071,.T.);
#16020=ORIENTED_EDGE('',*,*,#11070,.F.);
#16021=ORIENTED_EDGE('',*,*,#11072,.F.);
#16022=ORIENTED_EDGE('',*,*,#11073,.T.);
#16023=ORIENTED_EDGE('',*,*,#11074,.T.);
#16024=ORIENTED_EDGE('',*,*,#11073,.F.);
#16025=ORIENTED_EDGE('',*,*,#11075,.F.);
#16026=ORIENTED_EDGE('',*,*,#11076,.T.);
#16027=ORIENTED_EDGE('',*,*,#11077,.T.);
#16028=ORIENTED_EDGE('',*,*,#11076,.F.);
#16029=ORIENTED_EDGE('',*,*,#11078,.F.);
#16030=ORIENTED_EDGE('',*,*,#11079,.T.);
#16031=ORIENTED_EDGE('',*,*,#11080,.T.);
#16032=ORIENTED_EDGE('',*,*,#11079,.F.);
#16033=ORIENTED_EDGE('',*,*,#11081,.F.);
#16034=ORIENTED_EDGE('',*,*,#11082,.T.);
#16035=ORIENTED_EDGE('',*,*,#11083,.T.);
#16036=ORIENTED_EDGE('',*,*,#11082,.F.);
#16037=ORIENTED_EDGE('',*,*,#11084,.F.);
#16038=ORIENTED_EDGE('',*,*,#11085,.T.);
#16039=ORIENTED_EDGE('',*,*,#11086,.T.);
#16040=ORIENTED_EDGE('',*,*,#11085,.F.);
#16041=ORIENTED_EDGE('',*,*,#11087,.F.);
#16042=ORIENTED_EDGE('',*,*,#11088,.T.);
#16043=ORIENTED_EDGE('',*,*,#11089,.T.);
#16044=ORIENTED_EDGE('',*,*,#11088,.F.);
#16045=ORIENTED_EDGE('',*,*,#11090,.F.);
#16046=ORIENTED_EDGE('',*,*,#11091,.T.);
#16047=ORIENTED_EDGE('',*,*,#11092,.T.);
#16048=ORIENTED_EDGE('',*,*,#11091,.F.);
#16049=ORIENTED_EDGE('',*,*,#11093,.F.);
#16050=ORIENTED_EDGE('',*,*,#11094,.T.);
#16051=ORIENTED_EDGE('',*,*,#11095,.T.);
#16052=ORIENTED_EDGE('',*,*,#11094,.F.);
#16053=ORIENTED_EDGE('',*,*,#11096,.F.);
#16054=ORIENTED_EDGE('',*,*,#11097,.T.);
#16055=ORIENTED_EDGE('',*,*,#11098,.T.);
#16056=ORIENTED_EDGE('',*,*,#11097,.F.);
#16057=ORIENTED_EDGE('',*,*,#11099,.F.);
#16058=ORIENTED_EDGE('',*,*,#11100,.T.);
#16059=ORIENTED_EDGE('',*,*,#11101,.T.);
#16060=ORIENTED_EDGE('',*,*,#11100,.F.);
#16061=ORIENTED_EDGE('',*,*,#11102,.F.);
#16062=ORIENTED_EDGE('',*,*,#11103,.T.);
#16063=ORIENTED_EDGE('',*,*,#11104,.T.);
#16064=ORIENTED_EDGE('',*,*,#11103,.F.);
#16065=ORIENTED_EDGE('',*,*,#11105,.F.);
#16066=ORIENTED_EDGE('',*,*,#11106,.T.);
#16067=ORIENTED_EDGE('',*,*,#11107,.T.);
#16068=ORIENTED_EDGE('',*,*,#11106,.F.);
#16069=ORIENTED_EDGE('',*,*,#11108,.F.);
#16070=ORIENTED_EDGE('',*,*,#11109,.T.);
#16071=ORIENTED_EDGE('',*,*,#11110,.T.);
#16072=ORIENTED_EDGE('',*,*,#11109,.F.);
#16073=ORIENTED_EDGE('',*,*,#11111,.F.);
#16074=ORIENTED_EDGE('',*,*,#11112,.T.);
#16075=ORIENTED_EDGE('',*,*,#11113,.T.);
#16076=ORIENTED_EDGE('',*,*,#11112,.F.);
#16077=ORIENTED_EDGE('',*,*,#11114,.F.);
#16078=ORIENTED_EDGE('',*,*,#11115,.T.);
#16079=ORIENTED_EDGE('',*,*,#11116,.T.);
#16080=ORIENTED_EDGE('',*,*,#11115,.F.);
#16081=ORIENTED_EDGE('',*,*,#11117,.F.);
#16082=ORIENTED_EDGE('',*,*,#11118,.T.);
#16083=ORIENTED_EDGE('',*,*,#11119,.T.);
#16084=ORIENTED_EDGE('',*,*,#11118,.F.);
#16085=ORIENTED_EDGE('',*,*,#11120,.F.);
#16086=ORIENTED_EDGE('',*,*,#11121,.T.);
#16087=ORIENTED_EDGE('',*,*,#11122,.T.);
#16088=ORIENTED_EDGE('',*,*,#11121,.F.);
#16089=ORIENTED_EDGE('',*,*,#11123,.F.);
#16090=ORIENTED_EDGE('',*,*,#11124,.T.);
#16091=ORIENTED_EDGE('',*,*,#11125,.T.);
#16092=ORIENTED_EDGE('',*,*,#11124,.F.);
#16093=ORIENTED_EDGE('',*,*,#11126,.F.);
#16094=ORIENTED_EDGE('',*,*,#11127,.T.);
#16095=ORIENTED_EDGE('',*,*,#11128,.T.);
#16096=ORIENTED_EDGE('',*,*,#11127,.F.);
#16097=ORIENTED_EDGE('',*,*,#11129,.F.);
#16098=ORIENTED_EDGE('',*,*,#11130,.T.);
#16099=ORIENTED_EDGE('',*,*,#11131,.T.);
#16100=ORIENTED_EDGE('',*,*,#11130,.F.);
#16101=ORIENTED_EDGE('',*,*,#11132,.F.);
#16102=ORIENTED_EDGE('',*,*,#11133,.T.);
#16103=ORIENTED_EDGE('',*,*,#11134,.T.);
#16104=ORIENTED_EDGE('',*,*,#11133,.F.);
#16105=ORIENTED_EDGE('',*,*,#11135,.F.);
#16106=ORIENTED_EDGE('',*,*,#11136,.T.);
#16107=ORIENTED_EDGE('',*,*,#11137,.T.);
#16108=ORIENTED_EDGE('',*,*,#11136,.F.);
#16109=ORIENTED_EDGE('',*,*,#11138,.F.);
#16110=ORIENTED_EDGE('',*,*,#11139,.T.);
#16111=ORIENTED_EDGE('',*,*,#11140,.T.);
#16112=ORIENTED_EDGE('',*,*,#11139,.F.);
#16113=ORIENTED_EDGE('',*,*,#11141,.F.);
#16114=ORIENTED_EDGE('',*,*,#11142,.T.);
#16115=ORIENTED_EDGE('',*,*,#11143,.T.);
#16116=ORIENTED_EDGE('',*,*,#11142,.F.);
#16117=ORIENTED_EDGE('',*,*,#11144,.F.);
#16118=ORIENTED_EDGE('',*,*,#11145,.T.);
#16119=ORIENTED_EDGE('',*,*,#11146,.T.);
#16120=ORIENTED_EDGE('',*,*,#11145,.F.);
#16121=ORIENTED_EDGE('',*,*,#11147,.F.);
#16122=ORIENTED_EDGE('',*,*,#11148,.T.);
#16123=ORIENTED_EDGE('',*,*,#11149,.T.);
#16124=ORIENTED_EDGE('',*,*,#11148,.F.);
#16125=ORIENTED_EDGE('',*,*,#11150,.F.);
#16126=ORIENTED_EDGE('',*,*,#11151,.T.);
#16127=ORIENTED_EDGE('',*,*,#11152,.T.);
#16128=ORIENTED_EDGE('',*,*,#11151,.F.);
#16129=ORIENTED_EDGE('',*,*,#11153,.F.);
#16130=ORIENTED_EDGE('',*,*,#11154,.T.);
#16131=ORIENTED_EDGE('',*,*,#11155,.T.);
#16132=ORIENTED_EDGE('',*,*,#11154,.F.);
#16133=ORIENTED_EDGE('',*,*,#11156,.F.);
#16134=ORIENTED_EDGE('',*,*,#11157,.T.);
#16135=ORIENTED_EDGE('',*,*,#11158,.T.);
#16136=ORIENTED_EDGE('',*,*,#11157,.F.);
#16137=ORIENTED_EDGE('',*,*,#11159,.F.);
#16138=ORIENTED_EDGE('',*,*,#11160,.T.);
#16139=ORIENTED_EDGE('',*,*,#11161,.T.);
#16140=ORIENTED_EDGE('',*,*,#11160,.F.);
#16141=ORIENTED_EDGE('',*,*,#11162,.F.);
#16142=ORIENTED_EDGE('',*,*,#11163,.T.);
#16143=ORIENTED_EDGE('',*,*,#11164,.T.);
#16144=ORIENTED_EDGE('',*,*,#11163,.F.);
#16145=ORIENTED_EDGE('',*,*,#11165,.F.);
#16146=ORIENTED_EDGE('',*,*,#11166,.T.);
#16147=ORIENTED_EDGE('',*,*,#11167,.T.);
#16148=ORIENTED_EDGE('',*,*,#11166,.F.);
#16149=ORIENTED_EDGE('',*,*,#11168,.F.);
#16150=ORIENTED_EDGE('',*,*,#11169,.T.);
#16151=ORIENTED_EDGE('',*,*,#11170,.T.);
#16152=ORIENTED_EDGE('',*,*,#11169,.F.);
#16153=ORIENTED_EDGE('',*,*,#11171,.F.);
#16154=ORIENTED_EDGE('',*,*,#11172,.T.);
#16155=ORIENTED_EDGE('',*,*,#11173,.T.);
#16156=ORIENTED_EDGE('',*,*,#11172,.F.);
#16157=ORIENTED_EDGE('',*,*,#11174,.F.);
#16158=ORIENTED_EDGE('',*,*,#11175,.T.);
#16159=ORIENTED_EDGE('',*,*,#11176,.T.);
#16160=ORIENTED_EDGE('',*,*,#11175,.F.);
#16161=ORIENTED_EDGE('',*,*,#11177,.F.);
#16162=ORIENTED_EDGE('',*,*,#11050,.T.);
#16163=ORIENTED_EDGE('',*,*,#11176,.F.);
#16164=ORIENTED_EDGE('',*,*,#11049,.F.);
#16165=ORIENTED_EDGE('',*,*,#11055,.F.);
#16166=ORIENTED_EDGE('',*,*,#11056,.F.);
#16167=ORIENTED_EDGE('',*,*,#11059,.F.);
#16168=ORIENTED_EDGE('',*,*,#11062,.F.);
#16169=ORIENTED_EDGE('',*,*,#11065,.F.);
#16170=ORIENTED_EDGE('',*,*,#11068,.F.);
#16171=ORIENTED_EDGE('',*,*,#11071,.F.);
#16172=ORIENTED_EDGE('',*,*,#11074,.F.);
#16173=ORIENTED_EDGE('',*,*,#11077,.F.);
#16174=ORIENTED_EDGE('',*,*,#11080,.F.);
#16175=ORIENTED_EDGE('',*,*,#11083,.F.);
#16176=ORIENTED_EDGE('',*,*,#11086,.F.);
#16177=ORIENTED_EDGE('',*,*,#11089,.F.);
#16178=ORIENTED_EDGE('',*,*,#11092,.F.);
#16179=ORIENTED_EDGE('',*,*,#11095,.F.);
#16180=ORIENTED_EDGE('',*,*,#11098,.F.);
#16181=ORIENTED_EDGE('',*,*,#11101,.F.);
#16182=ORIENTED_EDGE('',*,*,#11104,.F.);
#16183=ORIENTED_EDGE('',*,*,#11107,.F.);
#16184=ORIENTED_EDGE('',*,*,#11110,.F.);
#16185=ORIENTED_EDGE('',*,*,#11113,.F.);
#16186=ORIENTED_EDGE('',*,*,#11116,.F.);
#16187=ORIENTED_EDGE('',*,*,#11119,.F.);
#16188=ORIENTED_EDGE('',*,*,#11122,.F.);
#16189=ORIENTED_EDGE('',*,*,#11125,.F.);
#16190=ORIENTED_EDGE('',*,*,#11128,.F.);
#16191=ORIENTED_EDGE('',*,*,#11131,.F.);
#16192=ORIENTED_EDGE('',*,*,#11134,.F.);
#16193=ORIENTED_EDGE('',*,*,#11137,.F.);
#16194=ORIENTED_EDGE('',*,*,#11140,.F.);
#16195=ORIENTED_EDGE('',*,*,#11143,.F.);
#16196=ORIENTED_EDGE('',*,*,#11146,.F.);
#16197=ORIENTED_EDGE('',*,*,#11149,.F.);
#16198=ORIENTED_EDGE('',*,*,#11152,.F.);
#16199=ORIENTED_EDGE('',*,*,#11155,.F.);
#16200=ORIENTED_EDGE('',*,*,#11158,.F.);
#16201=ORIENTED_EDGE('',*,*,#11161,.F.);
#16202=ORIENTED_EDGE('',*,*,#11164,.F.);
#16203=ORIENTED_EDGE('',*,*,#11167,.F.);
#16204=ORIENTED_EDGE('',*,*,#11170,.F.);
#16205=ORIENTED_EDGE('',*,*,#11173,.F.);
#16206=ORIENTED_EDGE('',*,*,#11048,.T.);
#16207=ORIENTED_EDGE('',*,*,#11177,.T.);
#16208=ORIENTED_EDGE('',*,*,#11174,.T.);
#16209=ORIENTED_EDGE('',*,*,#11171,.T.);
#16210=ORIENTED_EDGE('',*,*,#11168,.T.);
#16211=ORIENTED_EDGE('',*,*,#11165,.T.);
#16212=ORIENTED_EDGE('',*,*,#11162,.T.);
#16213=ORIENTED_EDGE('',*,*,#11159,.T.);
#16214=ORIENTED_EDGE('',*,*,#11156,.T.);
#16215=ORIENTED_EDGE('',*,*,#11153,.T.);
#16216=ORIENTED_EDGE('',*,*,#11150,.T.);
#16217=ORIENTED_EDGE('',*,*,#11147,.T.);
#16218=ORIENTED_EDGE('',*,*,#11144,.T.);
#16219=ORIENTED_EDGE('',*,*,#11141,.T.);
#16220=ORIENTED_EDGE('',*,*,#11138,.T.);
#16221=ORIENTED_EDGE('',*,*,#11135,.T.);
#16222=ORIENTED_EDGE('',*,*,#11132,.T.);
#16223=ORIENTED_EDGE('',*,*,#11129,.T.);
#16224=ORIENTED_EDGE('',*,*,#11126,.T.);
#16225=ORIENTED_EDGE('',*,*,#11123,.T.);
#16226=ORIENTED_EDGE('',*,*,#11120,.T.);
#16227=ORIENTED_EDGE('',*,*,#11117,.T.);
#16228=ORIENTED_EDGE('',*,*,#11114,.T.);
#16229=ORIENTED_EDGE('',*,*,#11111,.T.);
#16230=ORIENTED_EDGE('',*,*,#11108,.T.);
#16231=ORIENTED_EDGE('',*,*,#11105,.T.);
#16232=ORIENTED_EDGE('',*,*,#11102,.T.);
#16233=ORIENTED_EDGE('',*,*,#11099,.T.);
#16234=ORIENTED_EDGE('',*,*,#11096,.T.);
#16235=ORIENTED_EDGE('',*,*,#11093,.T.);
#16236=ORIENTED_EDGE('',*,*,#11090,.T.);
#16237=ORIENTED_EDGE('',*,*,#11087,.T.);
#16238=ORIENTED_EDGE('',*,*,#11084,.T.);
#16239=ORIENTED_EDGE('',*,*,#11081,.T.);
#16240=ORIENTED_EDGE('',*,*,#11078,.T.);
#16241=ORIENTED_EDGE('',*,*,#11075,.T.);
#16242=ORIENTED_EDGE('',*,*,#11072,.T.);
#16243=ORIENTED_EDGE('',*,*,#11069,.T.);
#16244=ORIENTED_EDGE('',*,*,#11066,.T.);
#16245=ORIENTED_EDGE('',*,*,#11063,.T.);
#16246=ORIENTED_EDGE('',*,*,#11060,.T.);
#16247=ORIENTED_EDGE('',*,*,#11057,.T.);
#16248=ORIENTED_EDGE('',*,*,#11053,.T.);
#16249=ORIENTED_EDGE('',*,*,#11051,.T.);
#16250=ORIENTED_EDGE('',*,*,#10863,.F.);
#16251=ORIENTED_EDGE('',*,*,#10861,.T.);
#16769=PLANE('',#19169);
#16770=PLANE('',#19237);
#16771=PLANE('',#19238);
#16772=PLANE('',#19240);
#16773=PLANE('',#19246);
#16774=PLANE('',#19247);
#16775=PLANE('',#19257);
#16776=PLANE('',#19259);
#16777=PLANE('',#19277);
#16778=PLANE('',#19282);
#16779=PLANE('',#19285);
#16780=PLANE('',#19290);
#16781=PLANE('',#19291);
#16782=PLANE('',#19292);
#16783=PLANE('',#19293);
#16784=PLANE('',#19295);
#16785=PLANE('',#19296);
#16786=PLANE('',#19297);
#16787=PLANE('',#19298);
#16788=PLANE('',#19303);
#16789=PLANE('',#19308);
#16790=PLANE('',#19313);
#16791=PLANE('',#19314);
#16792=PLANE('',#19315);
#16793=PLANE('',#19316);
#16794=PLANE('',#19321);
#16795=PLANE('',#19322);
#16796=PLANE('',#19323);
#16797=PLANE('',#19324);
#16798=PLANE('',#19329);
#16799=PLANE('',#19330);
#16800=PLANE('',#19331);
#16801=PLANE('',#19332);
#16802=PLANE('',#19333);
#16803=PLANE('',#19334);
#16804=PLANE('',#19335);
#16805=PLANE('',#19336);
#16806=PLANE('',#19337);
#16807=PLANE('',#19351);
#16808=PLANE('',#19355);
#16809=PLANE('',#19359);
#16810=PLANE('',#19360);
#16811=PLANE('',#19361);
#16812=PLANE('',#19362);
#16813=PLANE('',#19363);
#16814=PLANE('',#19364);
#16815=PLANE('',#19365);
#16816=PLANE('',#19366);
#16817=PLANE('',#19367);
#16818=PLANE('',#19368);
#16819=PLANE('',#19369);
#16820=PLANE('',#19370);
#16821=PLANE('',#19371);
#16822=PLANE('',#19372);
#16823=PLANE('',#19373);
#16824=PLANE('',#19374);
#16825=PLANE('',#19375);
#16826=PLANE('',#19376);
#16827=PLANE('',#19377);
#16828=PLANE('',#19378);
#16829=PLANE('',#19379);
#16830=PLANE('',#19380);
#16831=PLANE('',#19381);
#16832=PLANE('',#19382);
#16833=PLANE('',#19383);
#16834=PLANE('',#19384);
#16835=PLANE('',#19385);
#16836=PLANE('',#19386);
#16837=PLANE('',#19387);
#16838=PLANE('',#19388);
#16839=PLANE('',#19389);
#16840=PLANE('',#19390);
#16841=PLANE('',#19391);
#16842=PLANE('',#19392);
#16843=PLANE('',#19393);
#16844=PLANE('',#19394);
#16845=PLANE('',#19395);
#16846=PLANE('',#19396);
#16847=PLANE('',#19400);
#16848=PLANE('',#19401);
#16849=PLANE('',#19402);
#16850=PLANE('',#19403);
#16851=PLANE('',#19404);
#17622=ADVANCED_FACE('',(#2287,#956),#16769,.T.);
#17623=ADVANCED_FACE('',(#2288),#189,.T.);
#17624=ADVANCED_FACE('',(#2289),#710,.F.);
#17625=ADVANCED_FACE('',(#2290),#711,.F.);
#17626=ADVANCED_FACE('',(#2291),#712,.F.);
#17627=ADVANCED_FACE('',(#2292),#713,.F.);
#17628=ADVANCED_FACE('',(#2293),#714,.F.);
#17629=ADVANCED_FACE('',(#2294),#715,.F.);
#17630=ADVANCED_FACE('',(#2295),#716,.F.);
#17631=ADVANCED_FACE('',(#2296),#717,.F.);
#17632=ADVANCED_FACE('',(#2297),#718,.F.);
#17633=ADVANCED_FACE('',(#2298),#719,.F.);
#17634=ADVANCED_FACE('',(#2299),#720,.F.);
#17635=ADVANCED_FACE('',(#2300),#721,.F.);
#17636=ADVANCED_FACE('',(#2301),#722,.F.);
#17637=ADVANCED_FACE('',(#2302),#723,.F.);
#17638=ADVANCED_FACE('',(#2303),#724,.F.);
#17639=ADVANCED_FACE('',(#2304),#725,.F.);
#17640=ADVANCED_FACE('',(#2305),#726,.F.);
#17641=ADVANCED_FACE('',(#2306),#727,.F.);
#17642=ADVANCED_FACE('',(#2307),#728,.F.);
#17643=ADVANCED_FACE('',(#2308),#729,.F.);
#17644=ADVANCED_FACE('',(#2309),#730,.F.);
#17645=ADVANCED_FACE('',(#2310),#731,.F.);
#17646=ADVANCED_FACE('',(#2311),#732,.F.);
#17647=ADVANCED_FACE('',(#2312),#733,.F.);
#17648=ADVANCED_FACE('',(#2313),#734,.F.);
#17649=ADVANCED_FACE('',(#2314),#735,.F.);
#17650=ADVANCED_FACE('',(#2315),#736,.F.);
#17651=ADVANCED_FACE('',(#2316),#737,.F.);
#17652=ADVANCED_FACE('',(#2317),#738,.F.);
#17653=ADVANCED_FACE('',(#2318),#739,.T.);
#17654=ADVANCED_FACE('',(#2319),#740,.T.);
#17655=ADVANCED_FACE('',(#2320),#741,.T.);
#17656=ADVANCED_FACE('',(#2321),#230,.T.);
#17657=ADVANCED_FACE('',(#2322),#231,.T.);
#17658=ADVANCED_FACE('',(#2323),#232,.T.);
#17659=ADVANCED_FACE('',(#2324),#233,.T.);
#17660=ADVANCED_FACE('',(#2325),#742,.F.);
#17661=ADVANCED_FACE('',(#2326),#743,.T.);
#17662=ADVANCED_FACE('',(#2327,#957),#16770,.F.);
#17663=ADVANCED_FACE('',(#2328,#958),#16771,.T.);
#17664=ADVANCED_FACE('',(#2329,#959),#16772,.F.);
#17665=ADVANCED_FACE('',(#2330),#744,.T.);
#17666=ADVANCED_FACE('',(#2331),#415,.T.);
#17667=ADVANCED_FACE('',(#2332),#745,.F.);
#17668=ADVANCED_FACE('',(#2333),#416,.T.);
#17669=ADVANCED_FACE('',(#2334),#16773,.F.);
#17670=ADVANCED_FACE('',(#2335),#16774,.F.);
#17671=ADVANCED_FACE('',(#2336),#746,.T.);
#17672=ADVANCED_FACE('',(#2337),#190,.F.);
#17673=ADVANCED_FACE('',(#2338),#191,.F.);
#17674=ADVANCED_FACE('',(#2339),#192,.T.);
#17675=ADVANCED_FACE('',(#2340,#960),#16775,.T.);
#17676=ADVANCED_FACE('',(#2341),#747,.F.);
#17677=ADVANCED_FACE('',(#2342),#16776,.F.);
#17678=ADVANCED_FACE('',(#2343),#234,.T.);
#17679=ADVANCED_FACE('',(#2344),#235,.T.);
#17680=ADVANCED_FACE('',(#2345),#748,.T.);
#17681=ADVANCED_FACE('',(#2346),#749,.T.);
#17682=ADVANCED_FACE('',(#2347),#750,.T.);
#17683=ADVANCED_FACE('',(#2348),#751,.T.);
#17684=ADVANCED_FACE('',(#2349,#961,#962),#16777,.T.);
#17685=ADVANCED_FACE('',(#2350),#752,.T.);
#17686=ADVANCED_FACE('',(#2351,#963,#964),#16778,.F.);
#17687=ADVANCED_FACE('',(#2352),#16779,.F.);
#17688=ADVANCED_FACE('',(#2353),#16780,.F.);
#17689=ADVANCED_FACE('',(#2354),#16781,.F.);
#17690=ADVANCED_FACE('',(#2355),#16782,.F.);
#17691=ADVANCED_FACE('',(#2356),#16783,.F.);
#17692=ADVANCED_FACE('',(#2357),#753,.T.);
#17693=ADVANCED_FACE('',(#2358),#16784,.F.);
#17694=ADVANCED_FACE('',(#2359),#16785,.F.);
#17695=ADVANCED_FACE('',(#2360),#16786,.F.);
#17696=ADVANCED_FACE('',(#2361),#16787,.F.);
#17697=ADVANCED_FACE('',(#2362),#16788,.F.);
#17698=ADVANCED_FACE('',(#2363),#16789,.F.);
#17699=ADVANCED_FACE('',(#2364),#16790,.T.);
#17700=ADVANCED_FACE('',(#2365),#16791,.F.);
#17701=ADVANCED_FACE('',(#2366),#16792,.F.);
#17702=ADVANCED_FACE('',(#2367,#965),#16793,.F.);
#17703=ADVANCED_FACE('',(#2368),#754,.F.);
#17704=ADVANCED_FACE('',(#2369),#755,.T.);
#17705=ADVANCED_FACE('',(#2370),#756,.F.);
#17706=ADVANCED_FACE('',(#2371),#757,.T.);
#17707=ADVANCED_FACE('',(#2372),#16794,.T.);
#17708=ADVANCED_FACE('',(#2373),#16795,.F.);
#17709=ADVANCED_FACE('',(#2374),#16796,.F.);
#17710=ADVANCED_FACE('',(#2375,#966),#16797,.T.);
#17711=ADVANCED_FACE('',(#2376),#758,.T.);
#17712=ADVANCED_FACE('',(#2377),#759,.F.);
#17713=ADVANCED_FACE('',(#2378),#760,.F.);
#17714=ADVANCED_FACE('',(#2379),#761,.T.);
#17715=ADVANCED_FACE('',(#2380,#967),#16798,.F.);
#17716=ADVANCED_FACE('',(#2381),#16799,.T.);
#17717=ADVANCED_FACE('',(#2382),#16800,.T.);
#17718=ADVANCED_FACE('',(#2383),#16801,.T.);
#17719=ADVANCED_FACE('',(#2384),#16802,.T.);
#17720=ADVANCED_FACE('',(#2385),#16803,.T.);
#17721=ADVANCED_FACE('',(#2386),#16804,.T.);
#17722=ADVANCED_FACE('',(#2387),#16805,.T.);
#17723=ADVANCED_FACE('',(#2388),#16806,.F.);
#17724=ADVANCED_FACE('',(#2389),#762,.T.);
#17725=ADVANCED_FACE('',(#2390),#763,.T.);
#17726=ADVANCED_FACE('',(#2391),#764,.T.);
#17727=ADVANCED_FACE('',(#2392),#765,.T.);
#17728=ADVANCED_FACE('',(#2393),#766,.T.);
#17729=ADVANCED_FACE('',(#2394),#767,.T.);
#17730=ADVANCED_FACE('',(#2395),#768,.F.);
#17731=ADVANCED_FACE('',(#2396,#968),#16807,.F.);
#17732=ADVANCED_FACE('',(#2397),#769,.F.);
#17733=ADVANCED_FACE('',(#2398),#16808,.F.);
#17734=ADVANCED_FACE('',(#2399),#770,.T.);
#17735=ADVANCED_FACE('',(#2400),#16809,.F.);
#17736=ADVANCED_FACE('',(#2401),#16810,.F.);
#17737=ADVANCED_FACE('',(#2402),#16811,.F.);
#17738=ADVANCED_FACE('',(#2403),#16812,.F.);
#17739=ADVANCED_FACE('',(#2404),#16813,.F.);
#17740=ADVANCED_FACE('',(#2405),#16814,.F.);
#17741=ADVANCED_FACE('',(#2406),#16815,.F.);
#17742=ADVANCED_FACE('',(#2407),#16816,.F.);
#17743=ADVANCED_FACE('',(#2408),#16817,.F.);
#17744=ADVANCED_FACE('',(#2409),#16818,.F.);
#17745=ADVANCED_FACE('',(#2410),#16819,.F.);
#17746=ADVANCED_FACE('',(#2411),#16820,.F.);
#17747=ADVANCED_FACE('',(#2412),#16821,.F.);
#17748=ADVANCED_FACE('',(#2413),#16822,.F.);
#17749=ADVANCED_FACE('',(#2414),#16823,.F.);
#17750=ADVANCED_FACE('',(#2415),#16824,.F.);
#17751=ADVANCED_FACE('',(#2416),#16825,.F.);
#17752=ADVANCED_FACE('',(#2417),#16826,.F.);
#17753=ADVANCED_FACE('',(#2418),#16827,.F.);
#17754=ADVANCED_FACE('',(#2419),#16828,.F.);
#17755=ADVANCED_FACE('',(#2420),#16829,.F.);
#17756=ADVANCED_FACE('',(#2421),#16830,.F.);
#17757=ADVANCED_FACE('',(#2422),#16831,.F.);
#17758=ADVANCED_FACE('',(#2423),#16832,.F.);
#17759=ADVANCED_FACE('',(#2424),#16833,.F.);
#17760=ADVANCED_FACE('',(#2425),#16834,.F.);
#17761=ADVANCED_FACE('',(#2426),#16835,.F.);
#17762=ADVANCED_FACE('',(#2427),#16836,.F.);
#17763=ADVANCED_FACE('',(#2428),#16837,.F.);
#17764=ADVANCED_FACE('',(#2429),#16838,.F.);
#17765=ADVANCED_FACE('',(#2430),#16839,.F.);
#17766=ADVANCED_FACE('',(#2431),#16840,.F.);
#17767=ADVANCED_FACE('',(#2432),#16841,.F.);
#17768=ADVANCED_FACE('',(#2433),#16842,.F.);
#17769=ADVANCED_FACE('',(#2434),#16843,.F.);
#17770=ADVANCED_FACE('',(#2435),#16844,.F.);
#17771=ADVANCED_FACE('',(#2436),#16845,.F.);
#17772=ADVANCED_FACE('',(#2437),#16846,.F.);
#17773=ADVANCED_FACE('',(#2438),#771,.T.);
#17774=ADVANCED_FACE('',(#2439),#16847,.F.);
#17775=ADVANCED_FACE('',(#2440),#16848,.F.);
#17776=ADVANCED_FACE('',(#2441,#969),#16849,.F.);
#17777=ADVANCED_FACE('',(#2442,#970),#16850,.T.);
#17778=ADVANCED_FACE('',(#2443),#16851,.T.);
#17801=CLOSED_SHELL('',(#17622,#17623,#17624));
#17802=CLOSED_SHELL('',(#17625,#17626,#17627,#17628,#17629,#17630,#17631,
#17632,#17633,#17634,#17635,#17636,#17637,#17638,#17639,#17640,#17641,#17642,
#17643,#17644,#17645,#17646,#17647,#17648,#17649,#17650,#17651,#17652,#17653,
#17654,#17655,#17656,#17657,#17658,#17659,#17660,#17661,#17662,#17663,#17664,
#17665,#17666,#17667,#17668,#17669,#17670,#17671,#17672,#17673,#17674,#17675,
#17676,#17677,#17678,#17679,#17680,#17681,#17682,#17683,#17684,#17685,#17686,
#17687,#17688,#17689,#17690,#17691,#17692,#17693,#17694,#17695,#17696,#17697,
#17698,#17699,#17700,#17701,#17702,#17703,#17704,#17705,#17706,#17707,#17708,
#17709,#17710,#17711,#17712,#17713,#17714,#17715,#17716,#17717,#17718,#17719,
#17720,#17721,#17722,#17723,#17724,#17725,#17726,#17727,#17728,#17729,#17730,
#17731,#17732,#17733,#17734,#17735,#17736,#17737,#17738,#17739,#17740,#17741,
#17742,#17743,#17744,#17745,#17746,#17747,#17748,#17749,#17750,#17751,#17752,
#17753,#17754,#17755,#17756,#17757,#17758,#17759,#17760,#17761,#17762,#17763,
#17764,#17765,#17766,#17767,#17768,#17769,#17770,#17771,#17772,#17773,#17774,
#17775,#17776,#17777,#17778));
#19168=AXIS2_PLACEMENT_3D('',#33752,#23357,#23358);
#19169=AXIS2_PLACEMENT_3D('',#33753,#23359,#23360);
#19170=AXIS2_PLACEMENT_3D('',#33755,#23361,#23362);
#19171=AXIS2_PLACEMENT_3D('',#33757,#23363,#23364);
#19172=AXIS2_PLACEMENT_3D('',#33758,#23365,#23366);
#19173=AXIS2_PLACEMENT_3D('',#33761,#23367,#23368);
#19174=AXIS2_PLACEMENT_3D('',#33762,#23369,#23370);
#19175=AXIS2_PLACEMENT_3D('',#33764,#23372,#23373);
#19176=AXIS2_PLACEMENT_3D('',#33766,#23375,#23376);
#19177=AXIS2_PLACEMENT_3D('',#33773,#23379,#23380);
#19178=AXIS2_PLACEMENT_3D('',#33796,#23381,#23382);
#19179=AXIS2_PLACEMENT_3D('',#33872,#23384,#23385);
#19180=AXIS2_PLACEMENT_3D('',#33950,#23387,#23388);
#19181=AXIS2_PLACEMENT_3D('',#34026,#23390,#23391);
#19182=AXIS2_PLACEMENT_3D('',#34102,#23393,#23394);
#19183=AXIS2_PLACEMENT_3D('',#34178,#23396,#23397);
#19184=AXIS2_PLACEMENT_3D('',#34256,#23399,#23400);
#19185=AXIS2_PLACEMENT_3D('',#34332,#23402,#23403);
#19186=AXIS2_PLACEMENT_3D('',#34408,#23405,#23406);
#19187=AXIS2_PLACEMENT_3D('',#34486,#23408,#23409);
#19188=AXIS2_PLACEMENT_3D('',#34562,#23411,#23412);
#19189=AXIS2_PLACEMENT_3D('',#34638,#23414,#23415);
#19190=AXIS2_PLACEMENT_3D('',#34714,#23417,#23418);
#19191=AXIS2_PLACEMENT_3D('',#34719,#23420,#23421);
#19192=AXIS2_PLACEMENT_3D('',#34728,#23422,#23423);
#19193=AXIS2_PLACEMENT_3D('',#34749,#23426,#23427);
#19194=AXIS2_PLACEMENT_3D('',#34779,#23429,#23430);
#19195=AXIS2_PLACEMENT_3D('',#34809,#23432,#23433);
#19196=AXIS2_PLACEMENT_3D('',#34839,#23435,#23436);
#19197=AXIS2_PLACEMENT_3D('',#34869,#23438,#23439);
#19198=AXIS2_PLACEMENT_3D('',#34899,#23441,#23442);
#19199=AXIS2_PLACEMENT_3D('',#34929,#23444,#23445);
#19200=AXIS2_PLACEMENT_3D('',#34959,#23447,#23448);
#19201=AXIS2_PLACEMENT_3D('',#34989,#23450,#23451);
#19202=AXIS2_PLACEMENT_3D('',#35019,#23453,#23454);
#19203=AXIS2_PLACEMENT_3D('',#35049,#23456,#23457);
#19204=AXIS2_PLACEMENT_3D('',#35079,#23459,#23460);
#19205=AXIS2_PLACEMENT_3D('',#35109,#23462,#23463);
#19206=AXIS2_PLACEMENT_3D('',#35130,#23466,#23467);
#19207=AXIS2_PLACEMENT_3D('',#35132,#23468,#23469);
#19208=AXIS2_PLACEMENT_3D('',#35135,#23471,#23472);
#19209=AXIS2_PLACEMENT_3D('',#35136,#23473,#23474);
#19210=AXIS2_PLACEMENT_3D('',#35138,#23475,#23476);
#19211=AXIS2_PLACEMENT_3D('',#35141,#23478,#23479);
#19212=AXIS2_PLACEMENT_3D('',#35142,#23480,#23481);
#19213=AXIS2_PLACEMENT_3D('',#35144,#23482,#23483);
#19214=AXIS2_PLACEMENT_3D('',#35147,#23485,#23486);
#19215=AXIS2_PLACEMENT_3D('',#35148,#23487,#23488);
#19216=AXIS2_PLACEMENT_3D('',#35150,#23489,#23490);
#19217=AXIS2_PLACEMENT_3D('',#35152,#23491,#23492);
#19218=AXIS2_PLACEMENT_3D('',#35154,#23493,#23494);
#19219=AXIS2_PLACEMENT_3D('',#35155,#23495,#23496);
#19220=AXIS2_PLACEMENT_3D('',#35156,#23497,#23498);
#19221=AXIS2_PLACEMENT_3D('',#35159,#23499,#23500);
#19222=AXIS2_PLACEMENT_3D('',#35160,#23501,#23502);
#19223=AXIS2_PLACEMENT_3D('',#35162,#23503,#23504);
#19224=AXIS2_PLACEMENT_3D('',#35163,#23505,#23506);
#19225=AXIS2_PLACEMENT_3D('',#35164,#23507,#23508);
#19226=AXIS2_PLACEMENT_3D('',#35167,#23509,#23510);
#19227=AXIS2_PLACEMENT_3D('',#35168,#23511,#23512);
#19228=AXIS2_PLACEMENT_3D('',#35170,#23513,#23514);
#19229=AXIS2_PLACEMENT_3D('',#35171,#23515,#23516);
#19230=AXIS2_PLACEMENT_3D('',#35172,#23517,#23518);
#19231=AXIS2_PLACEMENT_3D('',#35174,#23519,#23520);
#19232=AXIS2_PLACEMENT_3D('',#35176,#23521,#23522);
#19233=AXIS2_PLACEMENT_3D('',#35178,#23523,#23524);
#19234=AXIS2_PLACEMENT_3D('',#35179,#23525,#23526);
#19235=AXIS2_PLACEMENT_3D('',#35180,#23527,#23528);
#19236=AXIS2_PLACEMENT_3D('',#35182,#23530,#23531);
#19237=AXIS2_PLACEMENT_3D('',#35184,#23533,#23534);
#19238=AXIS2_PLACEMENT_3D('',#35185,#23535,#23536);
#19239=AXIS2_PLACEMENT_3D('',#35187,#23537,#23538);
#19240=AXIS2_PLACEMENT_3D('',#35188,#23539,#23540);
#19241=AXIS2_PLACEMENT_3D('',#35190,#23541,#23542);
#19242=AXIS2_PLACEMENT_3D('',#35191,#23543,#23544);
#19243=AXIS2_PLACEMENT_3D('',#35207,#23545,#23546);
#19244=AXIS2_PLACEMENT_3D('',#35208,#23547,#23548);
#19245=AXIS2_PLACEMENT_3D('',#35599,#23552,#23553);
#19246=AXIS2_PLACEMENT_3D('',#35997,#23556,#23557);
#19247=AXIS2_PLACEMENT_3D('',#35999,#23559,#23560);
#19248=AXIS2_PLACEMENT_3D('',#36000,#23561,#23562);
#19249=AXIS2_PLACEMENT_3D('',#36001,#23563,#23564);
#19250=AXIS2_PLACEMENT_3D('',#36002,#23565,#23566);
#19251=AXIS2_PLACEMENT_3D('',#36005,#23568,#23569);
#19252=AXIS2_PLACEMENT_3D('',#36006,#23570,#23571);
#19253=AXIS2_PLACEMENT_3D('',#36008,#23573,#23574);
#19254=AXIS2_PLACEMENT_3D('',#36011,#23575,#23576);
#19255=AXIS2_PLACEMENT_3D('',#36012,#23577,#23578);
#19256=AXIS2_PLACEMENT_3D('',#36015,#23580,#23581);
#19257=AXIS2_PLACEMENT_3D('',#36016,#23582,#23583);
#19258=AXIS2_PLACEMENT_3D('',#36017,#23584,#23585);
#19259=AXIS2_PLACEMENT_3D('',#36018,#23586,#23587);
#19260=AXIS2_PLACEMENT_3D('',#36019,#23588,#23589);
#19261=AXIS2_PLACEMENT_3D('',#36021,#23590,#23591);
#19262=AXIS2_PLACEMENT_3D('',#36023,#23592,#23593);
#19263=AXIS2_PLACEMENT_3D('',#36024,#23594,#23595);
#19264=AXIS2_PLACEMENT_3D('',#36025,#23596,#23597);
#19265=AXIS2_PLACEMENT_3D('',#36027,#23598,#23599);
#19266=AXIS2_PLACEMENT_3D('',#36029,#23600,#23601);
#19267=AXIS2_PLACEMENT_3D('',#36030,#23602,#23603);
#19268=AXIS2_PLACEMENT_3D('',#36031,#23604,#23605);
#19269=AXIS2_PLACEMENT_3D('',#36033,#23607,#23608);
#19270=AXIS2_PLACEMENT_3D('',#36035,#23609,#23610);
#19271=AXIS2_PLACEMENT_3D('',#36037,#23612,#23613);
#19272=AXIS2_PLACEMENT_3D('',#36040,#23614,#23615);
#19273=AXIS2_PLACEMENT_3D('',#36044,#23617,#23618);
#19274=AXIS2_PLACEMENT_3D('',#36046,#23620,#23621);
#19275=AXIS2_PLACEMENT_3D('',#36048,#23622,#23623);
#19276=AXIS2_PLACEMENT_3D('',#36051,#23625,#23626);
#19277=AXIS2_PLACEMENT_3D('',#36052,#23627,#23628);
#19278=AXIS2_PLACEMENT_3D('',#36069,#23636,#23637);
#19279=AXIS2_PLACEMENT_3D('',#36081,#23644,#23645);
#19280=AXIS2_PLACEMENT_3D('',#36084,#23646,#23647);
#19281=AXIS2_PLACEMENT_3D('',#36088,#23649,#23650);
#19282=AXIS2_PLACEMENT_3D('',#36090,#23652,#23653);
#19283=AXIS2_PLACEMENT_3D('',#36111,#23663,#23664);
#19284=AXIS2_PLACEMENT_3D('',#36120,#23669,#23670);
#19285=AXIS2_PLACEMENT_3D('',#36133,#23677,#23678);
#19286=AXIS2_PLACEMENT_3D('',#36137,#23680,#23681);
#19287=AXIS2_PLACEMENT_3D('',#36140,#23683,#23684);
#19288=AXIS2_PLACEMENT_3D('',#36143,#23686,#23687);
#19289=AXIS2_PLACEMENT_3D('',#36147,#23689,#23690);
#19290=AXIS2_PLACEMENT_3D('',#36149,#23692,#23693);
#19291=AXIS2_PLACEMENT_3D('',#36151,#23695,#23696);
#19292=AXIS2_PLACEMENT_3D('',#36153,#23698,#23699);
#19293=AXIS2_PLACEMENT_3D('',#36155,#23701,#23702);
#19294=AXIS2_PLACEMENT_3D('',#36157,#23704,#23705);
#19295=AXIS2_PLACEMENT_3D('',#36159,#23707,#23708);
#19296=AXIS2_PLACEMENT_3D('',#36161,#23710,#23711);
#19297=AXIS2_PLACEMENT_3D('',#36163,#23713,#23714);
#19298=AXIS2_PLACEMENT_3D('',#36165,#23716,#23717);
#19299=AXIS2_PLACEMENT_3D('',#36167,#23718,#23719);
#19300=AXIS2_PLACEMENT_3D('',#36171,#23721,#23722);
#19301=AXIS2_PLACEMENT_3D('',#36176,#23725,#23726);
#19302=AXIS2_PLACEMENT_3D('',#36179,#23728,#23729);
#19303=AXIS2_PLACEMENT_3D('',#36180,#23730,#23731);
#19304=AXIS2_PLACEMENT_3D('',#36184,#23733,#23734);
#19305=AXIS2_PLACEMENT_3D('',#36187,#23736,#23737);
#19306=AXIS2_PLACEMENT_3D('',#36191,#23739,#23740);
#19307=AXIS2_PLACEMENT_3D('',#36195,#23743,#23744);
#19308=AXIS2_PLACEMENT_3D('',#36196,#23745,#23746);
#19309=AXIS2_PLACEMENT_3D('',#36201,#23748,#23749);
#19310=AXIS2_PLACEMENT_3D('',#36206,#23752,#23753);
#19311=AXIS2_PLACEMENT_3D('',#36209,#23755,#23756);
#19312=AXIS2_PLACEMENT_3D('',#36210,#23757,#23758);
#19313=AXIS2_PLACEMENT_3D('',#36211,#23759,#23760);
#19314=AXIS2_PLACEMENT_3D('',#36213,#23762,#23763);
#19315=AXIS2_PLACEMENT_3D('',#36216,#23766,#23767);
#19316=AXIS2_PLACEMENT_3D('',#36219,#23770,#23771);
#19317=AXIS2_PLACEMENT_3D('',#36221,#23773,#23774);
#19318=AXIS2_PLACEMENT_3D('',#36222,#23775,#23776);
#19319=AXIS2_PLACEMENT_3D('',#36223,#23777,#23778);
#19320=AXIS2_PLACEMENT_3D('',#36224,#23779,#23780);
#19321=AXIS2_PLACEMENT_3D('',#36225,#23781,#23782);
#19322=AXIS2_PLACEMENT_3D('',#36227,#23784,#23785);
#19323=AXIS2_PLACEMENT_3D('',#36230,#23788,#23789);
#19324=AXIS2_PLACEMENT_3D('',#36233,#23792,#23793);
#19325=AXIS2_PLACEMENT_3D('',#36235,#23795,#23796);
#19326=AXIS2_PLACEMENT_3D('',#36236,#23797,#23798);
#19327=AXIS2_PLACEMENT_3D('',#36237,#23799,#23800);
#19328=AXIS2_PLACEMENT_3D('',#36238,#23801,#23802);
#19329=AXIS2_PLACEMENT_3D('',#36239,#23803,#23804);
#19330=AXIS2_PLACEMENT_3D('',#36240,#23805,#23806);
#19331=AXIS2_PLACEMENT_3D('',#36241,#23807,#23808);
#19332=AXIS2_PLACEMENT_3D('',#36247,#23812,#23813);
#19333=AXIS2_PLACEMENT_3D('',#36251,#23816,#23817);
#19334=AXIS2_PLACEMENT_3D('',#36255,#23820,#23821);
#19335=AXIS2_PLACEMENT_3D('',#36259,#23824,#23825);
#19336=AXIS2_PLACEMENT_3D('',#36263,#23828,#23829);
#19337=AXIS2_PLACEMENT_3D('',#36265,#23831,#23832);
#19338=AXIS2_PLACEMENT_3D('',#36278,#23839,#23840);
#19339=AXIS2_PLACEMENT_3D('',#36279,#23841,#23842);
#19340=AXIS2_PLACEMENT_3D('',#36280,#23843,#23844);
#19341=AXIS2_PLACEMENT_3D('',#36281,#23845,#23846);
#19342=AXIS2_PLACEMENT_3D('',#36282,#23847,#23848);
#19343=AXIS2_PLACEMENT_3D('',#36283,#23849,#23850);
#19344=AXIS2_PLACEMENT_3D('',#36284,#23851,#23852);
#19345=AXIS2_PLACEMENT_3D('',#36285,#23853,#23854);
#19346=AXIS2_PLACEMENT_3D('',#36286,#23855,#23856);
#19347=AXIS2_PLACEMENT_3D('',#36287,#23857,#23858);
#19348=AXIS2_PLACEMENT_3D('',#36288,#23859,#23860);
#19349=AXIS2_PLACEMENT_3D('',#36289,#23861,#23862);
#19350=AXIS2_PLACEMENT_3D('',#36290,#23863,#23864);
#19351=AXIS2_PLACEMENT_3D('',#36292,#23866,#23867);
#19352=AXIS2_PLACEMENT_3D('',#36294,#23868,#23869);
#19353=AXIS2_PLACEMENT_3D('',#36295,#23870,#23871);
#19354=AXIS2_PLACEMENT_3D('',#36298,#23873,#23874);
#19355=AXIS2_PLACEMENT_3D('',#36299,#23875,#23876);
#19356=AXIS2_PLACEMENT_3D('',#36308,#23881,#23882);
#19357=AXIS2_PLACEMENT_3D('',#36310,#23883,#23884);
#19358=AXIS2_PLACEMENT_3D('',#36313,#23886,#23887);
#19359=AXIS2_PLACEMENT_3D('',#36314,#23888,#23889);
#19360=AXIS2_PLACEMENT_3D('',#36320,#23893,#23894);
#19361=AXIS2_PLACEMENT_3D('',#36326,#23898,#23899);
#19362=AXIS2_PLACEMENT_3D('',#36332,#23903,#23904);
#19363=AXIS2_PLACEMENT_3D('',#36338,#23908,#23909);
#19364=AXIS2_PLACEMENT_3D('',#36344,#23913,#23914);
#19365=AXIS2_PLACEMENT_3D('',#36350,#23918,#23919);
#19366=AXIS2_PLACEMENT_3D('',#36356,#23923,#23924);
#19367=AXIS2_PLACEMENT_3D('',#36362,#23928,#23929);
#19368=AXIS2_PLACEMENT_3D('',#36368,#23933,#23934);
#19369=AXIS2_PLACEMENT_3D('',#36374,#23938,#23939);
#19370=AXIS2_PLACEMENT_3D('',#36380,#23943,#23944);
#19371=AXIS2_PLACEMENT_3D('',#36386,#23948,#23949);
#19372=AXIS2_PLACEMENT_3D('',#36392,#23953,#23954);
#19373=AXIS2_PLACEMENT_3D('',#36398,#23958,#23959);
#19374=AXIS2_PLACEMENT_3D('',#36404,#23963,#23964);
#19375=AXIS2_PLACEMENT_3D('',#36410,#23968,#23969);
#19376=AXIS2_PLACEMENT_3D('',#36416,#23973,#23974);
#19377=AXIS2_PLACEMENT_3D('',#36422,#23978,#23979);
#19378=AXIS2_PLACEMENT_3D('',#36428,#23983,#23984);
#19379=AXIS2_PLACEMENT_3D('',#36434,#23988,#23989);
#19380=AXIS2_PLACEMENT_3D('',#36440,#23993,#23994);
#19381=AXIS2_PLACEMENT_3D('',#36446,#23998,#23999);
#19382=AXIS2_PLACEMENT_3D('',#36452,#24003,#24004);
#19383=AXIS2_PLACEMENT_3D('',#36458,#24008,#24009);
#19384=AXIS2_PLACEMENT_3D('',#36464,#24013,#24014);
#19385=AXIS2_PLACEMENT_3D('',#36470,#24018,#24019);
#19386=AXIS2_PLACEMENT_3D('',#36476,#24023,#24024);
#19387=AXIS2_PLACEMENT_3D('',#36482,#24028,#24029);
#19388=AXIS2_PLACEMENT_3D('',#36488,#24033,#24034);
#19389=AXIS2_PLACEMENT_3D('',#36494,#24038,#24039);
#19390=AXIS2_PLACEMENT_3D('',#36500,#24043,#24044);
#19391=AXIS2_PLACEMENT_3D('',#36506,#24048,#24049);
#19392=AXIS2_PLACEMENT_3D('',#36512,#24053,#24054);
#19393=AXIS2_PLACEMENT_3D('',#36518,#24058,#24059);
#19394=AXIS2_PLACEMENT_3D('',#36524,#24063,#24064);
#19395=AXIS2_PLACEMENT_3D('',#36530,#24068,#24069);
#19396=AXIS2_PLACEMENT_3D('',#36536,#24073,#24074);
#19397=AXIS2_PLACEMENT_3D('',#36542,#24078,#24079);
#19398=AXIS2_PLACEMENT_3D('',#36544,#24080,#24081);
#19399=AXIS2_PLACEMENT_3D('',#36546,#24082,#24083);
#19400=AXIS2_PLACEMENT_3D('',#36548,#24085,#24086);
#19401=AXIS2_PLACEMENT_3D('',#36554,#24090,#24091);
#19402=AXIS2_PLACEMENT_3D('',#36557,#24094,#24095);
#19403=AXIS2_PLACEMENT_3D('',#36558,#24096,#24097);
#19404=AXIS2_PLACEMENT_3D('',#36559,#24098,#24099);
#23357=DIRECTION('axis',(0.,0.,1.));
#23358=DIRECTION('refdir',(1.,0.,0.));
#23359=DIRECTION('center_axis',(0.,0.,1.));
#23360=DIRECTION('ref_axis',(1.,0.,0.));
#23361=DIRECTION('center_axis',(0.,0.,1.));
#23362=DIRECTION('ref_axis',(1.,0.,0.));
#23363=DIRECTION('center_axis',(0.,0.,-1.));
#23364=DIRECTION('ref_axis',(1.,0.,0.));
#23365=DIRECTION('center_axis',(0.,0.,1.));
#23366=DIRECTION('ref_axis',(1.,0.,0.));
#23367=DIRECTION('center_axis',(0.,0.,1.));
#23368=DIRECTION('ref_axis',(1.,0.,0.));
#23369=DIRECTION('center_axis',(0.,0.,1.));
#23370=DIRECTION('ref_axis',(1.,0.,0.));
#23371=DIRECTION('',(0.707106781186548,8.65956056235494E-17,-0.707106781186547));
#23372=DIRECTION('center_axis',(0.,0.,1.));
#23373=DIRECTION('ref_axis',(0.990993942369174,-0.133906707029938,0.));
#23374=DIRECTION('',(0.,0.,1.));
#23375=DIRECTION('center_axis',(0.,0.,-1.));
#23376=DIRECTION('ref_axis',(-1.,0.,0.));
#23377=DIRECTION('',(0.,0.,-1.));
#23378=DIRECTION('',(0.,0.,-1.));
#23379=DIRECTION('center_axis',(0.,0.,-1.));
#23380=DIRECTION('ref_axis',(1.,0.,0.));
#23381=DIRECTION('center_axis',(0.,0.,-1.));
#23382=DIRECTION('ref_axis',(-1.,0.,0.));
#23383=DIRECTION('',(0.,0.,-1.));
#23384=DIRECTION('center_axis',(0.,0.,-1.));
#23385=DIRECTION('ref_axis',(-1.,0.,0.));
#23386=DIRECTION('',(0.,0.,-1.));
#23387=DIRECTION('center_axis',(0.,0.,-1.));
#23388=DIRECTION('ref_axis',(-1.,0.,0.));
#23389=DIRECTION('',(0.,0.,-1.));
#23390=DIRECTION('center_axis',(0.,0.,-1.));
#23391=DIRECTION('ref_axis',(-1.,0.,0.));
#23392=DIRECTION('',(0.,0.,-1.));
#23393=DIRECTION('center_axis',(0.,0.,-1.));
#23394=DIRECTION('ref_axis',(-1.,0.,0.));
#23395=DIRECTION('',(0.,0.,-1.));
#23396=DIRECTION('center_axis',(0.,0.,-1.));
#23397=DIRECTION('ref_axis',(-1.,0.,0.));
#23398=DIRECTION('',(0.,0.,-1.));
#23399=DIRECTION('center_axis',(0.,0.,-1.));
#23400=DIRECTION('ref_axis',(-1.,0.,0.));
#23401=DIRECTION('',(0.,0.,-1.));
#23402=DIRECTION('center_axis',(0.,0.,-1.));
#23403=DIRECTION('ref_axis',(-1.,0.,0.));
#23404=DIRECTION('',(0.,0.,-1.));
#23405=DIRECTION('center_axis',(0.,0.,-1.));
#23406=DIRECTION('ref_axis',(-1.,0.,0.));
#23407=DIRECTION('',(0.,0.,-1.));
#23408=DIRECTION('center_axis',(0.,0.,-1.));
#23409=DIRECTION('ref_axis',(-1.,0.,0.));
#23410=DIRECTION('',(0.,0.,-1.));
#23411=DIRECTION('center_axis',(0.,0.,-1.));
#23412=DIRECTION('ref_axis',(-1.,0.,0.));
#23413=DIRECTION('',(0.,0.,-1.));
#23414=DIRECTION('center_axis',(0.,0.,-1.));
#23415=DIRECTION('ref_axis',(-1.,0.,0.));
#23416=DIRECTION('',(0.,0.,-1.));
#23417=DIRECTION('center_axis',(0.,0.,-1.));
#23418=DIRECTION('ref_axis',(-1.,0.,0.));
#23419=DIRECTION('',(0.,0.,-1.));
#23420=DIRECTION('center_axis',(0.,0.,1.));
#23421=DIRECTION('ref_axis',(1.,0.,0.));
#23422=DIRECTION('center_axis',(0.,0.,1.));
#23423=DIRECTION('ref_axis',(1.,-7.27351010247249E-15,0.));
#23424=DIRECTION('',(0.,0.,-1.));
#23425=DIRECTION('',(0.,0.,1.));
#23426=DIRECTION('center_axis',(0.,0.,1.));
#23427=DIRECTION('ref_axis',(1.,-7.27351010247249E-15,0.));
#23428=DIRECTION('',(0.,0.,-1.));
#23429=DIRECTION('center_axis',(0.,0.,1.));
#23430=DIRECTION('ref_axis',(1.,-7.27351010247249E-15,0.));
#23431=DIRECTION('',(0.,0.,-1.));
#23432=DIRECTION('center_axis',(0.,0.,1.));
#23433=DIRECTION('ref_axis',(1.,-7.27351010247249E-15,0.));
#23434=DIRECTION('',(0.,0.,-1.));
#23435=DIRECTION('center_axis',(0.,0.,1.));
#23436=DIRECTION('ref_axis',(1.,-7.27351010247249E-15,0.));
#23437=DIRECTION('',(0.,0.,-1.));
#23438=DIRECTION('center_axis',(0.,0.,1.));
#23439=DIRECTION('ref_axis',(1.,-7.27351010247249E-15,0.));
#23440=DIRECTION('',(0.,0.,-1.));
#23441=DIRECTION('center_axis',(0.,0.,1.));
#23442=DIRECTION('ref_axis',(1.,-7.27351010247249E-15,0.));
#23443=DIRECTION('',(0.,0.,-1.));
#23444=DIRECTION('center_axis',(0.,0.,1.));
#23445=DIRECTION('ref_axis',(1.,-7.27351010247249E-15,0.));
#23446=DIRECTION('',(0.,0.,-1.));
#23447=DIRECTION('center_axis',(0.,0.,1.));
#23448=DIRECTION('ref_axis',(1.,-7.27351010247249E-15,0.));
#23449=DIRECTION('',(0.,0.,-1.));
#23450=DIRECTION('center_axis',(0.,0.,1.));
#23451=DIRECTION('ref_axis',(1.,-7.27351010247249E-15,0.));
#23452=DIRECTION('',(0.,0.,-1.));
#23453=DIRECTION('center_axis',(0.,0.,1.));
#23454=DIRECTION('ref_axis',(1.,-7.27351010247249E-15,0.));
#23455=DIRECTION('',(0.,0.,-1.));
#23456=DIRECTION('center_axis',(0.,0.,1.));
#23457=DIRECTION('ref_axis',(1.,-7.27351010247249E-15,0.));
#23458=DIRECTION('',(0.,0.,-1.));
#23459=DIRECTION('center_axis',(0.,0.,1.));
#23460=DIRECTION('ref_axis',(1.,-7.27351010247249E-15,0.));
#23461=DIRECTION('',(0.,0.,-1.));
#23462=DIRECTION('center_axis',(0.,0.,1.));
#23463=DIRECTION('ref_axis',(1.,-7.27351010247249E-15,0.));
#23464=DIRECTION('',(0.,0.,-1.));
#23465=DIRECTION('',(0.,0.,-1.));
#23466=DIRECTION('center_axis',(0.,0.,1.));
#23467=DIRECTION('ref_axis',(1.,0.,0.));
#23468=DIRECTION('center_axis',(0.,0.,1.));
#23469=DIRECTION('ref_axis',(1.,0.,0.));
#23470=DIRECTION('',(0.,0.,-1.));
#23471=DIRECTION('center_axis',(0.,0.,1.));
#23472=DIRECTION('ref_axis',(0.999820197862873,-0.0189623823779183,0.));
#23473=DIRECTION('center_axis',(0.,0.,1.));
#23474=DIRECTION('ref_axis',(1.,0.,0.));
#23475=DIRECTION('center_axis',(0.,0.,-1.));
#23476=DIRECTION('ref_axis',(-0.990993942369175,0.133906707029934,0.));
#23477=DIRECTION('',(0.,0.,-1.));
#23478=DIRECTION('center_axis',(0.,0.,1.));
#23479=DIRECTION('ref_axis',(1.,0.,0.));
#23480=DIRECTION('center_axis',(0.,0.,-1.));
#23481=DIRECTION('ref_axis',(-1.,0.,0.));
#23482=DIRECTION('center_axis',(0.,0.,1.));
#23483=DIRECTION('ref_axis',(0.990993942369174,-0.133906707029939,0.));
#23484=DIRECTION('',(0.,0.,1.));
#23485=DIRECTION('center_axis',(0.,0.,-1.));
#23486=DIRECTION('ref_axis',(1.,0.,0.));
#23487=DIRECTION('center_axis',(0.,0.,1.));
#23488=DIRECTION('ref_axis',(1.,0.,0.));
#23489=DIRECTION('center_axis',(0.,0.,1.));
#23490=DIRECTION('ref_axis',(1.,0.,0.));
#23491=DIRECTION('center_axis',(0.,-1.,0.));
#23492=DIRECTION('ref_axis',(-1.,0.,0.));
#23493=DIRECTION('center_axis',(0.,0.,-1.));
#23494=DIRECTION('ref_axis',(1.,0.,0.));
#23495=DIRECTION('center_axis',(0.,0.,-1.));
#23496=DIRECTION('ref_axis',(1.,0.,0.));
#23497=DIRECTION('center_axis',(0.,0.,1.));
#23498=DIRECTION('ref_axis',(1.,0.,0.));
#23499=DIRECTION('center_axis',(0.,0.,1.));
#23500=DIRECTION('ref_axis',(1.,0.,0.));
#23501=DIRECTION('center_axis',(0.,0.,1.));
#23502=DIRECTION('ref_axis',(1.,0.,0.));
#23503=DIRECTION('center_axis',(0.,-1.,0.));
#23504=DIRECTION('ref_axis',(-1.,0.,0.));
#23505=DIRECTION('center_axis',(0.,0.,-1.));
#23506=DIRECTION('ref_axis',(1.,0.,0.));
#23507=DIRECTION('center_axis',(0.,0.,1.));
#23508=DIRECTION('ref_axis',(1.,0.,0.));
#23509=DIRECTION('center_axis',(0.,0.,1.));
#23510=DIRECTION('ref_axis',(1.,0.,0.));
#23511=DIRECTION('center_axis',(0.,0.,1.));
#23512=DIRECTION('ref_axis',(1.,0.,0.));
#23513=DIRECTION('center_axis',(0.,-1.,0.));
#23514=DIRECTION('ref_axis',(-1.,0.,0.));
#23515=DIRECTION('center_axis',(0.,0.,-1.));
#23516=DIRECTION('ref_axis',(1.,0.,0.));
#23517=DIRECTION('center_axis',(0.,0.,1.));
#23518=DIRECTION('ref_axis',(1.,0.,0.));
#23519=DIRECTION('center_axis',(0.,0.,1.));
#23520=DIRECTION('ref_axis',(1.,0.,0.));
#23521=DIRECTION('center_axis',(0.,-1.,0.));
#23522=DIRECTION('ref_axis',(-1.,0.,0.));
#23523=DIRECTION('center_axis',(0.,0.,-1.));
#23524=DIRECTION('ref_axis',(1.,0.,0.));
#23525=DIRECTION('center_axis',(0.,0.,-1.));
#23526=DIRECTION('ref_axis',(1.,0.,0.));
#23527=DIRECTION('center_axis',(0.,0.,-1.));
#23528=DIRECTION('ref_axis',(-1.,0.,0.));
#23529=DIRECTION('',(0.,0.,-1.));
#23530=DIRECTION('center_axis',(0.,0.,-1.));
#23531=DIRECTION('ref_axis',(-1.,0.,0.));
#23532=DIRECTION('',(0.,0.,1.));
#23533=DIRECTION('center_axis',(0.,0.,1.));
#23534=DIRECTION('ref_axis',(1.,0.,0.));
#23535=DIRECTION('center_axis',(0.,0.,1.));
#23536=DIRECTION('ref_axis',(1.,0.,0.));
#23537=DIRECTION('center_axis',(0.,0.,1.));
#23538=DIRECTION('ref_axis',(1.,0.,0.));
#23539=DIRECTION('center_axis',(0.,0.,1.));
#23540=DIRECTION('ref_axis',(1.,0.,0.));
#23541=DIRECTION('center_axis',(0.,0.,1.));
#23542=DIRECTION('ref_axis',(1.,0.,0.));
#23543=DIRECTION('center_axis',(0.,0.,1.));
#23544=DIRECTION('ref_axis',(-0.925614790208249,-0.378466986866409,0.));
#23545=DIRECTION('center_axis',(0.,0.,1.));
#23546=DIRECTION('ref_axis',(1.,0.,0.));
#23547=DIRECTION('center_axis',(0.,0.,1.));
#23548=DIRECTION('ref_axis',(1.,0.,0.));
#23549=DIRECTION('',(0.,0.,1.));
#23550=DIRECTION('',(-0.866025403784439,0.,-0.499999999999999));
#23551=DIRECTION('',(0.866025403784439,0.,0.499999999999999));
#23552=DIRECTION('center_axis',(0.,0.,1.));
#23553=DIRECTION('ref_axis',(1.,-7.27351010247249E-15,0.));
#23554=DIRECTION('',(0.866025403784439,0.,-0.499999999999999));
#23555=DIRECTION('',(-0.866025403784439,0.,0.499999999999999));
#23556=DIRECTION('center_axis',(0.,1.,0.));
#23557=DIRECTION('ref_axis',(1.,0.,0.));
#23558=DIRECTION('',(0.,0.,-1.));
#23559=DIRECTION('center_axis',(0.,-1.,0.));
#23560=DIRECTION('ref_axis',(0.,0.,-1.));
#23561=DIRECTION('center_axis',(0.,0.,1.));
#23562=DIRECTION('ref_axis',(1.,1.11022302462528E-14,0.));
#23563=DIRECTION('center_axis',(0.,0.,-1.));
#23564=DIRECTION('ref_axis',(1.,0.,0.));
#23565=DIRECTION('center_axis',(0.,0.,1.));
#23566=DIRECTION('ref_axis',(1.,0.,0.));
#23567=DIRECTION('',(-0.707106781186549,-8.65956056235495E-17,0.707106781186546));
#23568=DIRECTION('center_axis',(0.,0.,-1.));
#23569=DIRECTION('ref_axis',(1.,0.,0.));
#23570=DIRECTION('center_axis',(0.,0.,-1.));
#23571=DIRECTION('ref_axis',(-1.,0.,0.));
#23572=DIRECTION('',(0.707106781186545,-8.6595605623549E-17,-0.70710678118655));
#23573=DIRECTION('center_axis',(0.,0.,-1.));
#23574=DIRECTION('ref_axis',(-1.,0.,0.));
#23575=DIRECTION('center_axis',(0.,0.,-1.));
#23576=DIRECTION('ref_axis',(1.,0.,0.));
#23577=DIRECTION('center_axis',(0.,0.,-1.));
#23578=DIRECTION('ref_axis',(1.,0.,0.));
#23579=DIRECTION('',(-0.707106781186545,8.6595605623549E-17,0.70710678118655));
#23580=DIRECTION('center_axis',(0.,0.,1.));
#23581=DIRECTION('ref_axis',(1.,0.,0.));
#23582=DIRECTION('center_axis',(0.,0.,1.));
#23583=DIRECTION('ref_axis',(1.,0.,0.));
#23584=DIRECTION('center_axis',(0.,0.,-1.));
#23585=DIRECTION('ref_axis',(-1.,0.,0.));
#23586=DIRECTION('center_axis',(0.,0.,1.));
#23587=DIRECTION('ref_axis',(1.,0.,0.));
#23588=DIRECTION('center_axis',(0.,0.,-1.));
#23589=DIRECTION('ref_axis',(-0.990993942369175,0.133906707029934,0.));
#23590=DIRECTION('center_axis',(0.,0.,-1.));
#23591=DIRECTION('ref_axis',(-0.990993942369175,0.133906707029935,0.));
#23592=DIRECTION('center_axis',(-0.133906707029936,-0.990993942369174,0.));
#23593=DIRECTION('ref_axis',(0.990993942369174,-0.133906707029936,0.));
#23594=DIRECTION('center_axis',(0.,0.,1.));
#23595=DIRECTION('ref_axis',(-0.990993942369175,0.133906707029936,0.));
#23596=DIRECTION('center_axis',(0.,0.,-1.));
#23597=DIRECTION('ref_axis',(-0.990993942369175,0.133906707029934,0.));
#23598=DIRECTION('center_axis',(0.,0.,-1.));
#23599=DIRECTION('ref_axis',(-0.990993942369175,0.133906707029936,0.));
#23600=DIRECTION('center_axis',(-0.133906707029936,-0.990993942369174,0.));
#23601=DIRECTION('ref_axis',(0.990993942369174,-0.133906707029936,0.));
#23602=DIRECTION('center_axis',(0.,0.,1.));
#23603=DIRECTION('ref_axis',(-0.990993942369175,0.133906707029935,0.));
#23604=DIRECTION('center_axis',(0.,0.,-1.));
#23605=DIRECTION('ref_axis',(-0.990993942369175,0.133906707029935,0.));
#23606=DIRECTION('',(0.,0.,1.));
#23607=DIRECTION('center_axis',(0.,0.,1.));
#23608=DIRECTION('ref_axis',(0.990993942369175,-0.133906707029936,0.));
#23609=DIRECTION('center_axis',(0.,0.,-1.));
#23610=DIRECTION('ref_axis',(-0.990993942369175,0.133906707029936,0.));
#23611=DIRECTION('',(0.,0.,-1.));
#23612=DIRECTION('center_axis',(0.,0.,1.));
#23613=DIRECTION('ref_axis',(0.990993942369175,-0.133906707029935,0.));
#23614=DIRECTION('center_axis',(0.,0.,-1.));
#23615=DIRECTION('ref_axis',(-0.990993942369175,0.133906707029935,0.));
#23616=DIRECTION('',(0.,0.,1.));
#23617=DIRECTION('center_axis',(0.,0.,1.));
#23618=DIRECTION('ref_axis',(-0.990993942369175,0.133906707029935,0.));
#23619=DIRECTION('',(0.,0.,1.));
#23620=DIRECTION('center_axis',(0.,0.,-1.));
#23621=DIRECTION('ref_axis',(-0.990993942369175,0.133906707029934,0.));
#23622=DIRECTION('center_axis',(0.,0.,1.));
#23623=DIRECTION('ref_axis',(-0.990993942369175,0.133906707029934,0.));
#23624=DIRECTION('',(0.,0.,1.));
#23625=DIRECTION('center_axis',(0.,0.,-1.));
#23626=DIRECTION('ref_axis',(-0.990993942369175,0.133906707029934,0.));
#23627=DIRECTION('center_axis',(0.,0.,-1.));
#23628=DIRECTION('ref_axis',(-0.990993942369175,0.133906707029936,0.));
#23629=DIRECTION('',(-0.434556986477371,-0.900644339072703,0.));
#23630=DIRECTION('',(-0.986071242772467,0.166323492559414,0.));
#23631=DIRECTION('',(0.166323492559414,0.986071242772467,0.));
#23632=DIRECTION('',(-0.461967687527403,0.886896755930804,0.));
#23633=DIRECTION('',(-0.573632924010497,0.819112488301312,0.));
#23634=DIRECTION('',(-0.909238313074883,0.41627597821246,0.));
#23635=DIRECTION('',(-0.947556814961333,0.319587362735659,0.));
#23636=DIRECTION('center_axis',(0.,0.,-1.));
#23637=DIRECTION('ref_axis',(-0.990993942369174,0.133906707029937,0.));
#23638=DIRECTION('',(0.705703477039673,-0.708507305886196,0.));
#23639=DIRECTION('',(0.923615773230652,-0.383319583949927,0.));
#23640=DIRECTION('',(0.990993942369174,-0.133906707029936,0.));
#23641=DIRECTION('',(0.885144693704452,0.465315883252282,0.));
#23642=DIRECTION('',(0.662959137150796,-0.748655583341414,0.));
#23643=DIRECTION('',(-0.691641091103085,-0.722241373155633,0.));
#23644=DIRECTION('center_axis',(0.,0.,1.));
#23645=DIRECTION('ref_axis',(0.990993942369175,-0.133906707029936,0.));
#23646=DIRECTION('center_axis',(0.,0.,-1.));
#23647=DIRECTION('ref_axis',(-0.990993942369175,0.133906707029936,0.));
#23648=DIRECTION('',(0.,0.,1.));
#23649=DIRECTION('center_axis',(0.,0.,1.));
#23650=DIRECTION('ref_axis',(0.990993942369175,-0.133906707029936,0.));
#23651=DIRECTION('',(0.,0.,1.));
#23652=DIRECTION('center_axis',(0.,0.,-1.));
#23653=DIRECTION('ref_axis',(-0.990993942369175,0.133906707029936,0.));
#23654=DIRECTION('',(0.166323492559414,0.986071242772467,0.));
#23655=DIRECTION('',(0.986071242772467,-0.166323492559414,0.));
#23656=DIRECTION('',(-0.434556986477371,-0.900644339072703,0.));
#23657=DIRECTION('',(-0.691641091103085,-0.722241373155633,0.));
#23658=DIRECTION('',(-0.639459501656208,0.768824782210871,0.));
#23659=DIRECTION('',(0.885144693704452,0.465315883252282,0.));
#23660=DIRECTION('',(0.990993942369174,-0.133906707029936,0.));
#23661=DIRECTION('',(0.923615773230652,-0.383319583949927,0.));
#23662=DIRECTION('',(0.705703477039673,-0.708507305886196,0.));
#23663=DIRECTION('center_axis',(0.,0.,-1.));
#23664=DIRECTION('ref_axis',(-0.990993942369174,0.133906707029937,0.));
#23665=DIRECTION('',(-0.947556814961333,0.319587362735659,0.));
#23666=DIRECTION('',(-0.909238313074883,0.41627597821246,0.));
#23667=DIRECTION('',(-0.573632924010497,0.819112488301312,0.));
#23668=DIRECTION('',(-0.461967687527403,0.886896755930804,0.));
#23669=DIRECTION('center_axis',(0.,0.,-1.));
#23670=DIRECTION('ref_axis',(-0.990993942369174,0.133906707029938,0.));
#23671=DIRECTION('',(0.297235194420542,0.954804293663252,0.));
#23672=DIRECTION('',(0.975502371165105,0.219988917564631,0.));
#23673=DIRECTION('',(0.678267176744562,-0.734815376098623,0.));
#23674=DIRECTION('',(-0.297235194420543,-0.954804293663252,0.));
#23675=DIRECTION('',(-0.975502371165106,-0.219988917564629,0.));
#23676=DIRECTION('',(-0.678267176744562,0.734815376098623,0.));
#23677=DIRECTION('center_axis',(0.986071242772468,-0.166323492559414,0.));
#23678=DIRECTION('ref_axis',(0.166323492559414,0.986071242772467,0.));
#23679=DIRECTION('',(-0.166323492559414,-0.986071242772467,0.));
#23680=DIRECTION('center_axis',(-0.986071242772467,0.166323492559414,0.));
#23681=DIRECTION('ref_axis',(-0.166323492559414,-0.986071242772467,0.));
#23682=DIRECTION('',(0.,0.,-1.));
#23683=DIRECTION('center_axis',(0.986071242772467,-0.166323492559414,0.));
#23684=DIRECTION('ref_axis',(-0.166323492559414,-0.986071242772467,0.));
#23685=DIRECTION('',(0.,0.,1.));
#23686=DIRECTION('center_axis',(-0.986071242772467,0.166323492559414,1.02716263700652E-30));
#23687=DIRECTION('ref_axis',(-0.166323492559414,-0.986071242772467,-1.35177217172879E-45));
#23688=DIRECTION('',(0.,0.,-1.));
#23689=DIRECTION('center_axis',(0.986071242772467,-0.166323492559414,0.));
#23690=DIRECTION('ref_axis',(-0.166323492559414,-0.986071242772467,0.));
#23691=DIRECTION('',(0.166323492559414,0.986071242772467,0.));
#23692=DIRECTION('center_axis',(0.886896755930804,0.461967687527403,0.));
#23693=DIRECTION('ref_axis',(0.,0.,-1.));
#23694=DIRECTION('',(0.,0.,1.));
#23695=DIRECTION('center_axis',(0.819112488301313,0.573632924010497,0.));
#23696=DIRECTION('ref_axis',(0.,0.,-1.));
#23697=DIRECTION('',(0.,0.,1.));
#23698=DIRECTION('center_axis',(0.41627597821246,0.909238313074883,0.));
#23699=DIRECTION('ref_axis',(0.,0.,-1.));
#23700=DIRECTION('',(0.,0.,1.));
#23701=DIRECTION('center_axis',(0.319587362735659,0.947556814961333,0.));
#23702=DIRECTION('ref_axis',(0.,0.,-1.));
#23703=DIRECTION('',(0.,0.,1.));
#23704=DIRECTION('center_axis',(0.,0.,1.));
#23705=DIRECTION('ref_axis',(-0.803690873252051,0.595047040368538,0.));
#23706=DIRECTION('',(0.,0.,1.));
#23707=DIRECTION('center_axis',(-0.708507305886196,-0.705703477039673,0.));
#23708=DIRECTION('ref_axis',(0.,0.,1.));
#23709=DIRECTION('',(0.,0.,1.));
#23710=DIRECTION('center_axis',(-0.383319583949927,-0.923615773230652,0.));
#23711=DIRECTION('ref_axis',(0.,0.,1.));
#23712=DIRECTION('',(0.,0.,1.));
#23713=DIRECTION('center_axis',(-0.133906707029936,-0.990993942369175,0.));
#23714=DIRECTION('ref_axis',(0.,0.,1.));
#23715=DIRECTION('',(0.,0.,1.));
#23716=DIRECTION('center_axis',(0.465315883252282,-0.885144693704452,0.));
#23717=DIRECTION('ref_axis',(0.885144693704452,0.465315883252282,0.));
#23718=DIRECTION('center_axis',(-0.465315883252296,0.885144693704445,-2.1507739644884E-14));
#23719=DIRECTION('ref_axis',(0.885144693704445,0.465315883252296,-7.92224047828207E-11));
#23720=DIRECTION('',(0.,0.,1.));
#23721=DIRECTION('center_axis',(0.465315883252259,-0.885144693704465,-2.38928391774824E-14));
#23722=DIRECTION('ref_axis',(0.885144693704465,0.465315883252258,-1.11680359097547E-11));
#23723=DIRECTION('',(-0.885144693704452,-0.465315883252282,0.));
#23724=DIRECTION('',(0.885144693704452,0.465315883252282,0.));
#23725=DIRECTION('center_axis',(-0.465315883252314,0.885144693704436,-5.15404751531186E-14));
#23726=DIRECTION('ref_axis',(0.885144693704436,0.465315883252314,7.55878627128317E-11));
#23727=DIRECTION('',(0.,0.,1.));
#23728=DIRECTION('center_axis',(0.465315883252266,-0.885144693704461,-1.83477419639032E-14));
#23729=DIRECTION('ref_axis',(0.885144693704461,0.465315883252266,-5.12289412685469E-12));
#23730=DIRECTION('center_axis',(-0.722241373155633,0.691641091103085,0.));
#23731=DIRECTION('ref_axis',(0.,0.,1.));
#23732=DIRECTION('',(0.,0.,1.));
#23733=DIRECTION('center_axis',(0.722241373155643,-0.691641091103075,-1.34943523468737E-15));
#23734=DIRECTION('ref_axis',(0.691641091103075,0.722241373155643,-2.2903875502264E-10));
#23735=DIRECTION('',(0.,0.,1.));
#23736=DIRECTION('center_axis',(-0.72224137315561,0.691641091103109,3.34490341472713E-14));
#23737=DIRECTION('ref_axis',(0.691641091103109,0.72224137315561,-4.63418217506663E-10));
#23738=DIRECTION('',(0.,0.,1.));
#23739=DIRECTION('center_axis',(0.722241373155679,-0.691641091103037,7.1290365707807E-14));
#23740=DIRECTION('ref_axis',(0.691641091103036,0.722241373155679,4.52709546294639E-10));
#23741=DIRECTION('',(-0.691641091103085,-0.722241373155633,0.));
#23742=DIRECTION('',(0.691641091103085,0.722241373155633,0.));
#23743=DIRECTION('center_axis',(-0.722241373155636,0.691641091103082,-2.46271930330266E-14));
#23744=DIRECTION('ref_axis',(0.691641091103082,0.722241373155636,4.41696351613122E-10));
#23745=DIRECTION('center_axis',(-0.900644339072703,0.434556986477371,0.));
#23746=DIRECTION('ref_axis',(0.,0.,1.));
#23747=DIRECTION('',(0.,0.,-1.));
#23748=DIRECTION('center_axis',(0.900644339072708,-0.434556986477361,3.87104187789662E-16));
#23749=DIRECTION('ref_axis',(0.434556986477361,0.900644339072708,-1.76194029248825E-11));
#23750=DIRECTION('',(0.434556986477371,0.900644339072703,0.));
#23751=DIRECTION('',(-0.434556986477371,-0.900644339072703,0.));
#23752=DIRECTION('center_axis',(-0.900644339072692,0.434556986477393,2.41940117368536E-14));
#23753=DIRECTION('ref_axis',(0.434556986477393,0.900644339072692,9.15800115337473E-12));
#23754=DIRECTION('',(0.,0.,-1.));
#23755=DIRECTION('center_axis',(0.900644339072707,-0.434556986477363,1.7371300427058E-14));
#23756=DIRECTION('ref_axis',(0.434556986477363,0.900644339072707,-3.82265683540711E-11));
#23757=DIRECTION('center_axis',(-0.900644339072698,0.434556986477381,1.01614849294736E-14));
#23758=DIRECTION('ref_axis',(0.434556986477381,0.900644339072698,6.73661852370467E-11));
#23759=DIRECTION('center_axis',(0.,0.,-1.));
#23760=DIRECTION('ref_axis',(-0.990993942369175,0.133906707029936,0.));
#23761=DIRECTION('',(-0.662959137150796,0.748655583341414,0.));
#23762=DIRECTION('center_axis',(0.748655583341414,0.662959137150796,0.));
#23763=DIRECTION('ref_axis',(0.,0.,-1.));
#23764=DIRECTION('',(-0.662959137150796,0.748655583341414,0.));
#23765=DIRECTION('',(0.662959137150796,-0.748655583341414,0.));
#23766=DIRECTION('center_axis',(-0.768824782210871,-0.639459501656208,0.));
#23767=DIRECTION('ref_axis',(0.,0.,1.));
#23768=DIRECTION('',(-0.639459501656208,0.768824782210871,0.));
#23769=DIRECTION('',(0.639459501656208,-0.768824782210871,0.));
#23770=DIRECTION('center_axis',(0.,0.,-1.));
#23771=DIRECTION('ref_axis',(-0.990993942369175,0.133906707029936,0.));
#23772=DIRECTION('',(0.639459501656208,-0.768824782210871,0.));
#23773=DIRECTION('center_axis',(-0.639459501656208,0.768824782210872,0.));
#23774=DIRECTION('ref_axis',(0.768824782210872,0.639459501656208,0.));
#23775=DIRECTION('center_axis',(0.639459501656208,-0.768824782210871,0.));
#23776=DIRECTION('ref_axis',(-0.768824782210871,-0.639459501656208,0.));
#23777=DIRECTION('center_axis',(-0.662959137150795,0.748655583341415,0.));
#23778=DIRECTION('ref_axis',(0.748655583341415,0.662959137150795,0.));
#23779=DIRECTION('center_axis',(0.662959137150795,-0.748655583341415,0.));
#23780=DIRECTION('ref_axis',(-0.748655583341415,-0.662959137150795,0.));
#23781=DIRECTION('center_axis',(0.,0.,1.));
#23782=DIRECTION('ref_axis',(-0.133906707029936,-0.990993942369175,0.));
#23783=DIRECTION('',(-0.986071242772467,0.166323492559414,0.));
#23784=DIRECTION('center_axis',(-0.166323492559414,-0.986071242772468,0.));
#23785=DIRECTION('ref_axis',(0.,0.,1.));
#23786=DIRECTION('',(0.986071242772467,-0.166323492559414,0.));
#23787=DIRECTION('',(-0.986071242772467,0.166323492559414,0.));
#23788=DIRECTION('center_axis',(0.166323492559414,0.986071242772467,0.));
#23789=DIRECTION('ref_axis',(0.,0.,-1.));
#23790=DIRECTION('',(-0.986071242772467,0.166323492559414,0.));
#23791=DIRECTION('',(0.986071242772467,-0.166323492559414,0.));
#23792=DIRECTION('center_axis',(0.,0.,-1.));
#23793=DIRECTION('ref_axis',(-0.990993942369175,0.133906707029936,0.));
#23794=DIRECTION('',(0.986071242772467,-0.166323492559414,0.));
#23795=DIRECTION('center_axis',(0.986071242772468,-0.166323492559414,0.));
#23796=DIRECTION('ref_axis',(-0.166323492559414,-0.986071242772467,0.));
#23797=DIRECTION('center_axis',(0.986071242772467,-0.166323492559414,0.));
#23798=DIRECTION('ref_axis',(-0.166323492559414,-0.986071242772467,0.));
#23799=DIRECTION('center_axis',(0.986071242772467,-0.166323492559414,0.));
#23800=DIRECTION('ref_axis',(-0.166323492559414,-0.986071242772467,0.));
#23801=DIRECTION('center_axis',(-0.986071242772467,0.166323492559414,0.));
#23802=DIRECTION('ref_axis',(0.166323492559414,0.986071242772467,0.));
#23803=DIRECTION('center_axis',(0.,0.,-1.));
#23804=DIRECTION('ref_axis',(-0.990993942369175,0.133906707029936,0.));
#23805=DIRECTION('center_axis',(0.,0.,-1.));
#23806=DIRECTION('ref_axis',(-0.990993942369175,0.133906707029936,0.));
#23807=DIRECTION('center_axis',(0.219988917564632,-0.975502371165105,0.));
#23808=DIRECTION('ref_axis',(0.975502371165105,0.219988917564631,0.));
#23809=DIRECTION('',(0.,0.,1.));
#23810=DIRECTION('',(-0.975502371165105,-0.219988917564631,0.));
#23811=DIRECTION('',(0.,0.,1.));
#23812=DIRECTION('center_axis',(0.954804293663253,-0.297235194420542,0.));
#23813=DIRECTION('ref_axis',(0.297235194420542,0.954804293663252,0.));
#23814=DIRECTION('',(0.,0.,1.));
#23815=DIRECTION('',(-0.297235194420542,-0.954804293663252,0.));
#23816=DIRECTION('center_axis',(0.734815376098623,0.678267176744562,0.));
#23817=DIRECTION('ref_axis',(0.,0.,-1.));
#23818=DIRECTION('',(0.,0.,1.));
#23819=DIRECTION('',(0.678267176744562,-0.734815376098623,0.));
#23820=DIRECTION('center_axis',(-0.219988917564628,0.975502371165105,0.));
#23821=DIRECTION('ref_axis',(0.,0.,1.));
#23822=DIRECTION('',(0.,0.,1.));
#23823=DIRECTION('',(0.975502371165106,0.219988917564629,0.));
#23824=DIRECTION('center_axis',(-0.954804293663252,0.297235194420544,0.));
#23825=DIRECTION('ref_axis',(0.,0.,1.));
#23826=DIRECTION('',(0.,0.,1.));
#23827=DIRECTION('',(0.297235194420543,0.954804293663252,0.));
#23828=DIRECTION('center_axis',(-0.734815376098623,-0.678267176744562,0.));
#23829=DIRECTION('ref_axis',(0.,0.,1.));
#23830=DIRECTION('',(-0.678267176744562,0.734815376098623,0.));
#23831=DIRECTION('center_axis',(0.,0.,-1.));
#23832=DIRECTION('ref_axis',(-0.990993942369175,0.133906707029936,0.));
#23833=DIRECTION('',(-0.975502371165105,-0.219988917564628,0.));
#23834=DIRECTION('',(-0.297235194420543,-0.954804293663252,0.));
#23835=DIRECTION('',(0.678267176744562,-0.734815376098623,0.));
#23836=DIRECTION('',(0.975502371165105,0.219988917564631,0.));
#23837=DIRECTION('',(0.297235194420542,0.954804293663252,0.));
#23838=DIRECTION('',(-0.678267176744562,0.734815376098623,0.));
#23839=DIRECTION('center_axis',(-0.297235194420542,-0.954804293663253,0.));
#23840=DIRECTION('ref_axis',(-0.954804293663252,0.297235194420542,0.));
#23841=DIRECTION('center_axis',(-0.734815376098582,-0.678267176744606,5.08035781491937E-14));
#23842=DIRECTION('ref_axis',(0.678267176744606,-0.734815376098582,-3.83211898500117E-12));
#23843=DIRECTION('center_axis',(-0.219988917564645,0.975502371165102,5.18008130528868E-14));
#23844=DIRECTION('ref_axis',(0.975502371165102,0.219988917564645,-8.45195070037509E-12));
#23845=DIRECTION('center_axis',(0.678267176744561,-0.734815376098624,0.));
#23846=DIRECTION('ref_axis',(-0.734815376098624,-0.678267176744561,0.));
#23847=DIRECTION('center_axis',(-0.954804293663248,0.297235194420558,-1.28532498698092E-14));
#23848=DIRECTION('ref_axis',(0.297235194420558,0.954804293663248,-1.26871517833745E-11));
#23849=DIRECTION('center_axis',(-0.975502371165106,-0.219988917564627,0.));
#23850=DIRECTION('ref_axis',(-0.219988917564627,0.975502371165106,0.));
#23851=DIRECTION('center_axis',(-0.954804293663331,0.297235194420291,2.31967918986522E-13));
#23852=DIRECTION('ref_axis',(0.297235194420291,0.954804293663331,5.5906824425949E-12));
#23853=DIRECTION('center_axis',(0.975502371165106,0.219988917564627,0.));
#23854=DIRECTION('ref_axis',(0.219988917564627,-0.975502371165106,0.));
#23855=DIRECTION('center_axis',(-0.734815376098563,-0.678267176744628,-1.56233468245057E-14));
#23856=DIRECTION('ref_axis',(0.678267176744628,-0.734815376098563,2.56800988528237E-12));
#23857=DIRECTION('center_axis',(-0.678267176744561,0.734815376098624,0.));
#23858=DIRECTION('ref_axis',(0.734815376098624,0.678267176744561,0.));
#23859=DIRECTION('center_axis',(-0.219988917564712,0.975502371165087,1.20748526255343E-13));
#23860=DIRECTION('ref_axis',(0.975502371165087,0.219988917564712,-8.28276908751904E-12));
#23861=DIRECTION('center_axis',(0.297235194420542,0.954804293663253,0.));
#23862=DIRECTION('ref_axis',(0.954804293663252,-0.297235194420542,0.));
#23863=DIRECTION('center_axis',(0.,0.,1.));
#23864=DIRECTION('ref_axis',(0.990993942369174,-0.133906707029938,0.));
#23865=DIRECTION('',(0.,0.,1.));
#23866=DIRECTION('center_axis',(0.,0.,1.));
#23867=DIRECTION('ref_axis',(1.,0.,0.));
#23868=DIRECTION('center_axis',(0.,0.,1.));
#23869=DIRECTION('ref_axis',(1.,0.,0.));
#23870=DIRECTION('center_axis',(0.,0.,-1.));
#23871=DIRECTION('ref_axis',(-0.999820197862873,0.0189623823779183,0.));
#23872=DIRECTION('',(0.,0.,-1.));
#23873=DIRECTION('center_axis',(0.,0.,1.));
#23874=DIRECTION('ref_axis',(0.999820197862873,-0.0189623823779183,0.));
#23875=DIRECTION('center_axis',(0.39446700523415,0.918910105386594,0.));
#23876=DIRECTION('ref_axis',(0.,0.,-1.));
#23877=DIRECTION('',(0.918910105386594,-0.39446700523415,0.));
#23878=DIRECTION('',(0.,0.,-1.));
#23879=DIRECTION('',(0.918910105386594,-0.39446700523415,0.));
#23880=DIRECTION('',(0.,0.,-1.));
#23881=DIRECTION('center_axis',(0.,0.,-1.));
#23882=DIRECTION('ref_axis',(-0.999820197862872,0.0189623823779211,0.));
#23883=DIRECTION('center_axis',(0.,0.,1.));
#23884=DIRECTION('ref_axis',(0.999820197862872,-0.0189623823779211,0.));
#23885=DIRECTION('',(0.,0.,-1.));
#23886=DIRECTION('center_axis',(0.,0.,1.));
#23887=DIRECTION('ref_axis',(0.999820197862872,-0.0189623823779211,0.));
#23888=DIRECTION('center_axis',(-0.399400362728205,-0.91677660869624,0.));
#23889=DIRECTION('ref_axis',(-0.91677660869624,0.399400362728205,0.));
#23890=DIRECTION('',(-0.91677660869624,0.399400362728205,0.));
#23891=DIRECTION('',(-0.91677660869624,0.399400362728205,0.));
#23892=DIRECTION('',(0.,0.,-1.));
#23893=DIRECTION('center_axis',(-0.844295148658605,-0.535878439528541,0.));
#23894=DIRECTION('ref_axis',(-0.535878439528541,0.844295148658605,0.));
#23895=DIRECTION('',(-0.535878439528541,0.844295148658605,0.));
#23896=DIRECTION('',(-0.535878439528541,0.844295148658605,0.));
#23897=DIRECTION('',(0.,0.,-1.));
#23898=DIRECTION('center_axis',(0.213055394807629,-0.977040121358056,0.));
#23899=DIRECTION('ref_axis',(0.,0.,-1.));
#23900=DIRECTION('',(-0.977040121358056,-0.213055394807629,0.));
#23901=DIRECTION('',(-0.977040121358056,-0.213055394807629,0.));
#23902=DIRECTION('',(0.,0.,-1.));
#23903=DIRECTION('center_axis',(-0.91677660869624,0.399400362728203,0.));
#23904=DIRECTION('ref_axis',(0.,0.,1.));
#23905=DIRECTION('',(0.399400362728203,0.91677660869624,0.));
#23906=DIRECTION('',(0.399400362728203,0.91677660869624,0.));
#23907=DIRECTION('',(0.,0.,-1.));
#23908=DIRECTION('center_axis',(-0.38850791323187,-0.921445387071973,0.));
#23909=DIRECTION('ref_axis',(-0.921445387071973,0.38850791323187,0.));
#23910=DIRECTION('',(-0.921445387071973,0.38850791323187,0.));
#23911=DIRECTION('',(-0.921445387071973,0.38850791323187,0.));
#23912=DIRECTION('',(0.,0.,-1.));
#23913=DIRECTION('center_axis',(0.213055394807629,-0.977040121358056,0.));
#23914=DIRECTION('ref_axis',(0.,0.,-1.));
#23915=DIRECTION('',(-0.977040121358056,-0.213055394807629,0.));
#23916=DIRECTION('',(-0.977040121358056,-0.213055394807629,0.));
#23917=DIRECTION('',(0.,0.,-1.));
#23918=DIRECTION('center_axis',(-0.91677660869624,0.399400362728203,0.));
#23919=DIRECTION('ref_axis',(0.,0.,1.));
#23920=DIRECTION('',(0.399400362728203,0.91677660869624,0.));
#23921=DIRECTION('',(0.399400362728203,0.91677660869624,0.));
#23922=DIRECTION('',(0.,0.,-1.));
#23923=DIRECTION('center_axis',(-0.388507913231866,-0.921445387071974,0.));
#23924=DIRECTION('ref_axis',(-0.921445387071975,0.388507913231866,0.));
#23925=DIRECTION('',(-0.921445387071974,0.388507913231866,0.));
#23926=DIRECTION('',(-0.921445387071974,0.388507913231866,0.));
#23927=DIRECTION('',(0.,0.,-1.));
#23928=DIRECTION('center_axis',(0.213055394807629,-0.977040121358056,0.));
#23929=DIRECTION('ref_axis',(0.,0.,-1.));
#23930=DIRECTION('',(-0.977040121358056,-0.213055394807629,0.));
#23931=DIRECTION('',(-0.977040121358056,-0.213055394807629,0.));
#23932=DIRECTION('',(0.,0.,-1.));
#23933=DIRECTION('center_axis',(-0.91677660869624,0.399400362728203,0.));
#23934=DIRECTION('ref_axis',(0.,0.,1.));
#23935=DIRECTION('',(0.399400362728203,0.91677660869624,0.));
#23936=DIRECTION('',(0.399400362728203,0.91677660869624,0.));
#23937=DIRECTION('',(0.,0.,-1.));
#23938=DIRECTION('center_axis',(-0.38850791323187,-0.921445387071973,0.));
#23939=DIRECTION('ref_axis',(-0.921445387071973,0.38850791323187,0.));
#23940=DIRECTION('',(-0.921445387071973,0.38850791323187,0.));
#23941=DIRECTION('',(-0.921445387071973,0.38850791323187,0.));
#23942=DIRECTION('',(0.,0.,-1.));
#23943=DIRECTION('center_axis',(0.213055394807629,-0.977040121358056,0.));
#23944=DIRECTION('ref_axis',(0.,0.,-1.));
#23945=DIRECTION('',(-0.977040121358056,-0.213055394807629,0.));
#23946=DIRECTION('',(-0.977040121358056,-0.213055394807629,0.));
#23947=DIRECTION('',(0.,0.,-1.));
#23948=DIRECTION('center_axis',(-0.91677660869624,0.399400362728203,0.));
#23949=DIRECTION('ref_axis',(0.,0.,1.));
#23950=DIRECTION('',(0.399400362728203,0.91677660869624,0.));
#23951=DIRECTION('',(0.399400362728203,0.91677660869624,0.));
#23952=DIRECTION('',(0.,0.,-1.));
#23953=DIRECTION('center_axis',(-0.38850791323187,-0.921445387071973,0.));
#23954=DIRECTION('ref_axis',(-0.921445387071973,0.38850791323187,0.));
#23955=DIRECTION('',(-0.921445387071973,0.38850791323187,0.));
#23956=DIRECTION('',(-0.921445387071973,0.38850791323187,0.));
#23957=DIRECTION('',(0.,0.,-1.));
#23958=DIRECTION('center_axis',(0.213055394807629,-0.977040121358056,0.));
#23959=DIRECTION('ref_axis',(0.,0.,-1.));
#23960=DIRECTION('',(-0.977040121358056,-0.213055394807629,0.));
#23961=DIRECTION('',(-0.977040121358056,-0.213055394807629,0.));
#23962=DIRECTION('',(0.,0.,-1.));
#23963=DIRECTION('center_axis',(-0.916776608696241,0.399400362728203,0.));
#23964=DIRECTION('ref_axis',(0.,0.,1.));
#23965=DIRECTION('',(0.399400362728203,0.916776608696241,0.));
#23966=DIRECTION('',(0.399400362728203,0.916776608696241,0.));
#23967=DIRECTION('',(0.,0.,-1.));
#23968=DIRECTION('center_axis',(-0.388507913231868,-0.921445387071974,0.));
#23969=DIRECTION('ref_axis',(-0.921445387071974,0.388507913231868,0.));
#23970=DIRECTION('',(-0.921445387071974,0.388507913231868,0.));
#23971=DIRECTION('',(-0.921445387071974,0.388507913231868,0.));
#23972=DIRECTION('',(0.,0.,-1.));
#23973=DIRECTION('center_axis',(0.213055394807629,-0.977040121358056,0.));
#23974=DIRECTION('ref_axis',(0.,0.,-1.));
#23975=DIRECTION('',(-0.977040121358056,-0.213055394807629,0.));
#23976=DIRECTION('',(-0.977040121358056,-0.213055394807629,0.));
#23977=DIRECTION('',(0.,0.,-1.));
#23978=DIRECTION('center_axis',(-0.91677660869624,0.399400362728203,0.));
#23979=DIRECTION('ref_axis',(0.,0.,1.));
#23980=DIRECTION('',(0.399400362728203,0.91677660869624,0.));
#23981=DIRECTION('',(0.399400362728203,0.91677660869624,0.));
#23982=DIRECTION('',(0.,0.,-1.));
#23983=DIRECTION('center_axis',(-0.38850791323187,-0.921445387071973,0.));
#23984=DIRECTION('ref_axis',(-0.921445387071973,0.38850791323187,0.));
#23985=DIRECTION('',(-0.921445387071973,0.38850791323187,0.));
#23986=DIRECTION('',(-0.921445387071973,0.38850791323187,0.));
#23987=DIRECTION('',(0.,0.,-1.));
#23988=DIRECTION('center_axis',(0.213055394807629,-0.977040121358056,0.));
#23989=DIRECTION('ref_axis',(0.,0.,-1.));
#23990=DIRECTION('',(-0.977040121358056,-0.213055394807629,0.));
#23991=DIRECTION('',(-0.977040121358056,-0.213055394807629,0.));
#23992=DIRECTION('',(0.,0.,-1.));
#23993=DIRECTION('center_axis',(-0.916776608696241,0.399400362728203,0.));
#23994=DIRECTION('ref_axis',(0.,0.,1.));
#23995=DIRECTION('',(0.399400362728203,0.916776608696241,0.));
#23996=DIRECTION('',(0.399400362728203,0.916776608696241,0.));
#23997=DIRECTION('',(0.,0.,-1.));
#23998=DIRECTION('center_axis',(-0.388507913231866,-0.921445387071974,0.));
#23999=DIRECTION('ref_axis',(-0.921445387071975,0.388507913231866,0.));
#24000=DIRECTION('',(-0.921445387071974,0.388507913231866,0.));
#24001=DIRECTION('',(-0.921445387071974,0.388507913231866,0.));
#24002=DIRECTION('',(0.,0.,-1.));
#24003=DIRECTION('center_axis',(0.21305539480763,-0.977040121358056,0.));
#24004=DIRECTION('ref_axis',(0.,0.,-1.));
#24005=DIRECTION('',(-0.977040121358056,-0.21305539480763,0.));
#24006=DIRECTION('',(-0.977040121358056,-0.21305539480763,0.));
#24007=DIRECTION('',(0.,0.,-1.));
#24008=DIRECTION('center_axis',(-0.916776608696241,0.399400362728203,0.));
#24009=DIRECTION('ref_axis',(0.,0.,1.));
#24010=DIRECTION('',(0.399400362728203,0.916776608696241,0.));
#24011=DIRECTION('',(0.399400362728203,0.916776608696241,0.));
#24012=DIRECTION('',(0.,0.,-1.));
#24013=DIRECTION('center_axis',(-0.388507913231866,-0.921445387071974,0.));
#24014=DIRECTION('ref_axis',(-0.921445387071975,0.388507913231866,0.));
#24015=DIRECTION('',(-0.921445387071974,0.388507913231866,0.));
#24016=DIRECTION('',(-0.921445387071974,0.388507913231866,0.));
#24017=DIRECTION('',(0.,0.,-1.));
#24018=DIRECTION('center_axis',(0.21305539480763,-0.977040121358056,0.));
#24019=DIRECTION('ref_axis',(0.,0.,-1.));
#24020=DIRECTION('',(-0.977040121358056,-0.21305539480763,0.));
#24021=DIRECTION('',(-0.977040121358056,-0.21305539480763,0.));
#24022=DIRECTION('',(0.,0.,-1.));
#24023=DIRECTION('center_axis',(-0.91677660869624,0.399400362728203,0.));
#24024=DIRECTION('ref_axis',(0.,0.,1.));
#24025=DIRECTION('',(0.399400362728203,0.91677660869624,0.));
#24026=DIRECTION('',(0.399400362728203,0.91677660869624,0.));
#24027=DIRECTION('',(0.,0.,-1.));
#24028=DIRECTION('center_axis',(-0.388507913231866,-0.921445387071974,0.));
#24029=DIRECTION('ref_axis',(-0.921445387071975,0.388507913231866,0.));
#24030=DIRECTION('',(-0.921445387071974,0.388507913231866,0.));
#24031=DIRECTION('',(-0.921445387071974,0.388507913231866,0.));
#24032=DIRECTION('',(0.,0.,-1.));
#24033=DIRECTION('center_axis',(0.213055394807629,-0.977040121358056,0.));
#24034=DIRECTION('ref_axis',(0.,0.,-1.));
#24035=DIRECTION('',(-0.977040121358056,-0.213055394807629,0.));
#24036=DIRECTION('',(-0.977040121358056,-0.213055394807629,0.));
#24037=DIRECTION('',(0.,0.,-1.));
#24038=DIRECTION('center_axis',(-0.91677660869624,0.399400362728203,0.));
#24039=DIRECTION('ref_axis',(0.,0.,1.));
#24040=DIRECTION('',(0.399400362728203,0.91677660869624,0.));
#24041=DIRECTION('',(0.399400362728203,0.91677660869624,0.));
#24042=DIRECTION('',(0.,0.,-1.));
#24043=DIRECTION('center_axis',(-0.388507913231873,-0.921445387071972,0.));
#24044=DIRECTION('ref_axis',(-0.921445387071971,0.388507913231873,0.));
#24045=DIRECTION('',(-0.921445387071971,0.388507913231873,0.));
#24046=DIRECTION('',(-0.921445387071971,0.388507913231873,0.));
#24047=DIRECTION('',(0.,0.,-1.));
#24048=DIRECTION('center_axis',(0.213055394807629,-0.977040121358056,0.));
#24049=DIRECTION('ref_axis',(0.,0.,-1.));
#24050=DIRECTION('',(-0.977040121358056,-0.213055394807629,0.));
#24051=DIRECTION('',(-0.977040121358056,-0.213055394807629,0.));
#24052=DIRECTION('',(0.,0.,-1.));
#24053=DIRECTION('center_axis',(-0.916776608696241,0.399400362728203,0.));
#24054=DIRECTION('ref_axis',(0.,0.,1.));
#24055=DIRECTION('',(0.399400362728203,0.916776608696241,0.));
#24056=DIRECTION('',(0.399400362728203,0.916776608696241,0.));
#24057=DIRECTION('',(0.,0.,-1.));
#24058=DIRECTION('center_axis',(-0.388507913231871,-0.921445387071973,0.));
#24059=DIRECTION('ref_axis',(-0.921445387071973,0.388507913231871,0.));
#24060=DIRECTION('',(-0.921445387071973,0.388507913231871,0.));
#24061=DIRECTION('',(-0.921445387071973,0.388507913231871,0.));
#24062=DIRECTION('',(0.,0.,-1.));
#24063=DIRECTION('center_axis',(0.213055394807631,-0.977040121358056,0.));
#24064=DIRECTION('ref_axis',(0.,0.,-1.));
#24065=DIRECTION('',(-0.977040121358056,-0.213055394807631,0.));
#24066=DIRECTION('',(-0.977040121358056,-0.213055394807631,0.));
#24067=DIRECTION('',(0.,0.,-1.));
#24068=DIRECTION('center_axis',(-0.916776608696241,0.399400362728203,0.));
#24069=DIRECTION('ref_axis',(0.,0.,1.));
#24070=DIRECTION('',(0.399400362728203,0.916776608696241,0.));
#24071=DIRECTION('',(0.399400362728203,0.916776608696241,0.));
#24072=DIRECTION('',(0.,0.,-1.));
#24073=DIRECTION('center_axis',(-0.436416285895279,-0.899744866840245,0.));
#24074=DIRECTION('ref_axis',(-0.899744866840245,0.436416285895279,0.));
#24075=DIRECTION('',(-0.899744866840245,0.436416285895278,0.));
#24076=DIRECTION('',(-0.899744866840245,0.436416285895278,0.));
#24077=DIRECTION('',(0.,0.,-1.));
#24078=DIRECTION('center_axis',(0.,0.,-1.));
#24079=DIRECTION('ref_axis',(-0.999820197862872,0.0189623823779216,0.));
#24080=DIRECTION('center_axis',(0.,0.,1.));
#24081=DIRECTION('ref_axis',(-0.999820197862872,0.0189623823779216,0.));
#24082=DIRECTION('center_axis',(0.,0.,1.));
#24083=DIRECTION('ref_axis',(-0.999820197862872,0.0189623823779216,0.));
#24084=DIRECTION('',(0.,0.,-1.));
#24085=DIRECTION('center_axis',(0.399400362728205,0.91677660869624,0.));
#24086=DIRECTION('ref_axis',(0.,0.,-1.));
#24087=DIRECTION('',(0.91677660869624,-0.399400362728205,0.));
#24088=DIRECTION('',(0.91677660869624,-0.399400362728205,0.));
#24089=DIRECTION('',(0.,0.,-1.));
#24090=DIRECTION('center_axis',(0.740794344427866,0.671731895374701,0.));
#24091=DIRECTION('ref_axis',(0.,0.,-1.));
#24092=DIRECTION('',(0.671731895374701,-0.740794344427866,0.));
#24093=DIRECTION('',(0.671731895374701,-0.740794344427866,0.));
#24094=DIRECTION('center_axis',(0.,0.,1.));
#24095=DIRECTION('ref_axis',(0.999820197862872,-0.018962382377922,0.));
#24096=DIRECTION('center_axis',(0.,0.,1.));
#24097=DIRECTION('ref_axis',(0.999820197862872,-0.018962382377922,0.));
#24098=DIRECTION('center_axis',(0.,0.,1.));
#24099=DIRECTION('ref_axis',(1.,0.,0.));
#33752=CARTESIAN_POINT('',(0.,0.,0.));
#33753=CARTESIAN_POINT('Origin',(25.187903481163,63.761980950099,202.2));
#33754=CARTESIAN_POINT('',(21.2239277116833,64.2976077782208,202.2));
#33755=CARTESIAN_POINT('Origin',(25.18790348116,63.761980950101,202.2));
#33756=CARTESIAN_POINT('',(21.587903481163,63.761980950099,202.2));
#33757=CARTESIAN_POINT('Origin',(25.187903481163,63.761980950099,202.2));
#33758=CARTESIAN_POINT('Origin',(25.187903481163,63.761980950099,202.6));
#33759=CARTESIAN_POINT('',(21.2239277116865,64.2976077782203,202.6));
#33760=CARTESIAN_POINT('',(21.187903481163,63.761980950099,202.6));
#33761=CARTESIAN_POINT('Origin',(25.187903481163,63.761980950099,202.6));
#33762=CARTESIAN_POINT('Origin',(25.187903481163,63.761980950099,202.6));
#33763=CARTESIAN_POINT('',(21.187903481163,63.761980950099,202.6));
#33764=CARTESIAN_POINT('Origin',(25.18790348116,63.761980950101,211.3));
#33765=CARTESIAN_POINT('',(21.2239277116833,64.2976077782208,211.3));
#33766=CARTESIAN_POINT('Origin',(25.187903481163,63.761980950099,212.5));
#33767=CARTESIAN_POINT('',(26.787903481163,63.7619809500987,203.));
#33768=CARTESIAN_POINT('',(26.787903481163,63.761980950099,202.912499998088));
#33769=CARTESIAN_POINT('',(26.787903481163,63.761980950099,212.5));
#33770=CARTESIAN_POINT('',(26.787903481163,63.761980950099,202.6));
#33771=CARTESIAN_POINT('',(26.787903481163,63.761980950099,202.606249999044));
#33772=CARTESIAN_POINT('',(23.7486592957405,64.4609631921677,202.6));
#33773=CARTESIAN_POINT('Origin',(25.187903481163,63.761980950099,202.6));
#33774=CARTESIAN_POINT('Ctrl Pts',(26.787903481163,63.7619809500983,203.));
#33775=CARTESIAN_POINT('Ctrl Pts',(26.787903481163,63.7112520004935,202.996796584235));
#33776=CARTESIAN_POINT('Ctrl Pts',(26.7854910924781,63.6604721236311,202.99350200086));
#33777=CARTESIAN_POINT('Ctrl Pts',(26.7604511514014,63.3983856951183,202.97603893493));
#33778=CARTESIAN_POINT('Ctrl Pts',(26.6983614293065,63.1931353440354,202.960814162487));
#33779=CARTESIAN_POINT('Ctrl Pts',(26.5003141481196,62.8236961479851,202.930264458459));
#33780=CARTESIAN_POINT('Ctrl Pts',(26.3681111928548,62.662010067521,202.915234457258));
#33781=CARTESIAN_POINT('Ctrl Pts',(26.0503971457733,62.3987480817403,202.887026747492));
#33782=CARTESIAN_POINT('Ctrl Pts',(25.8682694857742,62.2993104687815,202.874610021169));
#33783=CARTESIAN_POINT('Ctrl Pts',(25.4696943299171,62.1727174517791,202.845547249388));
#33784=CARTESIAN_POINT('Ctrl Pts',(25.2563670240156,62.1493873298679,202.829992133333));
#33785=CARTESIAN_POINT('Ctrl Pts',(24.8410914178345,62.1866934369787,202.799711620382));
#33786=CARTESIAN_POINT('Ctrl Pts',(24.6427688077468,62.2438637796842,202.78525059673));
#33787=CARTESIAN_POINT('Ctrl Pts',(24.2712058497153,62.4335018359131,202.758157464374));
#33788=CARTESIAN_POINT('Ctrl Pts',(24.1029599888896,62.5669294408852,202.744242838934));
#33789=CARTESIAN_POINT('Ctrl Pts',(23.8302633753762,62.8897168830665,202.713917494956));
#33790=CARTESIAN_POINT('Ctrl Pts',(23.7276898417191,63.0750963218571,202.69847155234));
#33791=CARTESIAN_POINT('Ctrl Pts',(23.6024417596993,63.4670668651279,202.669153183349));
#33792=CARTESIAN_POINT('Ctrl Pts',(23.5779451866174,63.668940007034,202.656238383051));
#33793=CARTESIAN_POINT('Ctrl Pts',(23.6054510774695,64.0753209334884,202.629573549099));
#33794=CARTESIAN_POINT('Ctrl Pts',(23.6588128449442,64.2759642406826,202.614957907494));
#33795=CARTESIAN_POINT('Ctrl Pts',(23.7486592957404,64.4609631921677,202.6));
#33796=CARTESIAN_POINT('Origin',(25.187903481163,63.761980950099,212.5));
#33797=CARTESIAN_POINT('',(26.787903481163,63.7619809500989,203.7));
#33798=CARTESIAN_POINT('',(26.787903481163,63.761980950099,203.612499998088));
#33799=CARTESIAN_POINT('',(26.787903481163,63.761980950099,212.5));
#33800=CARTESIAN_POINT('Ctrl Pts',(26.787903481163,63.761980950099,202.912499998088));
#33801=CARTESIAN_POINT('Ctrl Pts',(26.787903481163,63.8816035254339,202.920053886877));
#33802=CARTESIAN_POINT('Ctrl Pts',(26.7744883750838,64.0008235214565,202.928071446123));
#33803=CARTESIAN_POINT('Ctrl Pts',(26.7204285286892,64.2381005673036,202.945025874336));
#33804=CARTESIAN_POINT('Ctrl Pts',(26.6790200147457,64.3551822716112,202.953928998405));
#33805=CARTESIAN_POINT('Ctrl Pts',(26.5308024775844,64.6575072281504,202.978423884113));
#33806=CARTESIAN_POINT('Ctrl Pts',(26.3998178470323,64.8281102460966,202.99397255119));
#33807=CARTESIAN_POINT('Ctrl Pts',(26.0848356880736,65.1026820164517,203.02279484759));
#33808=CARTESIAN_POINT('Ctrl Pts',(25.9060478414617,65.2063614843149,203.03513530515));
#33809=CARTESIAN_POINT('Ctrl Pts',(25.5166022913437,65.3415259652012,203.063532376512));
#33810=CARTESIAN_POINT('Ctrl Pts',(25.3093537590403,65.3707793765029,203.07864424866));
#33811=CARTESIAN_POINT('Ctrl Pts',(24.8903683797337,65.3483380052435,203.109195265901));
#33812=CARTESIAN_POINT('Ctrl Pts',(24.682721061272,65.2949157615971,203.124336216205));
#33813=CARTESIAN_POINT('Ctrl Pts',(24.3089997865868,65.1142494804449,203.151586725818));
#33814=CARTESIAN_POINT('Ctrl Pts',(24.1448884786953,64.9921268833827,203.164512384635));
#33815=CARTESIAN_POINT('Ctrl Pts',(23.8662397612558,64.687836578348,203.193886681));
#33816=CARTESIAN_POINT('Ctrl Pts',(23.7563717425979,64.5067740759857,203.209325963837));
#33817=CARTESIAN_POINT('Ctrl Pts',(23.6116618059432,64.1095748583762,203.239684058295));
#33818=CARTESIAN_POINT('Ctrl Pts',(23.5794678262025,63.8970057212076,203.253665946361));
#33819=CARTESIAN_POINT('Ctrl Pts',(23.599697430425,63.4801535614309,203.280726733181));
#33820=CARTESIAN_POINT('Ctrl Pts',(23.6486804568962,63.2797206238055,203.295169448835));
#33821=CARTESIAN_POINT('Ctrl Pts',(23.8226994528204,62.9009738311223,203.325430874816));
#33822=CARTESIAN_POINT('Ctrl Pts',(23.9489389782711,62.7275242008688,203.34098630025));
#33823=CARTESIAN_POINT('Ctrl Pts',(24.256932832041,62.4445394311034,203.370085076132));
#33824=CARTESIAN_POINT('Ctrl Pts',(24.4338702113582,62.3358715183235,203.382518405498));
#33825=CARTESIAN_POINT('Ctrl Pts',(24.8203227249822,62.1910946963225,203.410697234617));
#33826=CARTESIAN_POINT('Ctrl Pts',(25.0262711719672,62.1567869763195,203.425714308876));
#33827=CARTESIAN_POINT('Ctrl Pts',(25.4452179976236,62.1686010277284,203.456262514913));
#33828=CARTESIAN_POINT('Ctrl Pts',(25.6541792260724,62.2167638482125,203.471499271154));
#33829=CARTESIAN_POINT('Ctrl Pts',(26.0324903692996,62.3879978620503,203.499084458681));
#33830=CARTESIAN_POINT('Ctrl Pts',(26.1997047745697,62.5060199489405,203.511744223034));
#33831=CARTESIAN_POINT('Ctrl Pts',(26.4855979882815,62.8029319913109,203.540916721447));
#33832=CARTESIAN_POINT('Ctrl Pts',(26.5997607566442,62.980676287076,203.556303046633));
#33833=CARTESIAN_POINT('Ctrl Pts',(26.7501748873287,63.3623426521135,203.585888242806));
#33834=CARTESIAN_POINT('Ctrl Pts',(26.787903481163,63.5613581222044,203.599831130809));
#33835=CARTESIAN_POINT('Ctrl Pts',(26.787903481163,63.761980950099,203.612499998088));
#33836=CARTESIAN_POINT('Ctrl Pts',(26.787903481163,63.7619809500988,203.7));
#33837=CARTESIAN_POINT('Ctrl Pts',(26.787903481163,63.6848495192057,203.695129328645));
#33838=CARTESIAN_POINT('Ctrl Pts',(26.7823272250583,63.6076663989242,203.690052092221));
#33839=CARTESIAN_POINT('Ctrl Pts',(26.7402499780708,63.3192289003551,203.670303865423));
#33840=CARTESIAN_POINT('Ctrl Pts',(26.667176531147,63.11581633677,203.654794696706));
#33841=CARTESIAN_POINT('Ctrl Pts',(26.4496343128889,62.7567934686976,203.624192006769));
#33842=CARTESIAN_POINT('Ctrl Pts',(26.3099733765155,62.602947229556,203.609385167843));
#33843=CARTESIAN_POINT('Ctrl Pts',(25.9781444640218,62.3552648464668,203.581646669462));
#33844=CARTESIAN_POINT('Ctrl Pts',(25.7886683527539,62.2645066921842,203.568805771887));
#33845=CARTESIAN_POINT('Ctrl Pts',(25.382369354266,62.1598394149872,203.539179803247));
#33846=CARTESIAN_POINT('Ctrl Pts',(25.1692663810009,62.1481911110961,203.52364104478));
#33847=CARTESIAN_POINT('Ctrl Pts',(24.7587322026718,62.207248987663,203.493706260943));
#33848=CARTESIAN_POINT('Ctrl Pts',(24.5646851694379,62.2743564463977,203.479556998103));
#33849=CARTESIAN_POINT('Ctrl Pts',(24.2046978751832,62.4820298420444,203.453307924564));
#33850=CARTESIAN_POINT('Ctrl Pts',(24.0437650457417,62.6235440783622,203.438509606632));
#33851=CARTESIAN_POINT('Ctrl Pts',(23.7885670062959,62.9585764544945,203.40804899226));
#33852=CARTESIAN_POINT('Ctrl Pts',(23.6957639269873,63.1478699907815,203.392712097927));
#33853=CARTESIAN_POINT('Ctrl Pts',(23.5895951555988,63.5459326838728,203.36370462364));
#33854=CARTESIAN_POINT('Ctrl Pts',(23.5751062397505,63.7503103057142,203.351203540277));
#33855=CARTESIAN_POINT('Ctrl Pts',(23.6247059389547,64.1650452428808,203.323205666452));
#33856=CARTESIAN_POINT('Ctrl Pts',(23.6927866095703,64.3707804740557,203.307731854955));
#33857=CARTESIAN_POINT('Ctrl Pts',(23.9018731775003,64.7359913494376,203.277046685596));
#33858=CARTESIAN_POINT('Ctrl Pts',(24.0380772095468,64.8935726524055,203.262130019003));
#33859=CARTESIAN_POINT('Ctrl Pts',(24.3632744096962,65.1486279853084,203.234167717085));
#33860=CARTESIAN_POINT('Ctrl Pts',(24.5492366279778,65.2435061649562,203.221569458045));
#33861=CARTESIAN_POINT('Ctrl Pts',(24.9519305603642,65.3586094432589,203.192206358808));
#33862=CARTESIAN_POINT('Ctrl Pts',(25.1652176392351,65.3757892043211,203.176654175974));
#33863=CARTESIAN_POINT('Ctrl Pts',(25.5781415174269,65.3270040389637,203.146545143189));
#33864=CARTESIAN_POINT('Ctrl Pts',(25.7742792068995,65.2645760304671,203.132243436665));
#33865=CARTESIAN_POINT('Ctrl Pts',(26.1397504343722,65.0654395529092,203.105594492995));
#33866=CARTESIAN_POINT('Ctrl Pts',(26.3041087678418,64.9278245374005,203.091258673341));
#33867=CARTESIAN_POINT('Ctrl Pts',(26.567675494015,64.598662470267,203.060863647025));
#33868=CARTESIAN_POINT('Ctrl Pts',(26.665181531593,64.4111833670911,203.045469867924));
#33869=CARTESIAN_POINT('Ctrl Pts',(26.7664096376625,64.0643397927398,203.019876890872));
#33870=CARTESIAN_POINT('Ctrl Pts',(26.7879034811631,63.913436868219,203.009564090714));
#33871=CARTESIAN_POINT('Ctrl Pts',(26.787903481163,63.7619809500983,203.));
#33872=CARTESIAN_POINT('Origin',(25.187903481163,63.761980950099,212.5));
#33873=CARTESIAN_POINT('',(26.787903481163,63.761980950099,204.4));
#33874=CARTESIAN_POINT('',(26.787903481163,63.761980950099,204.312499998088));
#33875=CARTESIAN_POINT('',(26.787903481163,63.761980950099,212.5));
#33876=CARTESIAN_POINT('Ctrl Pts',(26.787903481163,63.761980950099,203.612499998088));
#33877=CARTESIAN_POINT('Ctrl Pts',(26.787903481163,63.7733300716832,203.613216668851));
#33878=CARTESIAN_POINT('Ctrl Pts',(26.7877827289335,63.7846837908196,203.613938032363));
#33879=CARTESIAN_POINT('Ctrl Pts',(26.7831991936214,63.9999555727865,203.627699055248));
#33880=CARTESIAN_POINT('Ctrl Pts',(26.7399082191147,64.2011116260035,203.64197991125));
#33881=CARTESIAN_POINT('Ctrl Pts',(26.5771050844058,64.5835518640169,203.672065658149));
#33882=CARTESIAN_POINT('Ctrl Pts',(26.4562637840854,64.760046779607,203.687616576013));
#33883=CARTESIAN_POINT('Ctrl Pts',(26.1562407270751,65.0524095270444,203.717016947517));
#33884=CARTESIAN_POINT('Ctrl Pts',(25.9813472815784,65.1667299651493,203.729644720974));
#33885=CARTESIAN_POINT('Ctrl Pts',(25.5982921414466,65.3221582302966,203.757575824942));
#33886=CARTESIAN_POINT('Ctrl Pts',(25.3939258076125,65.3620110358385,203.772477536784));
#33887=CARTESIAN_POINT('Ctrl Pts',(24.9732446111159,65.3619496379482,203.803152207362));
#33888=CARTESIAN_POINT('Ctrl Pts',(24.7609557974199,65.3188140611529,203.818631600028));
#33889=CARTESIAN_POINT('Ctrl Pts',(24.3764131853069,65.1558088196326,203.846671165494));
#33890=CARTESIAN_POINT('Ctrl Pts',(24.2062081008249,65.0416531052197,203.859149307122));
#33891=CARTESIAN_POINT('Ctrl Pts',(23.913547622975,64.7517280732952,203.888127315167));
#33892=CARTESIAN_POINT('Ctrl Pts',(23.7954277427113,64.5771996837515,203.903454833022));
#33893=CARTESIAN_POINT('Ctrl Pts',(23.6315585215372,64.1895285406312,203.933909767209));
#33894=CARTESIAN_POINT('Ctrl Pts',(23.5886182636867,63.9795728728208,203.948733511963));
#33895=CARTESIAN_POINT('Ctrl Pts',(23.587236335398,63.5640341496619,203.975024203449));
#33896=CARTESIAN_POINT('Ctrl Pts',(23.625303899541,63.3623430739075,203.989099762005));
#33897=CARTESIAN_POINT('Ctrl Pts',(23.7779729029101,62.9766614093573,204.01902072395));
#33898=CARTESIAN_POINT('Ctrl Pts',(23.893872407819,62.7975518937715,204.034556578128));
#33899=CARTESIAN_POINT('Ctrl Pts',(24.1865671125536,62.4967695520657,204.064221448014));
#33900=CARTESIAN_POINT('Ctrl Pts',(24.3596325075858,62.377284721672,204.077105239598));
#33901=CARTESIAN_POINT('Ctrl Pts',(24.7395813264973,62.2123431202278,204.104809840977));
#33902=CARTESIAN_POINT('Ctrl Pts',(24.9424115787873,62.1675939414645,204.119599546873));
#33903=CARTESIAN_POINT('Ctrl Pts',(25.3619149100335,62.1571561117494,204.150188331443));
#33904=CARTESIAN_POINT('Ctrl Pts',(25.5746728096165,62.1947594878389,204.165701928288));
#33905=CARTESIAN_POINT('Ctrl Pts',(25.9632553978713,62.3476624489653,204.194036075348));
#33906=CARTESIAN_POINT('Ctrl Pts',(26.1367309575285,62.4576799835756,204.206395745681));
#33907=CARTESIAN_POINT('Ctrl Pts',(26.4365577261353,62.7401058325329,204.235161468695));
#33908=CARTESIAN_POINT('Ctrl Pts',(26.558803278173,62.9111085532163,204.250416763838));
#33909=CARTESIAN_POINT('Ctrl Pts',(26.7325552445008,63.2939238566396,204.280925371403));
#33910=CARTESIAN_POINT('Ctrl Pts',(26.7809711604346,63.5027300416431,204.295876162346));
#33911=CARTESIAN_POINT('Ctrl Pts',(26.7876732452454,63.7306306492175,204.310511905124));
#33912=CARTESIAN_POINT('Ctrl Pts',(26.787903481163,63.7463097723831,204.311510399483));
#33913=CARTESIAN_POINT('Ctrl Pts',(26.787903481163,63.761980950099,204.312499998088));
#33914=CARTESIAN_POINT('Ctrl Pts',(26.787903481163,63.761980950099,204.4));
#33915=CARTESIAN_POINT('Ctrl Pts',(26.787903481163,63.6561553187078,204.393317356291));
#33916=CARTESIAN_POINT('Ctrl Pts',(26.7774081135394,63.5503731163489,204.386254811413));
#33917=CARTESIAN_POINT('Ctrl Pts',(26.7143998470148,63.2374536009571,204.364197491824));
#33918=CARTESIAN_POINT('Ctrl Pts',(26.6311516236278,63.0392550331286,204.348646619481));
#33919=CARTESIAN_POINT('Ctrl Pts',(26.3965428914708,62.6937415201734,204.318274797402));
#33920=CARTESIAN_POINT('Ctrl Pts',(26.249996570115,62.547920352436,204.303723693502));
#33921=CARTESIAN_POINT('Ctrl Pts',(25.9044069654626,62.3158467831105,204.276469163685));
#33922=CARTESIAN_POINT('Ctrl Pts',(25.7072891036901,62.2339218190914,204.262871868309));
#33923=CARTESIAN_POINT('Ctrl Pts',(25.2936850910905,62.1517017382011,204.232713242391));
#33924=CARTESIAN_POINT('Ctrl Pts',(25.081437358254,62.1517468396757,204.217236845205));
#33925=CARTESIAN_POINT('Ctrl Pts',(24.6763013596086,62.2324626340137,204.187695678637));
#33926=CARTESIAN_POINT('Ctrl Pts',(24.4867652763709,62.3095640693849,204.174487767628));
#33927=CARTESIAN_POINT('Ctrl Pts',(24.1386002292873,62.5355834334685,204.147521650523));
#33928=CARTESIAN_POINT('Ctrl Pts',(23.9853316554284,62.6854757681625,204.132468379729));
#33929=CARTESIAN_POINT('Ctrl Pts',(23.7487956744408,63.0325102641257,204.101930246813));
#33930=CARTESIAN_POINT('Ctrl Pts',(23.6663233411312,63.2253504812696,204.086746029573));
#33931=CARTESIAN_POINT('Ctrl Pts',(23.5804723637616,63.6283119424464,204.058169962327));
#33932=CARTESIAN_POINT('Ctrl Pts',(23.5765460629297,63.8342757255467,204.045848824783));
#33933=CARTESIAN_POINT('Ctrl Pts',(23.6479380218796,64.2457884260673,204.017259918275));
#33934=CARTESIAN_POINT('Ctrl Pts',(23.7261388223897,64.446656433769,204.001724497607));
#33935=CARTESIAN_POINT('Ctrl Pts',(23.9523099047955,64.7990266290427,203.971227314556));
#33936=CARTESIAN_POINT('Ctrl Pts',(24.0954681173645,64.9489001045456,203.956543841598));
#33937=CARTESIAN_POINT('Ctrl Pts',(24.4341862593746,65.188821316822,203.929044273366));
#33938=CARTESIAN_POINT('Ctrl Pts',(24.6274289558628,65.2752091081056,203.915867934136));
#33939=CARTESIAN_POINT('Ctrl Pts',(25.0374183239758,65.3687748161157,203.885972876045));
#33940=CARTESIAN_POINT('Ctrl Pts',(25.2501752060529,65.3746029806471,203.870459353393));
#33941=CARTESIAN_POINT('Ctrl Pts',(25.6581670236846,65.3047454842163,203.840709950024));
#33942=CARTESIAN_POINT('Ctrl Pts',(25.8499410107935,65.23265975469,203.827066511306));
#33943=CARTESIAN_POINT('Ctrl Pts',(26.2041413290638,65.0159083960482,203.800465611367));
#33944=CARTESIAN_POINT('Ctrl Pts',(26.3613218928151,64.8701835151,203.785532881));
#33945=CARTESIAN_POINT('Ctrl Pts',(26.6073305316025,64.5291897122417,203.755030846558));
#33946=CARTESIAN_POINT('Ctrl Pts',(26.6950561777834,64.3380787477797,203.739764300592));
#33947=CARTESIAN_POINT('Ctrl Pts',(26.773130908755,64.0128926025622,203.716383073535));
#33948=CARTESIAN_POINT('Ctrl Pts',(26.787903481163,63.8875395652734,203.707928735967));
#33949=CARTESIAN_POINT('Ctrl Pts',(26.787903481163,63.7619809500988,203.7));
#33950=CARTESIAN_POINT('Origin',(25.187903481163,63.761980950099,212.5));
#33951=CARTESIAN_POINT('',(26.787903481163,63.7619809500992,205.1));
#33952=CARTESIAN_POINT('',(26.787903481163,63.7619809500987,205.012499998088));
#33953=CARTESIAN_POINT('',(26.787903481163,63.761980950099,212.5));
#33954=CARTESIAN_POINT('Ctrl Pts',(26.787903481163,63.761980950099,204.312499998088));
#33955=CARTESIAN_POINT('Ctrl Pts',(26.787903481163,63.948993614655,204.32430941505));
#33956=CARTESIAN_POINT('Ctrl Pts',(26.755123306838,64.1347265371673,204.337233129786));
#33957=CARTESIAN_POINT('Ctrl Pts',(26.6185841151114,64.5086708134247,204.365824836775));
#33958=CARTESIAN_POINT('Ctrl Pts',(26.5079299539111,64.6903811727074,204.381333691723));
#33959=CARTESIAN_POINT('Ctrl Pts',(26.2230593960778,64.9999409107975,204.411267578522));
#33960=CARTESIAN_POINT('Ctrl Pts',(26.051903443519,65.124906678974,204.424500000833));
#33961=CARTESIAN_POINT('Ctrl Pts',(25.6752516759775,65.2997239560201,204.451964192216));
#33962=CARTESIAN_POINT('Ctrl Pts',(25.4741356316636,65.3494933455992,204.466628903781));
#33963=CARTESIAN_POINT('Ctrl Pts',(25.0561225496804,65.370749192906,204.497109024342));
#33964=CARTESIAN_POINT('Ctrl Pts',(24.8430251954706,65.3388723881688,204.512647373086));
#33965=CARTESIAN_POINT('Ctrl Pts',(24.4503611404348,65.1964758426224,204.5412791271));
#33966=CARTESIAN_POINT('Ctrl Pts',(24.2734513304366,65.0907111272842,204.553599830484));
#33967=CARTESIAN_POINT('Ctrl Pts',(23.9663523765791,64.8160016283683,204.582143415605));
#33968=CARTESIAN_POINT('Ctrl Pts',(23.8399956290488,64.6487001291288,204.597314874515));
#33969=CARTESIAN_POINT('Ctrl Pts',(23.6562920781972,64.2711090884843,204.627856400161));
#33970=CARTESIAN_POINT('Ctrl Pts',(23.602312744704,64.0636300296916,204.642926219087));
#33971=CARTESIAN_POINT('Ctrl Pts',(23.5790579779837,63.6491950704841,204.669944657668));
#33972=CARTESIAN_POINT('Ctrl Pts',(23.6062675524499,63.4464140350528,204.683096841887));
#33973=CARTESIAN_POINT('Ctrl Pts',(23.7373782505986,63.0547812867918,204.712607621118));
#33974=CARTESIAN_POINT('Ctrl Pts',(23.8426913754904,62.8706008495669,204.72807773049));
#33975=CARTESIAN_POINT('Ctrl Pts',(24.1195338803517,62.5522599158531,204.758273440038));
#33976=CARTESIAN_POINT('Ctrl Pts',(24.2887643768129,62.421704976831,204.771937771729));
#33977=CARTESIAN_POINT('Ctrl Pts',(24.6620546848367,62.2370421258754,204.799156856689));
#33978=CARTESIAN_POINT('Ctrl Pts',(24.8613439415423,62.1823374382017,204.813688364991));
#33979=CARTESIAN_POINT('Ctrl Pts',(25.2776046399742,62.1503923374427,204.844040707585));
#33980=CARTESIAN_POINT('Ctrl Pts',(25.4908919037134,62.1765839518245,204.859592903899));
#33981=CARTESIAN_POINT('Ctrl Pts',(25.8875113204723,62.3084868737419,204.888513069704));
#33982=CARTESIAN_POINT('Ctrl Pts',(26.0678799273478,62.4100430795969,204.900877391633));
#33983=CARTESIAN_POINT('Ctrl Pts',(26.3820689377125,62.677130053086,204.929198123557));
#33984=CARTESIAN_POINT('Ctrl Pts',(26.5123522718067,62.840707990013,204.944277604926));
#33985=CARTESIAN_POINT('Ctrl Pts',(26.7056636418925,63.2129224443078,204.974829896664));
#33986=CARTESIAN_POINT('Ctrl Pts',(26.7650632553928,63.4189512320688,204.990005748706));
#33987=CARTESIAN_POINT('Ctrl Pts',(26.786106360167,63.6743697842249,205.006902035686));
#33988=CARTESIAN_POINT('Ctrl Pts',(26.787903481163,63.7181969529131,205.009735139996));
#33989=CARTESIAN_POINT('Ctrl Pts',(26.787903481163,63.7619809500983,205.012499998088));
#33990=CARTESIAN_POINT('Ctrl Pts',(26.787903481163,63.7619809500994,205.1));
#33991=CARTESIAN_POINT('Ctrl Pts',(26.787903481163,63.6264828425327,205.091443608092));
#33992=CARTESIAN_POINT('Ctrl Pts',(26.7706999926308,63.4912888178938,205.082279207797));
#33993=CARTESIAN_POINT('Ctrl Pts',(26.6832262119226,63.1546623460736,205.057832876903));
#33994=CARTESIAN_POINT('Ctrl Pts',(26.5898345245813,62.962354263357,205.042284161272));
#33995=CARTESIAN_POINT('Ctrl Pts',(26.3384511179543,62.6316035675298,205.012233000256));
#33996=CARTESIAN_POINT('Ctrl Pts',(26.1852709114922,62.494377876291,204.99798282041));
#33997=CARTESIAN_POINT('Ctrl Pts',(25.8284519347283,62.2805296451923,204.971469774332));
#33998=CARTESIAN_POINT('Ctrl Pts',(25.6265091391473,62.2086860884792,204.956981662561));
#33999=CARTESIAN_POINT('Ctrl Pts',(25.2093276052313,62.1485135740385,204.926562175713));
#34000=CARTESIAN_POINT('Ctrl Pts',(24.9984682127779,62.1595268801106,204.91118701168));
#34001=CARTESIAN_POINT('Ctrl Pts',(24.598921244267,62.2605496429551,204.88205337856));
#34002=CARTESIAN_POINT('Ctrl Pts',(24.4134797710973,62.3472573851336,204.869435654593));
#34003=CARTESIAN_POINT('Ctrl Pts',(24.0771653217686,62.5909252241362,204.841787130184));
#34004=CARTESIAN_POINT('Ctrl Pts',(23.9317316240052,62.7485189726601,204.826533179454));
#34005=CARTESIAN_POINT('Ctrl Pts',(23.7138058929658,63.1064132848272,204.795987772974));
#34006=CARTESIAN_POINT('Ctrl Pts',(23.6415075215285,63.3021772569585,204.780989853066));
#34007=CARTESIAN_POINT('Ctrl Pts',(23.5755450635552,63.7096602484942,204.752853363912));
#34008=CARTESIAN_POINT('Ctrl Pts',(23.5821993024926,63.917403894635,204.740393365596));
#34009=CARTESIAN_POINT('Ctrl Pts',(23.6753531498165,64.3252574097626,204.711242125997));
#34010=CARTESIAN_POINT('Ctrl Pts',(23.763368903889,64.5207776850988,204.695686565403));
#34011=CARTESIAN_POINT('Ctrl Pts',(24.0058931859435,64.8595213712486,204.665453654464));
#34012=CARTESIAN_POINT('Ctrl Pts',(24.1555875636601,65.0013801322246,204.651037994492));
#34013=CARTESIAN_POINT('Ctrl Pts',(24.5077604326253,65.2258319272342,204.62402474724));
#34014=CARTESIAN_POINT('Ctrl Pts',(24.7087012206303,65.3033721329043,204.609941831497));
#34015=CARTESIAN_POINT('Ctrl Pts',(25.1256954229462,65.3744585977137,204.579536004245));
#34016=CARTESIAN_POINT('Ctrl Pts',(25.3372953688337,65.3687294288271,204.564106841524));
#34017=CARTESIAN_POINT('Ctrl Pts',(25.7395774805689,65.2774997981902,204.534773770877));
#34018=CARTESIAN_POINT('Ctrl Pts',(25.926979107786,65.1954643550273,204.521909027279));
#34019=CARTESIAN_POINT('Ctrl Pts',(26.2691032021819,64.9603581408769,204.494589339689));
#34020=CARTESIAN_POINT('Ctrl Pts',(26.4184001969773,64.8064601458988,204.479427917871));
#34021=CARTESIAN_POINT('Ctrl Pts',(26.6454454746705,64.4537256532122,204.448875858578));
#34022=CARTESIAN_POINT('Ctrl Pts',(26.7227058672447,64.2593184828226,204.43378271054));
#34023=CARTESIAN_POINT('Ctrl Pts',(26.7788529607801,63.9585157996665,204.412740687797));
#34024=CARTESIAN_POINT('Ctrl Pts',(26.787903481163,63.8602506888824,204.406205506578));
#34025=CARTESIAN_POINT('Ctrl Pts',(26.787903481163,63.761980950099,204.4));
#34026=CARTESIAN_POINT('Origin',(25.187903481163,63.761980950099,212.5));
#34027=CARTESIAN_POINT('',(26.787903481163,63.7619809500994,205.8));
#34028=CARTESIAN_POINT('',(26.787903481163,63.7619809500988,205.712499998088));
#34029=CARTESIAN_POINT('',(26.787903481163,63.761980950099,212.5));
#34030=CARTESIAN_POINT('Ctrl Pts',(26.787903481163,63.7619809500983,205.012499998088));
#34031=CARTESIAN_POINT('Ctrl Pts',(26.7879034811631,63.9203754308701,205.022502242975));
#34032=CARTESIAN_POINT('Ctrl Pts',(26.764394698655,64.078097013435,205.033319086927));
#34033=CARTESIAN_POINT('Ctrl Pts',(26.6565900458734,64.4304764207694,205.059501408952));
#34034=CARTESIAN_POINT('Ctrl Pts',(26.5564917553633,64.6169004300252,205.074923070535));
#34035=CARTESIAN_POINT('Ctrl Pts',(26.2875593368092,64.9436732159463,205.105362843473));
#34036=CARTESIAN_POINT('Ctrl Pts',(26.1202033059179,65.079700803322,205.119519802533));
#34037=CARTESIAN_POINT('Ctrl Pts',(25.750203601821,65.2737935921837,205.146498947623));
#34038=CARTESIAN_POINT('Ctrl Pts',(25.5527707440558,65.3331547757878,205.160895093502));
#34039=CARTESIAN_POINT('Ctrl Pts',(25.1384330669027,65.3752362020112,205.191107215795));
#34040=CARTESIAN_POINT('Ctrl Pts',(24.9251015083622,65.3544607625124,205.206662641938));
#34041=CARTESIAN_POINT('Ctrl Pts',(24.5248014746044,65.2326268377833,205.235851186066));
#34042=CARTESIAN_POINT('Ctrl Pts',(24.3410901005411,65.1350814473227,205.248331950634));
#34043=CARTESIAN_POINT('Ctrl Pts',(24.0202528598094,64.8752302082374,205.276438146074));
#34044=CARTESIAN_POINT('Ctrl Pts',(23.8863674965984,64.7152428409624,205.291422215258));
#34045=CARTESIAN_POINT('Ctrl Pts',(23.6841475426842,64.3483194106581,205.321965183195));
#34046=CARTESIAN_POINT('Ctrl Pts',(23.6196773382549,64.1437908321096,205.337231165791));
#34047=CARTESIAN_POINT('Ctrl Pts',(23.5753843646266,63.7308116046127,205.364924696244));
#34048=CARTESIAN_POINT('Ctrl Pts',(23.5923207633707,63.5267683405508,205.377514176774));
#34049=CARTESIAN_POINT('Ctrl Pts',(23.7032532954711,63.1298976168921,205.406620059725));
#34050=CARTESIAN_POINT('Ctrl Pts',(23.7984631158282,62.9415166825513,205.421987071124));
#34051=CARTESIAN_POINT('Ctrl Pts',(24.0579518435671,62.6094589432977,205.452416275407));
#34052=CARTESIAN_POINT('Ctrl Pts',(24.2206455088039,62.4699263013444,205.466970770937));
#34053=CARTESIAN_POINT('Ctrl Pts',(24.5834595825425,62.2665954546379,205.493425963814));
#34054=CARTESIAN_POINT('Ctrl Pts',(24.7785885703373,62.2018704889865,205.507654119174));
#34055=CARTESIAN_POINT('Ctrl Pts',(25.1903750294395,62.1480495849174,205.53768021515));
#34056=CARTESIAN_POINT('Ctrl Pts',(25.4035895306318,62.162521074076,205.553227105862));
#34057=CARTESIAN_POINT('Ctrl Pts',(25.808060349869,62.2725278142357,205.582719769765));
#34058=CARTESIAN_POINT('Ctrl Pts',(25.9957351330192,62.365391979812,205.595427499058));
#34059=CARTESIAN_POINT('Ctrl Pts',(26.3241902244079,62.6168371572382,205.623280605298));
#34060=CARTESIAN_POINT('Ctrl Pts',(26.4621032687503,62.7725947548537,205.638144416858));
#34061=CARTESIAN_POINT('Ctrl Pts',(26.6753613579213,63.134792561137,205.668791404589));
#34062=CARTESIAN_POINT('Ctrl Pts',(26.7459013793187,63.3394024204981,205.684283815291));
#34063=CARTESIAN_POINT('Ctrl Pts',(26.7832934753234,63.6216637007897,205.703471215402));
#34064=CARTESIAN_POINT('Ctrl Pts',(26.787903481163,63.6918511368568,205.708071462684));
#34065=CARTESIAN_POINT('Ctrl Pts',(26.787903481163,63.7619809500986,205.712499998088));
#34066=CARTESIAN_POINT('Ctrl Pts',(26.787903481163,63.7619809500998,205.8));
#34067=CARTESIAN_POINT('Ctrl Pts',(26.787903481163,63.5970233741762,205.789583310843));
#34068=CARTESIAN_POINT('Ctrl Pts',(26.7624058873089,63.4328282096167,205.778285166423));
#34069=CARTESIAN_POINT('Ctrl Pts',(26.6479661573429,63.0745487504577,205.751488365924));
#34070=CARTESIAN_POINT('Ctrl Pts',(26.5449154109998,62.8885614447829,205.735986639542));
#34071=CARTESIAN_POINT('Ctrl Pts',(26.2775921062976,62.5729472280983,205.706310170037));
#34072=CARTESIAN_POINT('Ctrl Pts',(26.1181448497944,62.4444819806854,205.692830099796));
#34073=CARTESIAN_POINT('Ctrl Pts',(25.7515596033761,62.2495753769853,205.666099925578));
#34074=CARTESIAN_POINT('Ctrl Pts',(25.5461691738736,62.1882350393232,205.651123540093));
#34075=CARTESIAN_POINT('Ctrl Pts',(25.1276467643565,62.1496308905272,205.620606281066));
#34076=CARTESIAN_POINT('Ctrl Pts',(24.918658424567,62.1711234328677,205.605367547956));
#34077=CARTESIAN_POINT('Ctrl Pts',(24.5247831157029,62.2916763130284,205.576647473352));
#34078=CARTESIAN_POINT('Ctrl Pts',(24.3431771222327,62.3879519502523,205.564302769579));
#34079=CARTESIAN_POINT('Ctrl Pts',(24.0179167377481,62.6498417170116,205.535906585384));
#34080=CARTESIAN_POINT('Ctrl Pts',(23.879954869629,62.815956019104,205.520386991871));
#34081=CARTESIAN_POINT('Ctrl Pts',(23.6813225898408,63.1853472172947,205.489818990723));
#34082=CARTESIAN_POINT('Ctrl Pts',(23.6197340287676,63.3836006133469,205.475054331292));
#34083=CARTESIAN_POINT('Ctrl Pts',(23.5747029995119,63.7955512694772,205.447398844463));
#34084=CARTESIAN_POINT('Ctrl Pts',(23.592813039977,64.0053928116448,205.434450109941));
#34085=CARTESIAN_POINT('Ctrl Pts',(23.7093125159563,64.4087873729732,205.404729300244));
#34086=CARTESIAN_POINT('Ctrl Pts',(23.8074847528848,64.5980587590194,205.38919805411));
#34087=CARTESIAN_POINT('Ctrl Pts',(24.066806173323,64.9215175853985,205.35931795102));
#34088=CARTESIAN_POINT('Ctrl Pts',(24.2230824675475,65.0544215778394,205.345351532243));
#34089=CARTESIAN_POINT('Ctrl Pts',(24.5846647970463,65.2590333925237,205.31898615405));
#34090=CARTESIAN_POINT('Ctrl Pts',(24.7883290378769,65.325742780325,205.30413563649));
#34091=CARTESIAN_POINT('Ctrl Pts',(25.206170580613,65.3754218477422,205.273668023998));
#34092=CARTESIAN_POINT('Ctrl Pts',(25.4161852664744,65.3592991558818,205.258354453154));
#34093=CARTESIAN_POINT('Ctrl Pts',(25.813009319228,65.2487766509945,205.229419365974));
#34094=CARTESIAN_POINT('Ctrl Pts',(25.9965736972429,65.1574589524346,205.216971771321));
#34095=CARTESIAN_POINT('Ctrl Pts',(26.328652143562,64.9041968716601,205.188871830358));
#34096=CARTESIAN_POINT('Ctrl Pts',(26.47123358898,64.7412633654917,205.173384674657));
#34097=CARTESIAN_POINT('Ctrl Pts',(26.6796688485015,64.3760948031904,205.14272592289));
#34098=CARTESIAN_POINT('Ctrl Pts',(26.7463232059866,64.1789448892568,205.127846255308));
#34099=CARTESIAN_POINT('Ctrl Pts',(26.7831857238628,63.903931748119,205.109135865945));
#34100=CARTESIAN_POINT('Ctrl Pts',(26.787903481163,63.8329256088025,205.104479991009));
#34101=CARTESIAN_POINT('Ctrl Pts',(26.787903481163,63.7619809500994,205.1));
#34102=CARTESIAN_POINT('Origin',(25.187903481163,63.761980950099,212.5));
#34103=CARTESIAN_POINT('',(26.787903481163,63.7619809500991,206.5));
#34104=CARTESIAN_POINT('',(26.787903481163,63.761980950099,206.412499998088));
#34105=CARTESIAN_POINT('',(26.787903481163,63.761980950099,212.5));
#34106=CARTESIAN_POINT('Ctrl Pts',(26.787903481163,63.7619809500986,205.712499998088));
#34107=CARTESIAN_POINT('Ctrl Pts',(26.787903481163,63.8943329583833,205.720857721108));
#34108=CARTESIAN_POINT('Ctrl Pts',(26.7714895796679,64.0264035874911,205.729796099176));
#34109=CARTESIAN_POINT('Ctrl Pts',(26.6875572351756,64.3574180908798,205.753758932389));
#34110=CARTESIAN_POINT('Ctrl Pts',(26.5972506194736,64.547623366758,205.769062384064));
#34111=CARTESIAN_POINT('Ctrl Pts',(26.3466230602689,64.8855389928907,205.79953843691));
#34112=CARTESIAN_POINT('Ctrl Pts',(26.1875546066788,65.0291679766956,205.81440764554));
#34113=CARTESIAN_POINT('Ctrl Pts',(25.8304058009002,65.241321917776,205.84082572614));
#34114=CARTESIAN_POINT('Ctrl Pts',(25.6374980048513,65.3109227042223,205.854717064069));
#34115=CARTESIAN_POINT('Ctrl Pts',(25.228111480123,65.3753410156036,205.884568164831));
#34116=CARTESIAN_POINT('Ctrl Pts',(25.0151601440169,65.3665725658219,205.900095866422));
#34117=CARTESIAN_POINT('Ctrl Pts',(24.6070218134671,65.2673819279788,205.929855953024));
#34118=CARTESIAN_POINT('Ctrl Pts',(24.4156909879703,65.1787807864123,205.942852614483));
#34119=CARTESIAN_POINT('Ctrl Pts',(24.0804425802019,64.934937537628,205.970473349515));
#34120=CARTESIAN_POINT('Ctrl Pts',(23.9390334905256,64.7830516539203,205.985220131289));
#34121=CARTESIAN_POINT('Ctrl Pts',(23.7171878133876,64.4273026847945,206.015772979022));
#34122=CARTESIAN_POINT('Ctrl Pts',(23.641561420083,64.2251364785299,206.031296519329));
#34123=CARTESIAN_POINT('Ctrl Pts',(23.5757688024019,63.812753944709,206.059736211146));
#34124=CARTESIAN_POINT('Ctrl Pts',(23.5824097134815,63.6072193302805,206.0720725426));
#34125=CARTESIAN_POINT('Ctrl Pts',(23.673441865874,63.2054789145064,206.100760400662));
#34126=CARTESIAN_POINT('Ctrl Pts',(23.7585569011475,63.0134896037899,206.115987233639));
#34127=CARTESIAN_POINT('Ctrl Pts',(23.9998699983602,62.6694564915045,206.146510001817));
#34128=CARTESIAN_POINT('Ctrl Pts',(24.1551180635514,62.5216441805762,206.161504092879));
#34129=CARTESIAN_POINT('Ctrl Pts',(24.5063252799646,62.3002726608011,206.188287621796));
#34130=CARTESIAN_POINT('Ctrl Pts',(24.6969757788931,62.2256880415114,206.201703186464));
#34131=CARTESIAN_POINT('Ctrl Pts',(25.1035511492808,62.1504001046736,206.231349307222));
#34132=CARTESIAN_POINT('Ctrl Pts',(25.316073602482,62.153291142219,206.246845736101));
#34133=CARTESIAN_POINT('Ctrl Pts',(25.7278845395229,62.2412021115542,206.276873616927));
#34134=CARTESIAN_POINT('Ctrl Pts',(25.9230557098139,62.3253657306034,206.290250163416));
#34135=CARTESIAN_POINT('Ctrl Pts',(26.2652195901742,62.5613652067408,206.317627708963));
#34136=CARTESIAN_POINT('Ctrl Pts',(26.410089584138,62.7092175623087,206.332245961572));
#34137=CARTESIAN_POINT('Ctrl Pts',(26.6405135656668,63.0581766093192,206.362682792118));
#34138=CARTESIAN_POINT('Ctrl Pts',(26.7212541523886,63.2577222668339,206.378227305805));
#34139=CARTESIAN_POINT('Ctrl Pts',(26.7787804698014,63.564663052373,206.399707219712));
#34140=CARTESIAN_POINT('Ctrl Pts',(26.787903481163,63.663318335078,206.406269682285));
#34141=CARTESIAN_POINT('Ctrl Pts',(26.787903481163,63.761980950099,206.412499998088));
#34142=CARTESIAN_POINT('Ctrl Pts',(26.787903481163,63.7619809500991,206.5));
#34143=CARTESIAN_POINT('Ctrl Pts',(26.787903481163,63.5675038931425,206.487719223933));
#34144=CARTESIAN_POINT('Ctrl Pts',(26.7524551032464,63.3744595409921,206.47423653108));
#34145=CARTESIAN_POINT('Ctrl Pts',(26.6084762635081,62.9965740307621,206.44512470712));
#34146=CARTESIAN_POINT('Ctrl Pts',(26.4961791586905,62.8173669190952,206.429714027479));
#34147=CARTESIAN_POINT('Ctrl Pts',(26.2134448205049,62.5172247748368,206.400452722944));
#34148=CARTESIAN_POINT('Ctrl Pts',(26.0475956006242,62.3974101336151,206.387685883711));
#34149=CARTESIAN_POINT('Ctrl Pts',(25.6712876897652,62.222031513499,206.36024676521));
#34150=CARTESIAN_POINT('Ctrl Pts',(25.462886059874,62.1715568643892,206.345050813031));
#34151=CARTESIAN_POINT('Ctrl Pts',(25.0438888044796,62.155081948558,206.314498929825));
#34152=CARTESIAN_POINT('Ctrl Pts',(24.8373549273612,62.1871777057293,206.299439167952));
#34153=CARTESIAN_POINT('Ctrl Pts',(24.4495807953107,62.3277374308245,206.271163970823));
#34154=CARTESIAN_POINT('Ctrl Pts',(24.2718327392805,62.4342039840849,206.258780963389));
#34155=CARTESIAN_POINT('Ctrl Pts',(23.9607494916364,62.7134916629651,206.229803016088));
#34156=CARTESIAN_POINT('Ctrl Pts',(23.8324132049372,62.8857034299824,206.214249314432));
#34157=CARTESIAN_POINT('Ctrl Pts',(23.6540181241615,63.2629139046671,206.183925358617));
#34158=CARTESIAN_POINT('Ctrl Pts',(23.6028055180387,63.4630195624287,206.169422023171));
#34159=CARTESIAN_POINT('Ctrl Pts',(23.5781678571076,63.8790318357696,206.142253562835));
#34160=CARTESIAN_POINT('Ctrl Pts',(23.6078144084343,64.0911015451921,206.128490876883));
#34161=CARTESIAN_POINT('Ctrl Pts',(23.7474692652303,64.4894792931328,206.098242660748));
#34162=CARTESIAN_POINT('Ctrl Pts',(23.8552907363838,64.672063101578,206.082781924664));
#34163=CARTESIAN_POINT('Ctrl Pts',(24.1305191199193,64.979800405088,206.053314657996));
#34164=CARTESIAN_POINT('Ctrl Pts',(24.2931987402541,65.1038466447376,206.040238887358));
#34165=CARTESIAN_POINT('Ctrl Pts',(24.6647590825583,65.2888774183122,206.013145945732));
#34166=CARTESIAN_POINT('Ctrl Pts',(24.8717496356647,65.3447302249742,205.998052884568));
#34167=CARTESIAN_POINT('Ctrl Pts',(25.2906602783368,65.3721118293582,205.967507316873));
#34168=CARTESIAN_POINT('Ctrl Pts',(25.4984710074416,65.3452210672238,205.952354451209));
#34169=CARTESIAN_POINT('Ctrl Pts',(25.8892867413197,65.2145216848601,205.923857470614));
#34170=CARTESIAN_POINT('Ctrl Pts',(26.0689326881062,65.1131282902506,205.91153430439));
#34171=CARTESIAN_POINT('Ctrl Pts',(26.3871001166582,64.8424457137608,205.882841471962));
#34172=CARTESIAN_POINT('Ctrl Pts',(26.5202476112438,64.6731947633831,205.867299330404));
#34173=CARTESIAN_POINT('Ctrl Pts',(26.708726986369,64.2997320722016,205.836844381879));
#34174=CARTESIAN_POINT('Ctrl Pts',(26.7650964196516,64.1004789522881,205.822206872901));
#34175=CARTESIAN_POINT('Ctrl Pts',(26.7860341842952,63.8513374056493,205.805710804818));
#34176=CARTESIAN_POINT('Ctrl Pts',(26.787903481163,63.8066355290279,205.802819833315));
#34177=CARTESIAN_POINT('Ctrl Pts',(26.787903481163,63.7619809500998,205.8));
#34178=CARTESIAN_POINT('Origin',(25.187903481163,63.761980950099,212.5));
#34179=CARTESIAN_POINT('',(26.787903481163,63.761980950099,207.2));
#34180=CARTESIAN_POINT('',(26.787903481163,63.7619809500991,207.112499998088));
#34181=CARTESIAN_POINT('',(26.787903481163,63.761980950099,212.5));
#34182=CARTESIAN_POINT('Ctrl Pts',(26.787903481163,63.761980950099,206.412499998088));
#34183=CARTESIAN_POINT('Ctrl Pts',(26.787903481163,63.8669814833784,206.419130538761));
#34184=CARTESIAN_POINT('Ctrl Pts',(26.7775710896497,63.9719422841774,206.426135272194));
#34185=CARTESIAN_POINT('Ctrl Pts',(26.7162585214528,64.2788956428125,206.447754020456));
#34186=CARTESIAN_POINT('Ctrl Pts',(26.636403592699,64.4725410986798,206.46289366045));
#34187=CARTESIAN_POINT('Ctrl Pts',(26.404622379655,64.822474271555,206.49344148719));
#34188=CARTESIAN_POINT('Ctrl Pts',(26.2533371620173,64.9743941693603,206.50855048404));
#34189=CARTESIAN_POINT('Ctrl Pts',(25.9081985957982,65.2049896057789,206.535695229074));
#34190=CARTESIAN_POINT('Ctrl Pts',(25.7197445976187,65.2845731385076,206.54871991668));
#34191=CARTESIAN_POINT('Ctrl Pts',(25.3160393231562,65.3705995212323,206.578156759609));
#34192=CARTESIAN_POINT('Ctrl Pts',(25.1040997470756,65.3735165796787,206.593610687032));
#34193=CARTESIAN_POINT('Ctrl Pts',(24.688769231921,65.2969019717223,206.623895203762));
#34194=CARTESIAN_POINT('Ctrl Pts',(24.4897287899226,65.2171834336825,206.63772828132));
#34195=CARTESIAN_POINT('Ctrl Pts',(24.140805289395,64.9889568079691,206.664861433838));
#34196=CARTESIAN_POINT('Ctrl Pts',(23.9926525128375,64.845132739593,206.679344994215));
#34197=CARTESIAN_POINT('Ctrl Pts',(23.7540140389359,64.5030234563659,206.709648764732));
#34198=CARTESIAN_POINT('Ctrl Pts',(23.6683427684131,64.3061666030387,206.72520325117));
#34199=CARTESIAN_POINT('Ctrl Pts',(23.5804518451138,63.897386451111,206.7542211283));
#34200=CARTESIAN_POINT('Ctrl Pts',(23.5763626287985,63.6900886543587,206.766619069941));
#34201=CARTESIAN_POINT('Ctrl Pts',(23.6470998404387,63.2836673668123,206.794862594507));
#34202=CARTESIAN_POINT('Ctrl Pts',(23.7218432357729,63.0885556424707,206.809908467972));
#34203=CARTESIAN_POINT('Ctrl Pts',(23.9442727309352,62.7331715354191,206.840459560542));
#34204=CARTESIAN_POINT('Ctrl Pts',(24.0916199902306,62.5773845806502,206.855669181692));
#34205=CARTESIAN_POINT('Ctrl Pts',(24.4308048030734,62.337925159989,206.883156602892));
#34206=CARTESIAN_POINT('Ctrl Pts',(24.6172038270259,62.2535174294369,206.895886481641));
#34207=CARTESIAN_POINT('Ctrl Pts',(25.0181007102128,62.1572951481852,206.92511854604));
#34208=CARTESIAN_POINT('Ctrl Pts',(25.2293396512559,62.1488703535295,206.940521385491));
#34209=CARTESIAN_POINT('Ctrl Pts',(25.6479031546538,62.2146190616609,206.971041640947));
#34210=CARTESIAN_POINT('Ctrl Pts',(25.8506822506942,62.290052850919,206.985381621091));
#34211=CARTESIAN_POINT('Ctrl Pts',(26.2059569395127,62.5108773418095,207.012278899665));
#34212=CARTESIAN_POINT('Ctrl Pts',(26.3571003183097,62.6508431118903,207.026627849807));
#34213=CARTESIAN_POINT('Ctrl Pts',(26.6032945590545,62.9863308225324,207.056788954007));
#34214=CARTESIAN_POINT('Ctrl Pts',(26.6935320133216,63.1805488813184,207.072343282125));
#34215=CARTESIAN_POINT('Ctrl Pts',(26.7729929267595,63.5098955615491,207.096037775242));
#34216=CARTESIAN_POINT('Ctrl Pts',(26.787903481163,63.6358376355474,207.104534339709));
#34217=CARTESIAN_POINT('Ctrl Pts',(26.787903481163,63.7619809500992,207.112499998088));
#34218=CARTESIAN_POINT('Ctrl Pts',(26.787903481163,63.761980950099,207.2));
#34219=CARTESIAN_POINT('Ctrl Pts',(26.787903481163,63.7525522129429,207.19940459707));
#34220=CARTESIAN_POINT('Ctrl Pts',(26.7878201364588,63.7431204336134,207.198805963424));
#34221=CARTESIAN_POINT('Ctrl Pts',(26.783899104122,63.5214261680704,207.18466352932));
#34222=CARTESIAN_POINT('Ctrl Pts',(26.7379395030619,63.3120852737804,207.169768525869));
#34223=CARTESIAN_POINT('Ctrl Pts',(26.5686100509296,62.9270568821559,207.139281404403));
#34224=CARTESIAN_POINT('Ctrl Pts',(26.4482055279597,62.7544583317913,207.12399245716));
#34225=CARTESIAN_POINT('Ctrl Pts',(26.1515917254345,62.4686574751092,207.095130749608));
#34226=CARTESIAN_POINT('Ctrl Pts',(25.9795960393133,62.3567786095062,207.082727582365));
#34227=CARTESIAN_POINT('Ctrl Pts',(25.5928230113361,62.1993160111005,207.054525382408));
#34228=CARTESIAN_POINT('Ctrl Pts',(25.3802594249269,62.1592184000023,207.039025954233));
#34229=CARTESIAN_POINT('Ctrl Pts',(24.9601931890366,62.1649284522877,207.008396124532));
#34230=CARTESIAN_POINT('Ctrl Pts',(24.7566557848746,62.2074757222851,206.993554855479));
#34231=CARTESIAN_POINT('Ctrl Pts',(24.3752971863953,62.3681255968876,206.965747457673));
#34232=CARTESIAN_POINT('Ctrl Pts',(24.2014062596625,62.4852668188097,206.952988831481));
#34233=CARTESIAN_POINT('Ctrl Pts',(23.9053806152225,62.7822461340029,206.923442673408));
#34234=CARTESIAN_POINT('Ctrl Pts',(23.787237955169,62.9601889469858,206.907898712102));
#34235=CARTESIAN_POINT('Ctrl Pts',(23.6300151410848,63.3443378617583,206.877908515409));
#34236=CARTESIAN_POINT('Ctrl Pts',(23.5895443702116,63.5457925868411,206.863711618893));
#34237=CARTESIAN_POINT('Ctrl Pts',(23.5862946558477,63.9615614157298,206.837338300396));
#34238=CARTESIAN_POINT('Ctrl Pts',(23.6268246611896,64.1720148428447,206.822688307262));
#34239=CARTESIAN_POINT('Ctrl Pts',(23.7865399355414,64.5618837336842,206.792246036372));
#34240=CARTESIAN_POINT('Ctrl Pts',(23.902876632678,64.7378807497438,206.776890790036));
#34241=CARTESIAN_POINT('Ctrl Pts',(24.1924756760677,65.0309779785475,206.747824079897));
#34242=CARTESIAN_POINT('Ctrl Pts',(24.3613164130033,65.1468874283103,206.73527197372));
#34243=CARTESIAN_POINT('Ctrl Pts',(24.7419805000195,65.3131954482369,206.707515217375));
#34244=CARTESIAN_POINT('Ctrl Pts',(24.9515707329539,65.3586099066965,206.692232596224));
#34245=CARTESIAN_POINT('Ctrl Pts',(25.3703900120067,65.3649041147617,206.661693690459));
#34246=CARTESIAN_POINT('Ctrl Pts',(25.5756143073771,65.3279862975776,206.646729418922));
#34247=CARTESIAN_POINT('Ctrl Pts',(25.9604830027105,65.1782107334265,206.618666076554));
#34248=CARTESIAN_POINT('Ctrl Pts',(26.1364608790847,65.0669067939199,206.606153558572));
#34249=CARTESIAN_POINT('Ctrl Pts',(26.440744275318,64.7795277983336,206.576912574596));
#34250=CARTESIAN_POINT('Ctrl Pts',(26.5644684661065,64.6046341242401,206.561357666046));
#34251=CARTESIAN_POINT('Ctrl Pts',(26.7332524044497,64.2241199869409,206.531175497817));
#34252=CARTESIAN_POINT('Ctrl Pts',(26.7795746640885,64.0233289589085,206.516807176706));
#34253=CARTESIAN_POINT('Ctrl Pts',(26.7875627091774,63.8001241285047,206.50242107742));
#34254=CARTESIAN_POINT('Ctrl Pts',(26.787903481163,63.7810464245148,206.501203940586));
#34255=CARTESIAN_POINT('Ctrl Pts',(26.787903481163,63.7619809500991,206.5));
#34256=CARTESIAN_POINT('Origin',(25.187903481163,63.761980950099,212.5));
#34257=CARTESIAN_POINT('',(26.787903481163,63.7619809500987,207.9));
#34258=CARTESIAN_POINT('',(26.787903481163,63.7619809500993,207.812499998088));
#34259=CARTESIAN_POINT('',(26.787903481163,63.761980950099,212.5));
#34260=CARTESIAN_POINT('Ctrl Pts',(26.787903481163,63.7619809500992,207.112499998088));
#34261=CARTESIAN_POINT('Ctrl Pts',(26.787903481163,63.8414450419085,207.117517971582));
#34262=CARTESIAN_POINT('Ctrl Pts',(26.7819848945636,63.9209615052248,207.122755034017));
#34263=CARTESIAN_POINT('Ctrl Pts',(26.7394037831285,64.204148469419,207.142190071779));
#34264=CARTESIAN_POINT('Ctrl Pts',(26.6694314194012,64.4005037511713,207.157140529156));
#34265=CARTESIAN_POINT('Ctrl Pts',(26.4558083281594,64.7607282463888,207.187676214227));
#34266=CARTESIAN_POINT('Ctrl Pts',(26.3122128226757,64.9200152164406,207.202970070551));
#34267=CARTESIAN_POINT('Ctrl Pts',(25.9786438161088,65.1676690187884,207.230770205053));
#34268=CARTESIAN_POINT('Ctrl Pts',(25.7940990874182,65.2565620664902,207.243298235132));
#34269=CARTESIAN_POINT('Ctrl Pts',(25.395840262536,65.3621086082077,207.272337941113));
#34270=CARTESIAN_POINT('Ctrl Pts',(25.1853676245001,65.3755574371444,207.287684904303));
#34271=CARTESIAN_POINT('Ctrl Pts',(24.7677560754606,65.3203677089534,207.318135746421));
#34272=CARTESIAN_POINT('Ctrl Pts',(24.5650041381801,65.2509311543605,207.332852777124));
#34273=CARTESIAN_POINT('Ctrl Pts',(24.2059193595989,65.0414997397462,207.35916951882));
#34274=CARTESIAN_POINT('Ctrl Pts',(24.0512725597523,64.9063076011827,207.373344754072));
#34275=CARTESIAN_POINT('Ctrl Pts',(23.7961294931413,64.5790903688926,207.40330985598));
#34276=CARTESIAN_POINT('Ctrl Pts',(23.7004427116352,64.3882183961412,207.418851559899));
#34277=CARTESIAN_POINT('Ctrl Pts',(23.5897447945303,63.9836613539396,207.448434262406));
#34278=CARTESIAN_POINT('Ctrl Pts',(23.5744955769871,63.7743576134366,207.461229610602));
#34279=CARTESIAN_POINT('Ctrl Pts',(23.6246916716907,63.3634812780015,207.489005566243));
#34280=CARTESIAN_POINT('Ctrl Pts',(23.6889197287988,63.1657863788744,207.503831189512));
#34281=CARTESIAN_POINT('Ctrl Pts',(23.8926661586705,62.7985618703457,207.534448822611));
#34282=CARTESIAN_POINT('Ctrl Pts',(24.0330416160228,62.634088036499,207.549952819791));
#34283=CARTESIAN_POINT('Ctrl Pts',(24.3618619747844,62.3766815978009,207.578195682924));
#34284=CARTESIAN_POINT('Ctrl Pts',(24.5444809220034,62.282989638787,207.590583769816));
#34285=CARTESIAN_POINT('Ctrl Pts',(24.9398951216553,62.1676393644531,207.619416055207));
#34286=CARTESIAN_POINT('Ctrl Pts',(25.149432996067,62.148928426027,207.63469485855));
#34287=CARTESIAN_POINT('Ctrl Pts',(25.5676390031476,62.1932803902761,207.665189046566));
#34288=CARTESIAN_POINT('Ctrl Pts',(25.7721517899316,62.2574129880585,207.680101437269));
#34289=CARTESIAN_POINT('Ctrl Pts',(26.1361523885087,62.4573606483448,207.706643147582));
#34290=CARTESIAN_POINT('Ctrl Pts',(26.2939522590617,62.5881190747884,207.720364699034));
#34291=CARTESIAN_POINT('Ctrl Pts',(26.5563272541312,62.90679721156,207.75005424088));
#34292=CARTESIAN_POINT('Ctrl Pts',(26.6564631834237,63.0932056096546,207.765476288902));
#34293=CARTESIAN_POINT('Ctrl Pts',(26.764364701095,63.4456647291453,207.791667176098));
#34294=CARTESIAN_POINT('Ctrl Pts',(26.787903481163,63.6034854768915,207.802491375762));
#34295=CARTESIAN_POINT('Ctrl Pts',(26.787903481163,63.7619809500997,207.812499998088));
#34296=CARTESIAN_POINT('Ctrl Pts',(26.787903481163,63.7619809500984,207.9));
#34297=CARTESIAN_POINT('Ctrl Pts',(26.787903481163,63.7243079680956,207.897621038373));
#34298=CARTESIAN_POINT('Ctrl Pts',(26.7865729824725,63.6865997397188,207.895191343255));
#34299=CARTESIAN_POINT('Ctrl Pts',(26.7688988089106,63.437094806524,207.878791313244));
#34300=CARTESIAN_POINT('Ctrl Pts',(26.7118745467737,63.2304111462137,207.863660708868));
#34301=CARTESIAN_POINT('Ctrl Pts',(26.5227629248067,62.8558053002262,207.833110522096));
#34302=CARTESIAN_POINT('Ctrl Pts',(26.3941907240463,62.6905811369211,207.81798947041));
#34303=CARTESIAN_POINT('Ctrl Pts',(26.0831113321561,62.420141149911,207.789570374949));
#34304=CARTESIAN_POINT('Ctrl Pts',(25.9042701815625,62.3167301764244,207.777235071904));
#34305=CARTESIAN_POINT('Ctrl Pts',(25.5093829261866,62.1801962118329,207.748441209533));
#34306=CARTESIAN_POINT('Ctrl Pts',(25.2961612486276,62.151500057009,207.732893795544));
#34307=CARTESIAN_POINT('Ctrl Pts',(24.8790950172265,62.1787423660481,207.702482716171));
#34308=CARTESIAN_POINT('Ctrl Pts',(24.6789856363008,62.2312788529102,207.687891407145));
#34309=CARTESIAN_POINT('Ctrl Pts',(24.3042032141398,62.4115984513379,207.660563522196));
#34310=CARTESIAN_POINT('Ctrl Pts',(24.134119969933,62.539672230542,207.647100109662));
#34311=CARTESIAN_POINT('Ctrl Pts',(23.853707430182,62.8541361711949,207.617019065731));
#34312=CARTESIAN_POINT('Ctrl Pts',(23.7460247799713,63.0372425981383,207.601530388678));
#34313=CARTESIAN_POINT('Ctrl Pts',(23.6101306899241,63.4275875000795,207.571926539466));
#34314=CARTESIAN_POINT('Ctrl Pts',(23.5805037377593,63.6301046122382,207.558597467845));
#34315=CARTESIAN_POINT('Ctrl Pts',(23.5988520001172,64.0448225402752,207.531740043409));
#34316=CARTESIAN_POINT('Ctrl Pts',(23.650364647311,64.2529100046123,207.516721736352));
#34317=CARTESIAN_POINT('Ctrl Pts',(23.8296670976769,64.6328538193687,207.486192095254));
#34318=CARTESIAN_POINT('Ctrl Pts',(23.9542111062302,64.8018112950849,207.470982154704));
#34319=CARTESIAN_POINT('Ctrl Pts',(24.2580861321395,65.0799549433225,207.442339250041));
#34320=CARTESIAN_POINT('Ctrl Pts',(24.4334586852997,65.1876122169457,207.430011599698));
#34321=CARTESIAN_POINT('Ctrl Pts',(24.8243161172515,65.3346987298797,207.401511578619));
#34322=CARTESIAN_POINT('Ctrl Pts',(25.0372805304777,65.3691279381029,207.385982923488));
#34323=CARTESIAN_POINT('Ctrl Pts',(25.4559918902457,65.3526875099004,207.355451886838));
#34324=CARTESIAN_POINT('Ctrl Pts',(25.657887576413,65.30514962692,207.340730326388));
#34325=CARTESIAN_POINT('Ctrl Pts',(26.0360195067286,65.1347384234157,207.313158206469));
#34326=CARTESIAN_POINT('Ctrl Pts',(26.2080294593705,65.0122333167422,207.300091783863));
#34327=CARTESIAN_POINT('Ctrl Pts',(26.496418568369,64.7065938874235,207.27027717498));
#34328=CARTESIAN_POINT('Ctrl Pts',(26.6094271514754,64.5260291333446,207.254754824049));
#34329=CARTESIAN_POINT('Ctrl Pts',(26.7528126375547,64.1475032009327,207.225624191596));
#34330=CARTESIAN_POINT('Ctrl Pts',(26.787903481163,63.9554620586892,207.212217884233));
#34331=CARTESIAN_POINT('Ctrl Pts',(26.787903481163,63.761980950099,207.2));
#34332=CARTESIAN_POINT('Origin',(25.187903481163,63.761980950099,212.5));
#34333=CARTESIAN_POINT('',(26.787903481163,63.7619809500988,208.6));
#34334=CARTESIAN_POINT('',(26.787903481163,63.761980950099,208.512499998088));
#34335=CARTESIAN_POINT('',(26.787903481163,63.761980950099,212.5));
#34336=CARTESIAN_POINT('Ctrl Pts',(26.787903481163,63.7619809500997,207.812499998088));
#34337=CARTESIAN_POINT('Ctrl Pts',(26.787903481163,63.8056642480145,207.815258497255));
#34338=CARTESIAN_POINT('Ctrl Pts',(26.7861146165017,63.8493905931841,207.81808493378));
#34339=CARTESIAN_POINT('Ctrl Pts',(26.7651281508763,64.1047120415683,207.834973023913));
#34340=CARTESIAN_POINT('Ctrl Pts',(26.705767618042,64.3107518492307,207.85014814702));
#34341=CARTESIAN_POINT('Ctrl Pts',(26.5125252086714,64.6830060953015,207.880700437324));
#34342=CARTESIAN_POINT('Ctrl Pts',(26.3822699050941,64.8466113004039,207.895780618669));
#34343=CARTESIAN_POINT('Ctrl Pts',(26.0681320770453,65.1137536200525,207.924102979553));
#34344=CARTESIAN_POINT('Ctrl Pts',(25.8877887905821,65.2153404598777,207.936466694276));
#34345=CARTESIAN_POINT('Ctrl Pts',(25.4911978350355,65.347320003828,207.965384784785));
#34346=CARTESIAN_POINT('Ctrl Pts',(25.2779114232912,65.3735529914763,207.980936918975));
#34347=CARTESIAN_POINT('Ctrl Pts',(24.8616369885109,65.3416854977625,208.011290263177));
#34348=CARTESIAN_POINT('Ctrl Pts',(24.662333987329,65.28701655059,208.02582277368));
#34349=CARTESIAN_POINT('Ctrl Pts',(24.2890188827847,65.1024255295337,208.05304366672));
#34350=CARTESIAN_POINT('Ctrl Pts',(24.1197742346218,64.9719118257991,208.06670454222));
#34351=CARTESIAN_POINT('Ctrl Pts',(23.8428723168436,64.6536350491948,208.096898366491));
#34352=CARTESIAN_POINT('Ctrl Pts',(23.737519834635,64.4694721685266,208.11236880211));
#34353=CARTESIAN_POINT('Ctrl Pts',(23.6063298640587,64.0778606163386,208.141881132998));
#34354=CARTESIAN_POINT('Ctrl Pts',(23.5790801805219,63.8750840617643,208.155036115506));
#34355=CARTESIAN_POINT('Ctrl Pts',(23.6022533838314,63.4606442276958,208.182051888257));
#34356=CARTESIAN_POINT('Ctrl Pts',(23.6561917661913,63.2531548067158,208.197120868521));
#34357=CARTESIAN_POINT('Ctrl Pts',(23.8398223974902,62.8755242290384,208.227662232314));
#34358=CARTESIAN_POINT('Ctrl Pts',(23.9661491818328,62.7081950422413,208.242834347222));
#34359=CARTESIAN_POINT('Ctrl Pts',(24.2731946119985,62.4334283554682,208.271379592238));
#34360=CARTESIAN_POINT('Ctrl Pts',(24.4500787049065,62.3276321216025,208.283700274819));
#34361=CARTESIAN_POINT('Ctrl Pts',(24.8427128071976,62.1851572893188,208.312329844778));
#34362=CARTESIAN_POINT('Ctrl Pts',(25.055808187246,62.15323793446,208.327868049573));
#34363=CARTESIAN_POINT('Ctrl Pts',(25.473833358999,62.1744135890098,208.35834905168));
#34364=CARTESIAN_POINT('Ctrl Pts',(25.674962606062,62.2241458580207,208.373014725945));
#34365=CARTESIAN_POINT('Ctrl Pts',(26.0516391923357,62.3988896184487,208.400480727028));
#34366=CARTESIAN_POINT('Ctrl Pts',(26.2228094273173,62.5238141254902,208.413710241233));
#34367=CARTESIAN_POINT('Ctrl Pts',(26.5077390647548,62.8333084000493,208.443642148105));
#34368=CARTESIAN_POINT('Ctrl Pts',(26.6184326947677,63.0149998441212,208.459151247569));
#34369=CARTESIAN_POINT('Ctrl Pts',(26.7550853208744,63.3890216421474,208.487751985506));
#34370=CARTESIAN_POINT('Ctrl Pts',(26.787903481163,63.5748601181481,208.500683750606));
#34371=CARTESIAN_POINT('Ctrl Pts',(26.787903481163,63.761980950099,208.512499998088));
#34372=CARTESIAN_POINT('Ctrl Pts',(26.787903481163,63.7619809500986,208.6));
#34373=CARTESIAN_POINT('Ctrl Pts',(26.787903481163,63.6903170416566,208.595474590034));
#34374=CARTESIAN_POINT('Ctrl Pts',(26.7830895983552,63.6185920864977,208.590769818965));
#34375=CARTESIAN_POINT('Ctrl Pts',(26.7457547260124,63.3428845494794,208.571998358854));
#34376=CARTESIAN_POINT('Ctrl Pts',(26.6788199082709,63.145799591795,208.557112567994));
#34377=CARTESIAN_POINT('Ctrl Pts',(26.4698434177921,62.7808726668203,208.526449342687));
#34378=CARTESIAN_POINT('Ctrl Pts',(26.3270077628508,62.6181192181451,208.510964289145));
#34379=CARTESIAN_POINT('Ctrl Pts',(25.9945535381211,62.3653376727936,208.482880992627));
#34380=CARTESIAN_POINT('Ctrl Pts',(25.8108789472433,62.2742944396459,208.470425294402));
#34381=CARTESIAN_POINT('Ctrl Pts',(25.4138922132662,62.1643328958762,208.441478345049));
#34382=CARTESIAN_POINT('Ctrl Pts',(25.2038241981467,62.1485113437469,208.426160885613));
#34383=CARTESIAN_POINT('Ctrl Pts',(24.7860294148133,62.1988088945462,208.395696682662));
#34384=CARTESIAN_POINT('Ctrl Pts',(24.5824658822676,62.2658167581286,208.380853508414));
#34385=CARTESIAN_POINT('Ctrl Pts',(24.2211657629679,62.4709696707996,208.354508708048));
#34386=CARTESIAN_POINT('Ctrl Pts',(24.0650662140339,62.6041240979823,208.340512538584));
#34387=CARTESIAN_POINT('Ctrl Pts',(23.807380615723,62.9265435585416,208.310757708387));
#34388=CARTESIAN_POINT('Ctrl Pts',(23.7100510270448,63.1140930482654,208.295365917533));
#34389=CARTESIAN_POINT('Ctrl Pts',(23.5949105617204,63.5098968986751,208.266173990926));
#34390=CARTESIAN_POINT('Ctrl Pts',(23.575820026113,63.7136565425895,208.253492117129));
#34391=CARTESIAN_POINT('Ctrl Pts',(23.6156799993393,64.1269759559357,208.225938724534));
#34392=CARTESIAN_POINT('Ctrl Pts',(23.6779527268435,64.3321719207942,208.210710714382));
#34393=CARTESIAN_POINT('Ctrl Pts',(23.8763213986302,64.7014197159999,208.180161379509));
#34394=CARTESIAN_POINT('Ctrl Pts',(24.0086542364851,64.8629760269156,208.165134837652));
#34395=CARTESIAN_POINT('Ctrl Pts',(24.3266082436035,65.1259766875288,208.136934881423));
#34396=CARTESIAN_POINT('Ctrl Pts',(24.5088567403975,65.2252694358942,208.124513824847));
#34397=CARTESIAN_POINT('Ctrl Pts',(24.9075646962965,65.3514986296844,208.09544136973));
#34398=CARTESIAN_POINT('Ctrl Pts',(25.1208933792387,65.3746331094214,208.079886153265));
#34399=CARTESIAN_POINT('Ctrl Pts',(25.5360991086036,65.3369609364821,208.049610735499));
#34400=CARTESIAN_POINT('Ctrl Pts',(25.7343544727492,65.2796224664386,208.035154615197));
#34401=CARTESIAN_POINT('Ctrl Pts',(26.1057984283124,65.0896437082546,208.008070160104));
#34402=CARTESIAN_POINT('Ctrl Pts',(26.2739765223907,64.9560181854706,207.994137608416));
#34403=CARTESIAN_POINT('Ctrl Pts',(26.5463869939338,64.6329260627183,207.963803456824));
#34404=CARTESIAN_POINT('Ctrl Pts',(26.6487719530388,64.4474657572087,207.948359282776));
#34405=CARTESIAN_POINT('Ctrl Pts',(26.7625332992819,64.0902789679199,207.921656214591));
#34406=CARTESIAN_POINT('Ctrl Pts',(26.7879034811631,63.9265241416833,207.910390521745));
#34407=CARTESIAN_POINT('Ctrl Pts',(26.787903481163,63.7619809500984,207.9));
#34408=CARTESIAN_POINT('Origin',(25.187903481163,63.761980950099,212.5));
#34409=CARTESIAN_POINT('',(26.787903481163,63.761980950099,209.3));
#34410=CARTESIAN_POINT('',(26.787903481163,63.761980950099,209.212499998088));
#34411=CARTESIAN_POINT('',(26.787903481163,63.761980950099,212.5));
#34412=CARTESIAN_POINT('Ctrl Pts',(26.787903481163,63.7619809500991,208.512499998088));
#34413=CARTESIAN_POINT('Ctrl Pts',(26.787903481163,63.7775474145994,208.513482984296));
#34414=CARTESIAN_POINT('Ctrl Pts',(26.7876763117769,63.7931217265644,208.51447474827));
#34415=CARTESIAN_POINT('Ctrl Pts',(26.781022091544,64.0209184771424,208.529102187656));
#34416=CARTESIAN_POINT('Ctrl Pts',(26.7326473328888,64.229733878515,208.544052060066));
#34417=CARTESIAN_POINT('Ctrl Pts',(26.5589693241796,64.61258673282,208.57456034251));
#34418=CARTESIAN_POINT('Ctrl Pts',(26.4367544896036,64.7836163848673,208.589816218399));
#34419=CARTESIAN_POINT('Ctrl Pts',(26.1369815391396,65.066098938011,208.618583560031));
#34420=CARTESIAN_POINT('Ctrl Pts',(25.9635309531092,65.1761477348963,208.630943828259));
#34421=CARTESIAN_POINT('Ctrl Pts',(25.5749786481579,65.3291274817817,208.659275767161));
#34422=CARTESIAN_POINT('Ctrl Pts',(25.3622237844917,65.3667728207009,208.674789142637));
#34423=CARTESIAN_POINT('Ctrl Pts',(24.9427105504864,65.3564144508637,208.705378649283));
#34424=CARTESIAN_POINT('Ctrl Pts',(24.7398682029649,65.3117022399689,208.720169237123));
#34425=CARTESIAN_POINT('Ctrl Pts',(24.3598955373424,65.1468328837485,208.747875577325));
#34426=CARTESIAN_POINT('Ctrl Pts',(24.1868162294044,65.0273876946373,208.760757130098));
#34427=CARTESIAN_POINT('Ctrl Pts',(23.8940651100409,64.7266694324474,208.790420010294));
#34428=CARTESIAN_POINT('Ctrl Pts',(23.7781276598159,64.5475793782385,208.805956018954));
#34429=CARTESIAN_POINT('Ctrl Pts',(23.6253804438905,64.1619200072396,208.835878424612));
#34430=CARTESIAN_POINT('Ctrl Pts',(23.5872736285872,63.9602324372348,208.849957912115));
#34431=CARTESIAN_POINT('Ctrl Pts',(23.5885773167067,63.5446904835471,208.876245955095));
#34432=CARTESIAN_POINT('Ctrl Pts',(23.6314779189152,63.3347270515375,208.891068744362));
#34433=CARTESIAN_POINT('Ctrl Pts',(23.7952752504989,62.9470217655082,208.921523213619));
#34434=CARTESIAN_POINT('Ctrl Pts',(23.913364966278,62.7724682616747,208.936851217637));
#34435=CARTESIAN_POINT('Ctrl Pts',(24.20597348562,62.482489234716,208.965830741023));
#34436=CARTESIAN_POINT('Ctrl Pts',(24.3761552541167,62.3683036891449,208.978310023199));
#34437=CARTESIAN_POINT('Ctrl Pts',(24.7606685283092,62.2052260923822,209.006347449443));
#34438=CARTESIAN_POINT('Ctrl Pts',(24.9729534744288,62.1620508183978,209.021826560097));
#34439=CARTESIAN_POINT('Ctrl Pts',(25.3936421928073,62.161913910055,209.052501779146));
#34440=CARTESIAN_POINT('Ctrl Pts',(25.5980191227873,62.2017314157506,209.067404263623));
#34441=CARTESIAN_POINT('Ctrl Pts',(25.9810962854264,62.3570914833136,209.095336973399));
#34442=CARTESIAN_POINT('Ctrl Pts',(26.1560028163382,62.4713752998897,209.107963193064));
#34443=CARTESIAN_POINT('Ctrl Pts',(26.4560776856708,62.7636778317421,209.137361651083));
#34444=CARTESIAN_POINT('Ctrl Pts',(26.5769540073409,62.9401536355283,209.152912638901));
#34445=CARTESIAN_POINT('Ctrl Pts',(26.739829675257,63.3225711041239,209.182999592404));
#34446=CARTESIAN_POINT('Ctrl Pts',(26.7831573581791,63.5237230098691,209.197281524831));
#34447=CARTESIAN_POINT('Ctrl Pts',(26.7877807320592,63.7390911262713,209.21105008346));
#34448=CARTESIAN_POINT('Ctrl Pts',(26.787903481163,63.7505383731459,209.211777425835));
#34449=CARTESIAN_POINT('Ctrl Pts',(26.787903481163,63.761980950099,209.212499998088));
#34450=CARTESIAN_POINT('Ctrl Pts',(26.787903481163,63.761980950099,209.3));
#34451=CARTESIAN_POINT('Ctrl Pts',(26.787903481163,63.6629707403392,209.293747734394));
#34452=CARTESIAN_POINT('Ctrl Pts',(26.7787160838662,63.5639686077502,209.287161021649));
#34453=CARTESIAN_POINT('Ctrl Pts',(26.7220086825207,63.2624852334651,209.266055586947));
#34454=CARTESIAN_POINT('Ctrl Pts',(26.6444624854735,63.0681602008647,209.250957205766));
#34455=CARTESIAN_POINT('Ctrl Pts',(26.416894414014,62.7157307945329,209.220405351781));
#34456=CARTESIAN_POINT('Ctrl Pts',(26.267377327109,62.5620491563593,209.205249568203));
#34457=CARTESIAN_POINT('Ctrl Pts',(25.9249204273251,62.3274386412541,209.17794904933));
#34458=CARTESIAN_POINT('Ctrl Pts',(25.7374038321486,62.2456729341707,209.165067733926));
#34459=CARTESIAN_POINT('Ctrl Pts',(25.3349647129544,62.155013595733,209.135723214818));
#34460=CARTESIAN_POINT('Ctrl Pts',(25.1233257200401,62.1495925231142,209.120291204918));
#34461=CARTESIAN_POINT('Ctrl Pts',(24.7065124792662,62.2212866237006,209.089898572778));
#34462=CARTESIAN_POINT('Ctrl Pts',(24.5057807588094,62.2990664084693,209.075843943418));
#34463=CARTESIAN_POINT('Ctrl Pts',(24.1539632003856,62.523932209519,209.048817506672));
#34464=CARTESIAN_POINT('Ctrl Pts',(24.0044362203571,62.6660067634534,209.034394322915));
#34465=CARTESIAN_POINT('Ctrl Pts',(23.7623348024638,63.0051207377533,209.004153446058));
#34466=CARTESIAN_POINT('Ctrl Pts',(23.6745745699214,63.2007885440448,208.988597885115));
#34467=CARTESIAN_POINT('Ctrl Pts',(23.5819964353755,63.6087447977246,208.959461147342));
#34468=CARTESIAN_POINT('Ctrl Pts',(23.5756230379735,63.8164391368395,208.947008816032));
#34469=CARTESIAN_POINT('Ctrl Pts',(23.6421067655174,64.2238069935368,208.918860592756));
#34470=CARTESIAN_POINT('Ctrl Pts',(23.7146720858874,64.4195012863386,208.903857340423));
#34471=CARTESIAN_POINT('Ctrl Pts',(23.9330904916492,64.7771245699987,208.873311086667));
#34472=CARTESIAN_POINT('Ctrl Pts',(24.0787340467908,64.9345223966226,208.858061856901));
#34473=CARTESIAN_POINT('Ctrl Pts',(24.4153626413047,65.1777316983955,208.830430834847));
#34474=CARTESIAN_POINT('Ctrl Pts',(24.6009079018128,65.2641884922171,208.817801760994));
#34475=CARTESIAN_POINT('Ctrl Pts',(25.0006024605227,65.3646894300876,208.788657366088));
#34476=CARTESIAN_POINT('Ctrl Pts',(25.2115046509785,65.3754215440957,208.773279081368));
#34477=CARTESIAN_POINT('Ctrl Pts',(25.6286330721951,65.3146747893705,208.742863467321));
#34478=CARTESIAN_POINT('Ctrl Pts',(25.8304808168065,65.2425542867193,208.728400814344));
#34479=CARTESIAN_POINT('Ctrl Pts',(26.1870350588532,65.0281984522,208.701865366071));
#34480=CARTESIAN_POINT('Ctrl Pts',(26.3400444864997,64.8907393312025,208.687606671987));
#34481=CARTESIAN_POINT('Ctrl Pts',(26.5909913895424,64.5595839971385,208.657545873196));
#34482=CARTESIAN_POINT('Ctrl Pts',(26.6841171531266,64.3671120691719,208.641996506253));
#34483=CARTESIAN_POINT('Ctrl Pts',(26.7709008326391,64.0310957604075,208.617613865684));
#34484=CARTESIAN_POINT('Ctrl Pts',(26.787903481163,63.8966856473105,208.608506289881));
#34485=CARTESIAN_POINT('Ctrl Pts',(26.787903481163,63.7619809500986,208.6));
#34486=CARTESIAN_POINT('Origin',(25.187903481163,63.761980950099,212.5));
#34487=CARTESIAN_POINT('',(26.787903481163,63.7619809500991,210.));
#34488=CARTESIAN_POINT('',(26.787903481163,63.7619809500987,209.912499998088));
#34489=CARTESIAN_POINT('',(26.787903481163,63.761980950099,212.5));
#34490=CARTESIAN_POINT('Ctrl Pts',(26.787903481163,63.761980950099,209.212499998088));
#34491=CARTESIAN_POINT('Ctrl Pts',(26.787903481163,63.9625096575748,209.22516292188));
#34492=CARTESIAN_POINT('Ctrl Pts',(26.7502103395188,64.1614336463926,209.239098740525));
#34493=CARTESIAN_POINT('Ctrl Pts',(26.5998957155974,64.5430426346555,209.268676685637));
#34494=CARTESIAN_POINT('Ctrl Pts',(26.4857614108062,64.7208094997246,209.284063398288));
#34495=CARTESIAN_POINT('Ctrl Pts',(26.1999165351698,65.0177711203375,209.313237265127));
#34496=CARTESIAN_POINT('Ctrl Pts',(26.0327231649848,65.1358206933445,209.325898562809));
#34497=CARTESIAN_POINT('Ctrl Pts',(25.6544426944634,65.3071185037487,209.353481513785));
#34498=CARTESIAN_POINT('Ctrl Pts',(25.4454898692234,65.3553169153305,209.368717657292));
#34499=CARTESIAN_POINT('Ctrl Pts',(25.0265418719815,65.3672025982405,209.399265948758));
#34500=CARTESIAN_POINT('Ctrl Pts',(24.8205842473973,65.3329288175183,209.414283692217));
#34501=CARTESIAN_POINT('Ctrl Pts',(24.4341113143586,65.1882168295297,209.442464010251));
#34502=CARTESIAN_POINT('Ctrl Pts',(24.2571614818908,65.0795829150789,209.454896452059));
#34503=CARTESIAN_POINT('Ctrl Pts',(23.9491198501745,64.7966550553686,209.483993376107));
#34504=CARTESIAN_POINT('Ctrl Pts',(23.8228479130678,64.6232243222286,209.499548789907));
#34505=CARTESIAN_POINT('Ctrl Pts',(23.6487613566745,64.2445008384581,209.529811207126));
#34506=CARTESIAN_POINT('Ctrl Pts',(23.5997439461575,64.0440727594058,209.544254869558));
#34507=CARTESIAN_POINT('Ctrl Pts',(23.5794462759211,63.6272334648883,209.57131732554));
#34508=CARTESIAN_POINT('Ctrl Pts',(23.6116007681108,63.4146720776778,209.585295713189));
#34509=CARTESIAN_POINT('Ctrl Pts',(23.7562325183374,63.017454396937,209.615652123004));
#34510=CARTESIAN_POINT('Ctrl Pts',(23.8660690515765,62.8363682030017,209.631091754003));
#34511=CARTESIAN_POINT('Ctrl Pts',(24.1446650021707,62.532024541803,209.660467495895));
#34512=CARTESIAN_POINT('Ctrl Pts',(24.3087540644221,62.409872210698,209.673395353117));
#34513=CARTESIAN_POINT('Ctrl Pts',(24.6824419683471,62.229138169489,209.700643429445));
#34514=CARTESIAN_POINT('Ctrl Pts',(24.8900793264089,62.1756781715759,209.715783653471));
#34515=CARTESIAN_POINT('Ctrl Pts',(25.3090639956147,62.1531602042708,209.746334618934));
#34516=CARTESIAN_POINT('Ctrl Pts',(25.5163214487618,62.1823770473555,209.761447141559));
#34517=CARTESIAN_POINT('Ctrl Pts',(25.9057883099507,62.3174722790651,209.789845766854));
#34518=CARTESIAN_POINT('Ctrl Pts',(26.084589526411,62.4211161840766,209.802185836687));
#34519=CARTESIAN_POINT('Ctrl Pts',(26.3996213423553,62.6956275303874,209.831006127859));
#34520=CARTESIAN_POINT('Ctrl Pts',(26.5306397132082,62.8662097222909,209.846554709935));
#34521=CARTESIAN_POINT('Ctrl Pts',(26.7146489611726,63.2413697020022,209.876953864917));
#34522=CARTESIAN_POINT('Ctrl Pts',(26.7687292090268,63.4410177911385,209.891532855402));
#34523=CARTESIAN_POINT('Ctrl Pts',(26.7864907564276,63.6843022602055,209.907543263004));
#34524=CARTESIAN_POINT('Ctrl Pts',(26.787903481163,63.7231612765527,209.910048625544));
#34525=CARTESIAN_POINT('Ctrl Pts',(26.787903481163,63.7619809500983,209.912499998088));
#34526=CARTESIAN_POINT('Ctrl Pts',(26.787903481163,63.7619809500992,210.));
#34527=CARTESIAN_POINT('Ctrl Pts',(26.787903481163,63.635661259033,209.992023203852));
#34528=CARTESIAN_POINT('Ctrl Pts',(26.7729513315449,63.5095551023203,209.983514761449));
#34529=CARTESIAN_POINT('Ctrl Pts',(26.6942281251588,63.1837109674741,209.960068341537));
#34530=CARTESIAN_POINT('Ctrl Pts',(26.606212810655,62.9926997944486,209.944797536345));
#34531=CARTESIAN_POINT('Ctrl Pts',(26.3596846196389,62.6520478145269,209.914298145222));
#34532=CARTESIAN_POINT('Ctrl Pts',(26.2022910462423,62.5065565628155,209.899372402024));
#34533=CARTESIAN_POINT('Ctrl Pts',(25.8477593079741,62.2903196808869,209.872791907078));
#34534=CARTESIAN_POINT('Ctrl Pts',(25.6558592320014,62.2185120888091,209.859121773499));
#34535=CARTESIAN_POINT('Ctrl Pts',(25.2477105958396,62.1492614922979,209.829360935445));
#34536=CARTESIAN_POINT('Ctrl Pts',(25.0349300186893,62.1554178305597,209.813845685028));
#34537=CARTESIAN_POINT('Ctrl Pts',(24.6251458927997,62.2496130926411,209.783965592515));
#34538=CARTESIAN_POINT('Ctrl Pts',(24.4321175076648,62.3362485402014,209.770810338485));
#34539=CARTESIAN_POINT('Ctrl Pts',(24.093785600076,62.5766076676862,209.743297198385));
#34540=CARTESIAN_POINT('Ctrl Pts',(23.9508208408974,62.7267062961762,209.728606560525));
#34541=CARTESIAN_POINT('Ctrl Pts',(23.725129139662,63.0794554025556,209.698102927553));
#34542=CARTESIAN_POINT('Ctrl Pts',(23.6472140844721,63.2804695810034,209.682568694339));
#34543=CARTESIAN_POINT('Ctrl Pts',(23.5764456589093,63.6920806143508,209.653996311329));
#34544=CARTESIAN_POINT('Ctrl Pts',(23.5806743473847,63.8979958834204,209.64167453391));
#34545=CARTESIAN_POINT('Ctrl Pts',(23.667100980843,64.3008226245383,209.613085986462));
#34546=CARTESIAN_POINT('Ctrl Pts',(23.7498671504022,64.4935701194035,209.59789691164));
#34547=CARTESIAN_POINT('Ctrl Pts',(23.986935465546,64.8402746188052,209.567360209227));
#34548=CARTESIAN_POINT('Ctrl Pts',(24.1404252825187,64.9899373162383,209.552313373339));
#34549=CARTESIAN_POINT('Ctrl Pts',(24.4889292317419,65.2154412930024,209.525367445943));
#34550=CARTESIAN_POINT('Ctrl Pts',(24.6785881192932,65.2922634592259,209.51213757847));
#34551=CARTESIAN_POINT('Ctrl Pts',(25.0838844226146,65.3723790789397,209.482584723019));
#34552=CARTESIAN_POINT('Ctrl Pts',(25.2961645249118,65.3720995389519,209.46710596556));
#34553=CARTESIAN_POINT('Ctrl Pts',(25.7095716663637,65.2892482902382,209.436961694829));
#34554=CARTESIAN_POINT('Ctrl Pts',(25.9064733534398,65.2070749914989,209.423389817729));
#34555=CARTESIAN_POINT('Ctrl Pts',(26.2516850693628,64.9745670252063,209.396121633943));
#34556=CARTESIAN_POINT('Ctrl Pts',(26.3980477416357,64.8285207487543,209.381563010488));
#34557=CARTESIAN_POINT('Ctrl Pts',(26.6321970240694,64.4826245370138,209.351183772638));
#34558=CARTESIAN_POINT('Ctrl Pts',(26.7151695069104,64.2842757963881,209.33563347027));
#34559=CARTESIAN_POINT('Ctrl Pts',(26.777564314995,63.9720117850579,209.313639909918));
#34560=CARTESIAN_POINT('Ctrl Pts',(26.787903481163,63.8670158574599,209.306632711317));
#34561=CARTESIAN_POINT('Ctrl Pts',(26.787903481163,63.761980950099,209.3));
#34562=CARTESIAN_POINT('Origin',(25.187903481163,63.761980950099,212.5));
#34563=CARTESIAN_POINT('',(26.787903481163,63.7619809500994,210.7));
#34564=CARTESIAN_POINT('',(26.787903481163,63.7619809500987,210.612499998088));
#34565=CARTESIAN_POINT('',(26.787903481163,63.761980950099,212.5));
#34566=CARTESIAN_POINT('Ctrl Pts',(26.787903481163,63.7619809500983,209.912499998088));
#34567=CARTESIAN_POINT('Ctrl Pts',(26.7879034811631,63.9335970442676,209.923337157262));
#34568=CARTESIAN_POINT('Ctrl Pts',(26.7603050063469,64.1043181033942,209.93512399144));
#34569=CARTESIAN_POINT('Ctrl Pts',(26.6394171169629,64.4672093546526,209.962447105082));
#34570=CARTESIAN_POINT('Ctrl Pts',(26.534242295437,64.6517055105942,209.97793210905));
#34571=CARTESIAN_POINT('Ctrl Pts',(26.2634103644491,64.9638391022234,210.007516703806));
#34572=CARTESIAN_POINT('Ctrl Pts',(26.1025412418608,65.0903474203494,210.020807661371));
#34573=CARTESIAN_POINT('Ctrl Pts',(25.7337514358277,65.2809066557851,210.047698584727));
#34574=CARTESIAN_POINT('Ctrl Pts',(25.5276371511831,65.339833831516,210.062727751316));
#34575=CARTESIAN_POINT('Ctrl Pts',(25.1089062067284,65.3734909493857,210.093260216016));
#34576=CARTESIAN_POINT('Ctrl Pts',(24.9004199290461,65.3496134728875,210.10846234043));
#34577=CARTESIAN_POINT('Ctrl Pts',(24.5078841996179,65.2245866177153,210.137084737367));
#34578=CARTESIAN_POINT('Ctrl Pts',(24.3271448115197,65.1260675356885,210.149409580288));
#34579=CARTESIAN_POINT('Ctrl Pts',(24.0049872090873,64.8603085050649,210.177936977279));
#34580=CARTESIAN_POINT('Ctrl Pts',(23.869130810807,64.6928005525691,210.193467814668));
#34581=CARTESIAN_POINT('Ctrl Pts',(23.6749465000499,64.32158831826,210.223988644495));
#34582=CARTESIAN_POINT('Ctrl Pts',(23.615647832192,64.1228792481685,210.238698592997));
#34583=CARTESIAN_POINT('Ctrl Pts',(23.5751036531259,63.7100102747399,210.266248486358));
#34584=CARTESIAN_POINT('Ctrl Pts',(23.5957181798156,63.4996920144276,210.279347848247));
#34585=CARTESIAN_POINT('Ctrl Pts',(23.7172785329909,63.0973418160769,210.309187219987));
#34586=CARTESIAN_POINT('Ctrl Pts',(23.8175972209408,62.9094916850686,210.324706973182));
#34587=CARTESIAN_POINT('Ctrl Pts',(24.0804303953468,62.5894595343949,210.354498722328));
#34588=CARTESIAN_POINT('Ctrl Pts',(24.2380864280138,62.4584995642421,210.368242504629));
#34589=CARTESIAN_POINT('Ctrl Pts',(24.6018598470313,62.2581116168253,210.394767649766));
#34590=CARTESIAN_POINT('Ctrl Pts',(24.8062940313073,62.1937354835571,210.409674309036));
#34591=CARTESIAN_POINT('Ctrl Pts',(25.2244685855717,62.1488809917243,210.440166203618));
#34592=CARTESIAN_POINT('Ctrl Pts',(25.4340527763025,62.1673481920154,210.455448384192));
#34593=CARTESIAN_POINT('Ctrl Pts',(25.8296006406912,62.2822433160495,210.48429041597));
#34594=CARTESIAN_POINT('Ctrl Pts',(26.0123084898772,62.3757104938337,210.496683326307));
#34595=CARTESIAN_POINT('Ctrl Pts',(26.3414378648629,62.6327255493329,210.524912740713));
#34596=CARTESIAN_POINT('Ctrl Pts',(26.4820226865197,62.797054890118,210.540415246564));
#34597=CARTESIAN_POINT('Ctrl Pts',(26.6862135177991,63.1640874037339,210.571036957764));
#34598=CARTESIAN_POINT('Ctrl Pts',(26.7506712760385,63.3617320086207,210.585867779588));
#34599=CARTESIAN_POINT('Ctrl Pts',(26.7839044580146,63.6312850583613,210.604101057276));
#34600=CARTESIAN_POINT('Ctrl Pts',(26.787903481163,63.6966644992972,210.608375415382));
#34601=CARTESIAN_POINT('Ctrl Pts',(26.787903481163,63.7619809500984,210.612499998088));
#34602=CARTESIAN_POINT('Ctrl Pts',(26.787903481163,63.7619809500997,210.7));
#34603=CARTESIAN_POINT('Ctrl Pts',(26.787903481163,63.6098599431785,210.690393910468));
#34604=CARTESIAN_POINT('Ctrl Pts',(26.7662204259159,63.4583029385245,210.680032908317));
#34605=CARTESIAN_POINT('Ctrl Pts',(26.664368656578,63.1109236989383,210.654383367523));
#34606=CARTESIAN_POINT('Ctrl Pts',(26.5666136050719,62.9235442379033,210.638986801959));
#34607=CARTESIAN_POINT('Ctrl Pts',(26.3012618617114,62.593025913473,210.608441052382));
#34608=CARTESIAN_POINT('Ctrl Pts',(26.134749550499,62.4545324444443,210.594040859222));
#34609=CARTESIAN_POINT('Ctrl Pts',(25.7662324440654,62.256255964826,210.567169820212));
#34610=CARTESIAN_POINT('Ctrl Pts',(25.569655691065,62.1948521984884,210.552836098639));
#34611=CARTESIAN_POINT('Ctrl Pts',(25.1562464175635,62.1483084122457,210.522691672446));
#34612=CARTESIAN_POINT('Ctrl Pts',(24.9429378720832,62.1666916011874,210.507137924338));
#34613=CARTESIAN_POINT('Ctrl Pts',(24.5410407365537,62.2840519395233,210.477832924872));
#34614=CARTESIAN_POINT('Ctrl Pts',(24.355834723001,62.3798235040937,210.46527753717));
#34615=CARTESIAN_POINT('Ctrl Pts',(24.0320922328871,62.6364834962525,210.437266941037));
#34616=CARTESIAN_POINT('Ctrl Pts',(23.8966578737162,62.7948720268811,210.422327360876));
#34617=CARTESIAN_POINT('Ctrl Pts',(23.6905773432696,63.1594076509547,210.39179442719));
#34618=CARTESIAN_POINT('Ctrl Pts',(23.6238959356232,63.3632377791808,210.376491933331));
#34619=CARTESIAN_POINT('Ctrl Pts',(23.5751260975114,63.7758548244946,210.348658054828));
#34620=CARTESIAN_POINT('Ctrl Pts',(23.58989155688,63.9801940249824,210.336147867406));
#34621=CARTESIAN_POINT('Ctrl Pts',(23.6965976329302,64.3781231113291,210.307129240844));
#34622=CARTESIAN_POINT('Ctrl Pts',(23.7896725171562,64.5673152440865,210.291788840355));
#34623=CARTESIAN_POINT('Ctrl Pts',(24.0453559413064,64.9020147242601,210.261331551274));
#34624=CARTESIAN_POINT('Ctrl Pts',(24.2064884219356,65.0433065986533,210.246561514735));
#34625=CARTESIAN_POINT('Ctrl Pts',(24.5667970441878,65.2504923103573,210.220289011029));
#34626=CARTESIAN_POINT('Ctrl Pts',(24.7609675184813,65.3173319874089,210.206130747279));
#34627=CARTESIAN_POINT('Ctrl Pts',(25.1716461741282,65.3758005468082,210.176185428638));
#34628=CARTESIAN_POINT('Ctrl Pts',(25.3847635454736,65.3638342065162,210.160645620311));
#34629=CARTESIAN_POINT('Ctrl Pts',(25.7908578316024,65.2585640109584,210.131034578614));
#34630=CARTESIAN_POINT('Ctrl Pts',(25.9801301897951,65.1675682217721,210.11820965116));
#34631=CARTESIAN_POINT('Ctrl Pts',(26.311580130965,64.9194619400752,210.090458201226));
#34632=CARTESIAN_POINT('Ctrl Pts',(26.4510458637665,64.765399864603,210.075644849532));
#34633=CARTESIAN_POINT('Ctrl Pts',(26.668108721095,64.4060176157923,210.045036942234));
#34634=CARTESIAN_POINT('Ctrl Pts',(26.7408983027634,64.2024689537162,210.029529528466));
#34635=CARTESIAN_POINT('Ctrl Pts',(26.7824404364531,63.9147221412979,210.009844426239));
#34636=CARTESIAN_POINT('Ctrl Pts',(26.787903481163,63.8383252279674,210.004820964463));
#34637=CARTESIAN_POINT('Ctrl Pts',(26.787903481163,63.7619809500992,210.));
#34638=CARTESIAN_POINT('Origin',(25.187903481163,63.761980950099,212.5));
#34639=CARTESIAN_POINT('',(26.787903481163,63.7619809500991,211.4));
#34640=CARTESIAN_POINT('',(26.787903481163,63.761980950099,211.312499998088));
#34641=CARTESIAN_POINT('',(26.787903481163,63.761980950099,212.5));
#34642=CARTESIAN_POINT('Ctrl Pts',(26.787903481163,63.7619809500984,210.612499998088));
#34643=CARTESIAN_POINT('Ctrl Pts',(26.7879034811631,63.9037107253896,210.621449905392));
#34644=CARTESIAN_POINT('Ctrl Pts',(26.7690814709595,64.0450567131394,210.631061796522));
#34645=CARTESIAN_POINT('Ctrl Pts',(26.676120457749,64.3864277595664,210.656007791673));
#34646=CARTESIAN_POINT('Ctrl Pts',(26.5806505336575,64.5774371296308,210.671550265654));
#34647=CARTESIAN_POINT('Ctrl Pts',(26.3258621156874,64.9049914141014,210.701523721729));
#34648=CARTESIAN_POINT('Ctrl Pts',(26.1713533227639,65.0403771596247,210.71570615131));
#34649=CARTESIAN_POINT('Ctrl Pts',(25.8124811708408,65.2502286765258,210.74204166948));
#34650=CARTESIAN_POINT('Ctrl Pts',(25.6098048312725,65.3198939590718,210.756736357976));
#34651=CARTESIAN_POINT('Ctrl Pts',(25.1922317328634,65.3755565745708,210.787184396402));
#34652=CARTESIAN_POINT('Ctrl Pts',(24.9817212059254,65.3623385461095,210.802534122324));
#34653=CARTESIAN_POINT('Ctrl Pts',(24.5833395517246,65.2572210268484,210.83158278461));
#34654=CARTESIAN_POINT('Ctrl Pts',(24.3987100063986,65.1685359919833,210.844118647828));
#34655=CARTESIAN_POINT('Ctrl Pts',(24.0648789193331,64.9212610365502,210.871904414043));
#34656=CARTESIAN_POINT('Ctrl Pts',(23.9211076293836,64.7621342296066,210.887194565245));
#34657=CARTESIAN_POINT('Ctrl Pts',(23.7070740647399,64.4021292053075,210.917731356412));
#34658=CARTESIAN_POINT('Ctrl Pts',(23.6368802079579,64.2058290103964,210.93268641045));
#34659=CARTESIAN_POINT('Ctrl Pts',(23.5750272679402,63.7974449517029,210.960729973735));
#34660=CARTESIAN_POINT('Ctrl Pts',(23.5839027566284,63.5893072917234,210.973258080246));
#34661=CARTESIAN_POINT('Ctrl Pts',(23.6816051332063,63.1822774641359,211.002523137679));
#34662=CARTESIAN_POINT('Ctrl Pts',(23.7716313957965,62.9879341047716,211.018077678543));
#34663=CARTESIAN_POINT('Ctrl Pts',(24.0174773001968,62.6521340551642,211.048245806462));
#34664=CARTESIAN_POINT('Ctrl Pts',(24.168483443106,62.5119870400657,211.062601198416));
#34665=CARTESIAN_POINT('Ctrl Pts',(24.5234622974082,62.2908155773961,211.089509601821));
#34666=CARTESIAN_POINT('Ctrl Pts',(24.7260650487856,62.2151797158321,211.103824279061));
#34667=CARTESIAN_POINT('Ctrl Pts',(25.1444797102404,62.1489193406298,211.134333681458));
#34668=CARTESIAN_POINT('Ctrl Pts',(25.3557546484568,62.1570865885378,211.149739145703));
#34669=CARTESIAN_POINT('Ctrl Pts',(25.7567847791617,62.2528316013046,211.178980926067));
#34670=CARTESIAN_POINT('Ctrl Pts',(25.9432793469075,62.3370116972185,211.191722899357));
#34671=CARTESIAN_POINT('Ctrl Pts',(26.2827471489827,62.5760539273622,211.219194293258));
#34672=CARTESIAN_POINT('Ctrl Pts',(26.4302825723362,62.7316607245787,211.234399398023));
#34673=CARTESIAN_POINT('Ctrl Pts',(26.6531563261176,63.0867932265012,211.26495079924));
#34674=CARTESIAN_POINT('Ctrl Pts',(26.7281414813671,63.2818387401592,211.280001305818));
#34675=CARTESIAN_POINT('Ctrl Pts',(26.7799044875922,63.5771945052862,211.300539531777));
#34676=CARTESIAN_POINT('Ctrl Pts',(26.787903481163,63.6695974072158,211.306666191159));
#34677=CARTESIAN_POINT('Ctrl Pts',(26.787903481163,63.761980950099,211.312499998088));
#34678=CARTESIAN_POINT('Ctrl Pts',(26.787903481163,63.7619809500992,211.4));
#34679=CARTESIAN_POINT('Ctrl Pts',(26.787903481163,63.5818177827691,211.388623112936));
#34680=CARTESIAN_POINT('Ctrl Pts',(26.7574834653626,63.4027735141896,211.376207818663));
#34681=CARTESIAN_POINT('Ctrl Pts',(26.6280540227834,63.0338003226158,211.348189233772));
#34682=CARTESIAN_POINT('Ctrl Pts',(26.5199058336431,62.8509089809943,211.332697166086));
#34683=CARTESIAN_POINT('Ctrl Pts',(26.2387935136483,62.5372102260688,211.302638929041));
#34684=CARTESIAN_POINT('Ctrl Pts',(26.0685425028871,62.409623601325,211.289213262001));
#34685=CARTESIAN_POINT('Ctrl Pts',(25.6934670952748,62.2301618676489,211.261864013529));
#34686=CARTESIAN_POINT('Ctrl Pts',(25.4931983745446,62.1780553272494,211.247261085976));
#34687=CARTESIAN_POINT('Ctrl Pts',(25.0759790833614,62.1517443047337,211.216838845994));
#34688=CARTESIAN_POINT('Ctrl Pts',(24.8627737506939,62.1809358106765,211.20129262382));
#34689=CARTESIAN_POINT('Ctrl Pts',(24.4682306869984,62.318384231228,211.172523858759));
#34690=CARTESIAN_POINT('Ctrl Pts',(24.2896915048165,62.4221615228617,211.160192517772));
#34691=CARTESIAN_POINT('Ctrl Pts',(23.9792294077263,62.6932657854073,211.131753980388));
#34692=CARTESIAN_POINT('Ctrl Pts',(23.850999101966,62.8588144578357,211.116624901623));
#34693=CARTESIAN_POINT('Ctrl Pts',(23.6627242118601,63.2338890512605,211.086075620385));
#34694=CARTESIAN_POINT('Ctrl Pts',(23.6061720701984,63.4406992708552,211.070954236808));
#34695=CARTESIAN_POINT('Ctrl Pts',(23.5777851557484,63.8548157504408,211.043768799926));
#34696=CARTESIAN_POINT('Ctrl Pts',(23.6024758470122,64.0578851219841,211.030783052187));
#34697=CARTESIAN_POINT('Ctrl Pts',(23.7286150058584,64.4508373542569,211.001370204632));
#34698=CARTESIAN_POINT('Ctrl Pts',(23.8314542072517,64.6361025043355,210.985921793281));
#34699=CARTESIAN_POINT('Ctrl Pts',(24.1045537716373,64.9584604062835,210.955608882856));
#34700=CARTESIAN_POINT('Ctrl Pts',(24.2728951014121,65.0916092228732,210.941719361024));
#34701=CARTESIAN_POINT('Ctrl Pts',(24.6446256883595,65.2807669139696,210.914614005725));
#34702=CARTESIAN_POINT('Ctrl Pts',(24.8430428829701,65.3377000506952,210.900146085285));
#34703=CARTESIAN_POINT('Ctrl Pts',(25.2584164857913,65.3744897977321,210.869858426746));
#34704=CARTESIAN_POINT('Ctrl Pts',(25.4717415535027,65.3508837642616,210.854303473892));
#34705=CARTESIAN_POINT('Ctrl Pts',(25.8701292242356,65.2237778267173,210.825254372901));
#34706=CARTESIAN_POINT('Ctrl Pts',(26.0520865945744,65.1241359209362,210.812843591287));
#34707=CARTESIAN_POINT('Ctrl Pts',(26.3694620049696,64.8605053532319,210.784624952554));
#34708=CARTESIAN_POINT('Ctrl Pts',(26.5014814935139,64.6986363516567,210.7695900892));
#34709=CARTESIAN_POINT('Ctrl Pts',(26.6990750005974,64.3289275833056,210.739039906152));
#34710=CARTESIAN_POINT('Ctrl Pts',(26.760906433387,64.123600783922,210.723819722973));
#34711=CARTESIAN_POINT('Ctrl Pts',(26.7855541995538,63.8621531395226,210.706411292825));
#34712=CARTESIAN_POINT('Ctrl Pts',(26.787903481163,63.8120419129629,210.703161233948));
#34713=CARTESIAN_POINT('Ctrl Pts',(26.787903481163,63.7619809500997,210.7));
#34714=CARTESIAN_POINT('Origin',(25.187903481163,63.761980950099,212.5));
#34715=CARTESIAN_POINT('',(26.787903481163,63.761980950099,212.1));
#34716=CARTESIAN_POINT('',(26.787903481163,63.7619809500991,212.012499998088));
#34717=CARTESIAN_POINT('',(26.787903481163,63.761980950099,212.5));
#34718=CARTESIAN_POINT('',(26.3295442486903,64.882987800176,212.1));
#34719=CARTESIAN_POINT('Origin',(25.187903481163,63.761980950099,212.1));
#34720=CARTESIAN_POINT('Ctrl Pts',(26.787903481163,63.7619809500991,212.012499998088));
#34721=CARTESIAN_POINT('Ctrl Pts',(26.787903481163,63.8455254713351,212.017775641257));
#34722=CARTESIAN_POINT('Ctrl Pts',(26.7813616254594,63.929111069376,212.023292383486));
#34723=CARTESIAN_POINT('Ctrl Pts',(26.7425017960021,64.174747183526,212.040220500233));
#34724=CARTESIAN_POINT('Ctrl Pts',(26.6917702440339,64.3325238033038,212.05203331646));
#34725=CARTESIAN_POINT('Ctrl Pts',(26.5433031849841,64.6283088414431,212.076124318609));
#34726=CARTESIAN_POINT('Ctrl Pts',(26.4460274836205,64.7643605056857,212.088262176286));
#34727=CARTESIAN_POINT('Ctrl Pts',(26.3295442486903,64.882987800176,212.1));
#34728=CARTESIAN_POINT('Origin',(25.1879034811629,63.761980950099,212.406249999044));
#34729=CARTESIAN_POINT('',(23.966789593663,63.761980950099,203.043749999044));
#34730=CARTESIAN_POINT('',(23.966789593663,63.761980950099,202.868749999044));
#34731=CARTESIAN_POINT('',(23.9667895936629,63.761980950099,212.406249999044));
#34732=CARTESIAN_POINT('',(26.409017368663,63.761980950099,202.518749999044));
#34733=CARTESIAN_POINT('Ctrl Pts',(23.966789593663,63.761980950099,202.868749999044));
#34734=CARTESIAN_POINT('Ctrl Pts',(23.966789593663,64.4669913817583,202.810416665711));
#34735=CARTESIAN_POINT('Ctrl Pts',(24.577346537413,64.819496597588,202.752083332377));
#34736=CARTESIAN_POINT('Ctrl Pts',(25.187903481163,65.1720018134176,202.693749999044));
#34737=CARTESIAN_POINT('Ctrl Pts',(25.798460424913,64.819496597588,202.635416665711));
#34738=CARTESIAN_POINT('Ctrl Pts',(26.409017368663,64.4669913817583,202.577083332377));
#34739=CARTESIAN_POINT('Ctrl Pts',(26.409017368663,63.761980950099,202.518749999044));
#34740=CARTESIAN_POINT('',(26.409017368663,63.761980950099,202.693749999044));
#34741=CARTESIAN_POINT('',(26.409017368663,63.761980950099,202.606249999044));
#34742=CARTESIAN_POINT('Ctrl Pts',(23.966789593663,63.761980950099,203.043749999044));
#34743=CARTESIAN_POINT('Ctrl Pts',(23.966789593663,64.4669913817583,202.985416665711));
#34744=CARTESIAN_POINT('Ctrl Pts',(24.577346537413,64.819496597588,202.927083332377));
#34745=CARTESIAN_POINT('Ctrl Pts',(25.187903481163,65.1720018134176,202.868749999044));
#34746=CARTESIAN_POINT('Ctrl Pts',(25.798460424913,64.819496597588,202.810416665711));
#34747=CARTESIAN_POINT('Ctrl Pts',(26.409017368663,64.4669913817583,202.752083332377));
#34748=CARTESIAN_POINT('Ctrl Pts',(26.409017368663,63.761980950099,202.693749999044));
#34749=CARTESIAN_POINT('Origin',(25.1879034811629,63.761980950099,212.406249999044));
#34750=CARTESIAN_POINT('',(23.966789593663,63.761980950099,203.743749999044));
#34751=CARTESIAN_POINT('',(23.966789593663,63.761980950099,203.568749999044));
#34752=CARTESIAN_POINT('',(23.9667895936629,63.761980950099,212.406249999044));
#34753=CARTESIAN_POINT('Ctrl Pts',(23.966789593663,63.761980950099,203.568749999044));
#34754=CARTESIAN_POINT('Ctrl Pts',(23.966789593663,64.4669913817583,203.510416665711));
#34755=CARTESIAN_POINT('Ctrl Pts',(24.577346537413,64.819496597588,203.452083332377));
#34756=CARTESIAN_POINT('Ctrl Pts',(25.187903481163,65.1720018134176,203.393749999044));
#34757=CARTESIAN_POINT('Ctrl Pts',(25.798460424913,64.819496597588,203.335416665711));
#34758=CARTESIAN_POINT('Ctrl Pts',(26.409017368663,64.4669913817583,203.277083332377));
#34759=CARTESIAN_POINT('Ctrl Pts',(26.409017368663,63.761980950099,203.218749999044));
#34760=CARTESIAN_POINT('Ctrl Pts',(26.409017368663,63.0569705184397,203.160416665711));
#34761=CARTESIAN_POINT('Ctrl Pts',(25.798460424913,62.70446530261,203.102083332377));
#34762=CARTESIAN_POINT('Ctrl Pts',(25.187903481163,62.3519600867804,203.043749999044));
#34763=CARTESIAN_POINT('Ctrl Pts',(24.577346537413,62.70446530261,202.985416665711));
#34764=CARTESIAN_POINT('Ctrl Pts',(23.966789593663,63.0569705184397,202.927083332377));
#34765=CARTESIAN_POINT('Ctrl Pts',(23.966789593663,63.761980950099,202.868749999044));
#34766=CARTESIAN_POINT('Ctrl Pts',(23.966789593663,63.761980950099,203.743749999044));
#34767=CARTESIAN_POINT('Ctrl Pts',(23.966789593663,64.4669913817583,203.685416665711));
#34768=CARTESIAN_POINT('Ctrl Pts',(24.577346537413,64.819496597588,203.627083332377));
#34769=CARTESIAN_POINT('Ctrl Pts',(25.187903481163,65.1720018134176,203.568749999044));
#34770=CARTESIAN_POINT('Ctrl Pts',(25.798460424913,64.819496597588,203.510416665711));
#34771=CARTESIAN_POINT('Ctrl Pts',(26.409017368663,64.4669913817583,203.452083332377));
#34772=CARTESIAN_POINT('Ctrl Pts',(26.409017368663,63.761980950099,203.393749999044));
#34773=CARTESIAN_POINT('Ctrl Pts',(26.409017368663,63.0569705184397,203.335416665711));
#34774=CARTESIAN_POINT('Ctrl Pts',(25.798460424913,62.70446530261,203.277083332377));
#34775=CARTESIAN_POINT('Ctrl Pts',(25.187903481163,62.3519600867804,203.218749999044));
#34776=CARTESIAN_POINT('Ctrl Pts',(24.577346537413,62.70446530261,203.160416665711));
#34777=CARTESIAN_POINT('Ctrl Pts',(23.966789593663,63.0569705184397,203.102083332377));
#34778=CARTESIAN_POINT('Ctrl Pts',(23.966789593663,63.761980950099,203.043749999044));
#34779=CARTESIAN_POINT('Origin',(25.1879034811629,63.761980950099,212.406249999044));
#34780=CARTESIAN_POINT('',(23.966789593663,63.761980950099,204.443749999044));
#34781=CARTESIAN_POINT('',(23.966789593663,63.761980950099,204.268749999044));
#34782=CARTESIAN_POINT('',(23.9667895936629,63.761980950099,212.406249999044));
#34783=CARTESIAN_POINT('Ctrl Pts',(23.966789593663,63.761980950099,204.268749999044));
#34784=CARTESIAN_POINT('Ctrl Pts',(23.966789593663,64.4669913817583,204.210416665711));
#34785=CARTESIAN_POINT('Ctrl Pts',(24.577346537413,64.819496597588,204.152083332377));
#34786=CARTESIAN_POINT('Ctrl Pts',(25.187903481163,65.1720018134176,204.093749999044));
#34787=CARTESIAN_POINT('Ctrl Pts',(25.798460424913,64.819496597588,204.035416665711));
#34788=CARTESIAN_POINT('Ctrl Pts',(26.409017368663,64.4669913817583,203.977083332377));
#34789=CARTESIAN_POINT('Ctrl Pts',(26.409017368663,63.761980950099,203.918749999044));
#34790=CARTESIAN_POINT('Ctrl Pts',(26.409017368663,63.0569705184397,203.860416665711));
#34791=CARTESIAN_POINT('Ctrl Pts',(25.798460424913,62.70446530261,203.802083332377));
#34792=CARTESIAN_POINT('Ctrl Pts',(25.187903481163,62.3519600867804,203.743749999044));
#34793=CARTESIAN_POINT('Ctrl Pts',(24.577346537413,62.70446530261,203.685416665711));
#34794=CARTESIAN_POINT('Ctrl Pts',(23.966789593663,63.0569705184397,203.627083332377));
#34795=CARTESIAN_POINT('Ctrl Pts',(23.966789593663,63.761980950099,203.568749999044));
#34796=CARTESIAN_POINT('Ctrl Pts',(23.966789593663,63.761980950099,204.443749999044));
#34797=CARTESIAN_POINT('Ctrl Pts',(23.966789593663,64.4669913817583,204.385416665711));
#34798=CARTESIAN_POINT('Ctrl Pts',(24.577346537413,64.819496597588,204.327083332377));
#34799=CARTESIAN_POINT('Ctrl Pts',(25.187903481163,65.1720018134176,204.268749999044));
#34800=CARTESIAN_POINT('Ctrl Pts',(25.798460424913,64.819496597588,204.210416665711));
#34801=CARTESIAN_POINT('Ctrl Pts',(26.409017368663,64.4669913817583,204.152083332377));
#34802=CARTESIAN_POINT('Ctrl Pts',(26.409017368663,63.761980950099,204.093749999044));
#34803=CARTESIAN_POINT('Ctrl Pts',(26.409017368663,63.0569705184397,204.035416665711));
#34804=CARTESIAN_POINT('Ctrl Pts',(25.798460424913,62.70446530261,203.977083332377));
#34805=CARTESIAN_POINT('Ctrl Pts',(25.187903481163,62.3519600867804,203.918749999044));
#34806=CARTESIAN_POINT('Ctrl Pts',(24.577346537413,62.70446530261,203.860416665711));
#34807=CARTESIAN_POINT('Ctrl Pts',(23.966789593663,63.0569705184397,203.802083332377));
#34808=CARTESIAN_POINT('Ctrl Pts',(23.966789593663,63.761980950099,203.743749999044));
#34809=CARTESIAN_POINT('Origin',(25.1879034811629,63.761980950099,212.406249999044));
#34810=CARTESIAN_POINT('',(23.966789593663,63.761980950099,205.143749999044));
#34811=CARTESIAN_POINT('',(23.966789593663,63.761980950099,204.968749999044));
#34812=CARTESIAN_POINT('',(23.9667895936629,63.761980950099,212.406249999044));
#34813=CARTESIAN_POINT('Ctrl Pts',(23.966789593663,63.761980950099,204.968749999044));
#34814=CARTESIAN_POINT('Ctrl Pts',(23.966789593663,64.4669913817583,204.910416665711));
#34815=CARTESIAN_POINT('Ctrl Pts',(24.577346537413,64.819496597588,204.852083332377));
#34816=CARTESIAN_POINT('Ctrl Pts',(25.187903481163,65.1720018134176,204.793749999044));
#34817=CARTESIAN_POINT('Ctrl Pts',(25.798460424913,64.819496597588,204.735416665711));
#34818=CARTESIAN_POINT('Ctrl Pts',(26.409017368663,64.4669913817583,204.677083332377));
#34819=CARTESIAN_POINT('Ctrl Pts',(26.409017368663,63.761980950099,204.618749999044));
#34820=CARTESIAN_POINT('Ctrl Pts',(26.409017368663,63.0569705184397,204.560416665711));
#34821=CARTESIAN_POINT('Ctrl Pts',(25.798460424913,62.70446530261,204.502083332377));
#34822=CARTESIAN_POINT('Ctrl Pts',(25.187903481163,62.3519600867804,204.443749999044));
#34823=CARTESIAN_POINT('Ctrl Pts',(24.577346537413,62.70446530261,204.385416665711));
#34824=CARTESIAN_POINT('Ctrl Pts',(23.966789593663,63.0569705184397,204.327083332377));
#34825=CARTESIAN_POINT('Ctrl Pts',(23.966789593663,63.761980950099,204.268749999044));
#34826=CARTESIAN_POINT('Ctrl Pts',(23.966789593663,63.761980950099,205.143749999044));
#34827=CARTESIAN_POINT('Ctrl Pts',(23.966789593663,64.4669913817583,205.085416665711));
#34828=CARTESIAN_POINT('Ctrl Pts',(24.577346537413,64.819496597588,205.027083332377));
#34829=CARTESIAN_POINT('Ctrl Pts',(25.187903481163,65.1720018134176,204.968749999044));
#34830=CARTESIAN_POINT('Ctrl Pts',(25.798460424913,64.819496597588,204.910416665711));
#34831=CARTESIAN_POINT('Ctrl Pts',(26.409017368663,64.4669913817583,204.852083332377));
#34832=CARTESIAN_POINT('Ctrl Pts',(26.409017368663,63.761980950099,204.793749999044));
#34833=CARTESIAN_POINT('Ctrl Pts',(26.409017368663,63.0569705184397,204.735416665711));
#34834=CARTESIAN_POINT('Ctrl Pts',(25.798460424913,62.70446530261,204.677083332377));
#34835=CARTESIAN_POINT('Ctrl Pts',(25.187903481163,62.3519600867804,204.618749999044));
#34836=CARTESIAN_POINT('Ctrl Pts',(24.577346537413,62.70446530261,204.560416665711));
#34837=CARTESIAN_POINT('Ctrl Pts',(23.966789593663,63.0569705184397,204.502083332377));
#34838=CARTESIAN_POINT('Ctrl Pts',(23.966789593663,63.761980950099,204.443749999044));
#34839=CARTESIAN_POINT('Origin',(25.1879034811629,63.761980950099,212.406249999044));
#34840=CARTESIAN_POINT('',(23.966789593663,63.761980950099,205.843749999044));
#34841=CARTESIAN_POINT('',(23.966789593663,63.761980950099,205.668749999044));
#34842=CARTESIAN_POINT('',(23.9667895936629,63.761980950099,212.406249999044));
#34843=CARTESIAN_POINT('Ctrl Pts',(23.966789593663,63.761980950099,205.668749999044));
#34844=CARTESIAN_POINT('Ctrl Pts',(23.966789593663,64.4669913817583,205.610416665711));
#34845=CARTESIAN_POINT('Ctrl Pts',(24.577346537413,64.819496597588,205.552083332377));
#34846=CARTESIAN_POINT('Ctrl Pts',(25.187903481163,65.1720018134176,205.493749999044));
#34847=CARTESIAN_POINT('Ctrl Pts',(25.798460424913,64.819496597588,205.435416665711));
#34848=CARTESIAN_POINT('Ctrl Pts',(26.409017368663,64.4669913817583,205.377083332377));
#34849=CARTESIAN_POINT('Ctrl Pts',(26.409017368663,63.761980950099,205.318749999044));
#34850=CARTESIAN_POINT('Ctrl Pts',(26.409017368663,63.0569705184397,205.260416665711));
#34851=CARTESIAN_POINT('Ctrl Pts',(25.798460424913,62.70446530261,205.202083332377));
#34852=CARTESIAN_POINT('Ctrl Pts',(25.187903481163,62.3519600867804,205.143749999044));
#34853=CARTESIAN_POINT('Ctrl Pts',(24.577346537413,62.70446530261,205.085416665711));
#34854=CARTESIAN_POINT('Ctrl Pts',(23.966789593663,63.0569705184397,205.027083332377));
#34855=CARTESIAN_POINT('Ctrl Pts',(23.966789593663,63.761980950099,204.968749999044));
#34856=CARTESIAN_POINT('Ctrl Pts',(23.966789593663,63.761980950099,205.843749999044));
#34857=CARTESIAN_POINT('Ctrl Pts',(23.966789593663,64.4669913817583,205.785416665711));
#34858=CARTESIAN_POINT('Ctrl Pts',(24.577346537413,64.819496597588,205.727083332377));
#34859=CARTESIAN_POINT('Ctrl Pts',(25.187903481163,65.1720018134176,205.668749999044));
#34860=CARTESIAN_POINT('Ctrl Pts',(25.798460424913,64.819496597588,205.610416665711));
#34861=CARTESIAN_POINT('Ctrl Pts',(26.409017368663,64.4669913817583,205.552083332377));
#34862=CARTESIAN_POINT('Ctrl Pts',(26.409017368663,63.761980950099,205.493749999044));
#34863=CARTESIAN_POINT('Ctrl Pts',(26.409017368663,63.0569705184397,205.435416665711));
#34864=CARTESIAN_POINT('Ctrl Pts',(25.798460424913,62.70446530261,205.377083332377));
#34865=CARTESIAN_POINT('Ctrl Pts',(25.187903481163,62.3519600867804,205.318749999044));
#34866=CARTESIAN_POINT('Ctrl Pts',(24.577346537413,62.70446530261,205.260416665711));
#34867=CARTESIAN_POINT('Ctrl Pts',(23.966789593663,63.0569705184397,205.202083332377));
#34868=CARTESIAN_POINT('Ctrl Pts',(23.966789593663,63.761980950099,205.143749999044));
#34869=CARTESIAN_POINT('Origin',(25.1879034811629,63.761980950099,212.406249999044));
#34870=CARTESIAN_POINT('',(23.966789593663,63.761980950099,206.543749999044));
#34871=CARTESIAN_POINT('',(23.966789593663,63.761980950099,206.368749999044));
#34872=CARTESIAN_POINT('',(23.9667895936629,63.761980950099,212.406249999044));
#34873=CARTESIAN_POINT('Ctrl Pts',(23.966789593663,63.761980950099,206.368749999044));
#34874=CARTESIAN_POINT('Ctrl Pts',(23.966789593663,64.4669913817583,206.310416665711));
#34875=CARTESIAN_POINT('Ctrl Pts',(24.577346537413,64.819496597588,206.252083332377));
#34876=CARTESIAN_POINT('Ctrl Pts',(25.187903481163,65.1720018134176,206.193749999044));
#34877=CARTESIAN_POINT('Ctrl Pts',(25.798460424913,64.819496597588,206.135416665711));
#34878=CARTESIAN_POINT('Ctrl Pts',(26.409017368663,64.4669913817583,206.077083332377));
#34879=CARTESIAN_POINT('Ctrl Pts',(26.409017368663,63.761980950099,206.018749999044));
#34880=CARTESIAN_POINT('Ctrl Pts',(26.409017368663,63.0569705184397,205.960416665711));
#34881=CARTESIAN_POINT('Ctrl Pts',(25.798460424913,62.70446530261,205.902083332377));
#34882=CARTESIAN_POINT('Ctrl Pts',(25.187903481163,62.3519600867804,205.843749999044));
#34883=CARTESIAN_POINT('Ctrl Pts',(24.577346537413,62.70446530261,205.785416665711));
#34884=CARTESIAN_POINT('Ctrl Pts',(23.966789593663,63.0569705184397,205.727083332377));
#34885=CARTESIAN_POINT('Ctrl Pts',(23.966789593663,63.761980950099,205.668749999044));
#34886=CARTESIAN_POINT('Ctrl Pts',(23.966789593663,63.761980950099,206.543749999044));
#34887=CARTESIAN_POINT('Ctrl Pts',(23.966789593663,64.4669913817583,206.485416665711));
#34888=CARTESIAN_POINT('Ctrl Pts',(24.577346537413,64.819496597588,206.427083332377));
#34889=CARTESIAN_POINT('Ctrl Pts',(25.187903481163,65.1720018134176,206.368749999044));
#34890=CARTESIAN_POINT('Ctrl Pts',(25.798460424913,64.819496597588,206.310416665711));
#34891=CARTESIAN_POINT('Ctrl Pts',(26.409017368663,64.4669913817583,206.252083332377));
#34892=CARTESIAN_POINT('Ctrl Pts',(26.409017368663,63.761980950099,206.193749999044));
#34893=CARTESIAN_POINT('Ctrl Pts',(26.409017368663,63.0569705184397,206.135416665711));
#34894=CARTESIAN_POINT('Ctrl Pts',(25.798460424913,62.70446530261,206.077083332377));
#34895=CARTESIAN_POINT('Ctrl Pts',(25.187903481163,62.3519600867804,206.018749999044));
#34896=CARTESIAN_POINT('Ctrl Pts',(24.577346537413,62.70446530261,205.960416665711));
#34897=CARTESIAN_POINT('Ctrl Pts',(23.966789593663,63.0569705184397,205.902083332377));
#34898=CARTESIAN_POINT('Ctrl Pts',(23.966789593663,63.761980950099,205.843749999044));
#34899=CARTESIAN_POINT('Origin',(25.1879034811629,63.761980950099,212.406249999044));
#34900=CARTESIAN_POINT('',(23.966789593663,63.761980950099,207.243749999044));
#34901=CARTESIAN_POINT('',(23.966789593663,63.761980950099,207.068749999044));
#34902=CARTESIAN_POINT('',(23.9667895936629,63.761980950099,212.406249999044));
#34903=CARTESIAN_POINT('Ctrl Pts',(23.966789593663,63.761980950099,207.068749999044));
#34904=CARTESIAN_POINT('Ctrl Pts',(23.966789593663,64.4669913817583,207.010416665711));
#34905=CARTESIAN_POINT('Ctrl Pts',(24.577346537413,64.819496597588,206.952083332377));
#34906=CARTESIAN_POINT('Ctrl Pts',(25.187903481163,65.1720018134176,206.893749999044));
#34907=CARTESIAN_POINT('Ctrl Pts',(25.798460424913,64.819496597588,206.835416665711));
#34908=CARTESIAN_POINT('Ctrl Pts',(26.409017368663,64.4669913817583,206.777083332377));
#34909=CARTESIAN_POINT('Ctrl Pts',(26.409017368663,63.761980950099,206.718749999044));
#34910=CARTESIAN_POINT('Ctrl Pts',(26.409017368663,63.0569705184397,206.660416665711));
#34911=CARTESIAN_POINT('Ctrl Pts',(25.798460424913,62.70446530261,206.602083332377));
#34912=CARTESIAN_POINT('Ctrl Pts',(25.187903481163,62.3519600867804,206.543749999044));
#34913=CARTESIAN_POINT('Ctrl Pts',(24.577346537413,62.70446530261,206.485416665711));
#34914=CARTESIAN_POINT('Ctrl Pts',(23.966789593663,63.0569705184397,206.427083332377));
#34915=CARTESIAN_POINT('Ctrl Pts',(23.966789593663,63.761980950099,206.368749999044));
#34916=CARTESIAN_POINT('Ctrl Pts',(23.966789593663,63.761980950099,207.243749999044));
#34917=CARTESIAN_POINT('Ctrl Pts',(23.966789593663,64.4669913817583,207.185416665711));
#34918=CARTESIAN_POINT('Ctrl Pts',(24.577346537413,64.819496597588,207.127083332377));
#34919=CARTESIAN_POINT('Ctrl Pts',(25.187903481163,65.1720018134176,207.068749999044));
#34920=CARTESIAN_POINT('Ctrl Pts',(25.798460424913,64.819496597588,207.010416665711));
#34921=CARTESIAN_POINT('Ctrl Pts',(26.409017368663,64.4669913817583,206.952083332377));
#34922=CARTESIAN_POINT('Ctrl Pts',(26.409017368663,63.761980950099,206.893749999044));
#34923=CARTESIAN_POINT('Ctrl Pts',(26.409017368663,63.0569705184397,206.835416665711));
#34924=CARTESIAN_POINT('Ctrl Pts',(25.798460424913,62.70446530261,206.777083332377));
#34925=CARTESIAN_POINT('Ctrl Pts',(25.187903481163,62.3519600867804,206.718749999044));
#34926=CARTESIAN_POINT('Ctrl Pts',(24.577346537413,62.70446530261,206.660416665711));
#34927=CARTESIAN_POINT('Ctrl Pts',(23.966789593663,63.0569705184397,206.602083332377));
#34928=CARTESIAN_POINT('Ctrl Pts',(23.966789593663,63.761980950099,206.543749999044));
#34929=CARTESIAN_POINT('Origin',(25.1879034811629,63.761980950099,212.406249999044));
#34930=CARTESIAN_POINT('',(23.966789593663,63.761980950099,207.943749999044));
#34931=CARTESIAN_POINT('',(23.966789593663,63.761980950099,207.768749999044));
#34932=CARTESIAN_POINT('',(23.9667895936629,63.761980950099,212.406249999044));
#34933=CARTESIAN_POINT('Ctrl Pts',(23.966789593663,63.761980950099,207.768749999044));
#34934=CARTESIAN_POINT('Ctrl Pts',(23.966789593663,64.4669913817583,207.710416665711));
#34935=CARTESIAN_POINT('Ctrl Pts',(24.577346537413,64.819496597588,207.652083332377));
#34936=CARTESIAN_POINT('Ctrl Pts',(25.187903481163,65.1720018134176,207.593749999044));
#34937=CARTESIAN_POINT('Ctrl Pts',(25.798460424913,64.819496597588,207.535416665711));
#34938=CARTESIAN_POINT('Ctrl Pts',(26.409017368663,64.4669913817583,207.477083332377));
#34939=CARTESIAN_POINT('Ctrl Pts',(26.409017368663,63.761980950099,207.418749999044));
#34940=CARTESIAN_POINT('Ctrl Pts',(26.409017368663,63.0569705184397,207.360416665711));
#34941=CARTESIAN_POINT('Ctrl Pts',(25.798460424913,62.70446530261,207.302083332377));
#34942=CARTESIAN_POINT('Ctrl Pts',(25.187903481163,62.3519600867804,207.243749999044));
#34943=CARTESIAN_POINT('Ctrl Pts',(24.577346537413,62.70446530261,207.185416665711));
#34944=CARTESIAN_POINT('Ctrl Pts',(23.966789593663,63.0569705184397,207.127083332377));
#34945=CARTESIAN_POINT('Ctrl Pts',(23.966789593663,63.761980950099,207.068749999044));
#34946=CARTESIAN_POINT('Ctrl Pts',(23.966789593663,63.761980950099,207.943749999044));
#34947=CARTESIAN_POINT('Ctrl Pts',(23.966789593663,64.4669913817583,207.885416665711));
#34948=CARTESIAN_POINT('Ctrl Pts',(24.577346537413,64.819496597588,207.827083332377));
#34949=CARTESIAN_POINT('Ctrl Pts',(25.187903481163,65.1720018134176,207.768749999044));
#34950=CARTESIAN_POINT('Ctrl Pts',(25.798460424913,64.819496597588,207.710416665711));
#34951=CARTESIAN_POINT('Ctrl Pts',(26.409017368663,64.4669913817583,207.652083332377));
#34952=CARTESIAN_POINT('Ctrl Pts',(26.409017368663,63.761980950099,207.593749999044));
#34953=CARTESIAN_POINT('Ctrl Pts',(26.409017368663,63.0569705184397,207.535416665711));
#34954=CARTESIAN_POINT('Ctrl Pts',(25.798460424913,62.70446530261,207.477083332377));
#34955=CARTESIAN_POINT('Ctrl Pts',(25.187903481163,62.3519600867804,207.418749999044));
#34956=CARTESIAN_POINT('Ctrl Pts',(24.577346537413,62.70446530261,207.360416665711));
#34957=CARTESIAN_POINT('Ctrl Pts',(23.966789593663,63.0569705184397,207.302083332377));
#34958=CARTESIAN_POINT('Ctrl Pts',(23.966789593663,63.761980950099,207.243749999044));
#34959=CARTESIAN_POINT('Origin',(25.1879034811629,63.761980950099,212.406249999044));
#34960=CARTESIAN_POINT('',(23.966789593663,63.761980950099,208.643749999044));
#34961=CARTESIAN_POINT('',(23.966789593663,63.761980950099,208.468749999044));
#34962=CARTESIAN_POINT('',(23.9667895936629,63.761980950099,212.406249999044));
#34963=CARTESIAN_POINT('Ctrl Pts',(23.966789593663,63.761980950099,208.468749999044));
#34964=CARTESIAN_POINT('Ctrl Pts',(23.966789593663,64.4669913817583,208.410416665711));
#34965=CARTESIAN_POINT('Ctrl Pts',(24.577346537413,64.819496597588,208.352083332377));
#34966=CARTESIAN_POINT('Ctrl Pts',(25.187903481163,65.1720018134176,208.293749999044));
#34967=CARTESIAN_POINT('Ctrl Pts',(25.798460424913,64.819496597588,208.235416665711));
#34968=CARTESIAN_POINT('Ctrl Pts',(26.409017368663,64.4669913817583,208.177083332377));
#34969=CARTESIAN_POINT('Ctrl Pts',(26.409017368663,63.761980950099,208.118749999044));
#34970=CARTESIAN_POINT('Ctrl Pts',(26.409017368663,63.0569705184397,208.060416665711));
#34971=CARTESIAN_POINT('Ctrl Pts',(25.798460424913,62.70446530261,208.002083332377));
#34972=CARTESIAN_POINT('Ctrl Pts',(25.187903481163,62.3519600867804,207.943749999044));
#34973=CARTESIAN_POINT('Ctrl Pts',(24.577346537413,62.70446530261,207.885416665711));
#34974=CARTESIAN_POINT('Ctrl Pts',(23.966789593663,63.0569705184397,207.827083332377));
#34975=CARTESIAN_POINT('Ctrl Pts',(23.966789593663,63.761980950099,207.768749999044));
#34976=CARTESIAN_POINT('Ctrl Pts',(23.966789593663,63.761980950099,208.643749999044));
#34977=CARTESIAN_POINT('Ctrl Pts',(23.966789593663,64.4669913817583,208.585416665711));
#34978=CARTESIAN_POINT('Ctrl Pts',(24.577346537413,64.819496597588,208.527083332377));
#34979=CARTESIAN_POINT('Ctrl Pts',(25.187903481163,65.1720018134176,208.468749999044));
#34980=CARTESIAN_POINT('Ctrl Pts',(25.798460424913,64.819496597588,208.410416665711));
#34981=CARTESIAN_POINT('Ctrl Pts',(26.409017368663,64.4669913817583,208.352083332377));
#34982=CARTESIAN_POINT('Ctrl Pts',(26.409017368663,63.761980950099,208.293749999044));
#34983=CARTESIAN_POINT('Ctrl Pts',(26.409017368663,63.0569705184397,208.235416665711));
#34984=CARTESIAN_POINT('Ctrl Pts',(25.798460424913,62.70446530261,208.177083332377));
#34985=CARTESIAN_POINT('Ctrl Pts',(25.187903481163,62.3519600867804,208.118749999044));
#34986=CARTESIAN_POINT('Ctrl Pts',(24.577346537413,62.70446530261,208.060416665711));
#34987=CARTESIAN_POINT('Ctrl Pts',(23.966789593663,63.0569705184397,208.002083332377));
#34988=CARTESIAN_POINT('Ctrl Pts',(23.966789593663,63.761980950099,207.943749999044));
#34989=CARTESIAN_POINT('Origin',(25.1879034811629,63.761980950099,212.406249999044));
#34990=CARTESIAN_POINT('',(23.966789593663,63.761980950099,209.343749999044));
#34991=CARTESIAN_POINT('',(23.966789593663,63.761980950099,209.168749999044));
#34992=CARTESIAN_POINT('',(23.9667895936629,63.761980950099,212.406249999044));
#34993=CARTESIAN_POINT('Ctrl Pts',(23.966789593663,63.761980950099,209.168749999044));
#34994=CARTESIAN_POINT('Ctrl Pts',(23.966789593663,64.4669913817583,209.110416665711));
#34995=CARTESIAN_POINT('Ctrl Pts',(24.577346537413,64.819496597588,209.052083332377));
#34996=CARTESIAN_POINT('Ctrl Pts',(25.187903481163,65.1720018134176,208.993749999044));
#34997=CARTESIAN_POINT('Ctrl Pts',(25.798460424913,64.819496597588,208.935416665711));
#34998=CARTESIAN_POINT('Ctrl Pts',(26.409017368663,64.4669913817583,208.877083332377));
#34999=CARTESIAN_POINT('Ctrl Pts',(26.409017368663,63.761980950099,208.818749999044));
#35000=CARTESIAN_POINT('Ctrl Pts',(26.409017368663,63.0569705184397,208.760416665711));
#35001=CARTESIAN_POINT('Ctrl Pts',(25.798460424913,62.70446530261,208.702083332377));
#35002=CARTESIAN_POINT('Ctrl Pts',(25.187903481163,62.3519600867804,208.643749999044));
#35003=CARTESIAN_POINT('Ctrl Pts',(24.577346537413,62.70446530261,208.585416665711));
#35004=CARTESIAN_POINT('Ctrl Pts',(23.966789593663,63.0569705184397,208.527083332377));
#35005=CARTESIAN_POINT('Ctrl Pts',(23.966789593663,63.761980950099,208.468749999044));
#35006=CARTESIAN_POINT('Ctrl Pts',(23.966789593663,63.761980950099,209.343749999044));
#35007=CARTESIAN_POINT('Ctrl Pts',(23.966789593663,64.4669913817583,209.285416665711));
#35008=CARTESIAN_POINT('Ctrl Pts',(24.577346537413,64.819496597588,209.227083332377));
#35009=CARTESIAN_POINT('Ctrl Pts',(25.187903481163,65.1720018134176,209.168749999044));
#35010=CARTESIAN_POINT('Ctrl Pts',(25.798460424913,64.819496597588,209.110416665711));
#35011=CARTESIAN_POINT('Ctrl Pts',(26.409017368663,64.4669913817583,209.052083332377));
#35012=CARTESIAN_POINT('Ctrl Pts',(26.409017368663,63.761980950099,208.993749999044));
#35013=CARTESIAN_POINT('Ctrl Pts',(26.409017368663,63.0569705184397,208.935416665711));
#35014=CARTESIAN_POINT('Ctrl Pts',(25.798460424913,62.70446530261,208.877083332377));
#35015=CARTESIAN_POINT('Ctrl Pts',(25.187903481163,62.3519600867804,208.818749999044));
#35016=CARTESIAN_POINT('Ctrl Pts',(24.577346537413,62.70446530261,208.760416665711));
#35017=CARTESIAN_POINT('Ctrl Pts',(23.966789593663,63.0569705184397,208.702083332377));
#35018=CARTESIAN_POINT('Ctrl Pts',(23.966789593663,63.761980950099,208.643749999044));
#35019=CARTESIAN_POINT('Origin',(25.1879034811629,63.761980950099,212.406249999044));
#35020=CARTESIAN_POINT('',(23.966789593663,63.761980950099,210.043749999044));
#35021=CARTESIAN_POINT('',(23.966789593663,63.761980950099,209.868749999044));
#35022=CARTESIAN_POINT('',(23.9667895936629,63.761980950099,212.406249999044));
#35023=CARTESIAN_POINT('Ctrl Pts',(23.966789593663,63.761980950099,209.868749999044));
#35024=CARTESIAN_POINT('Ctrl Pts',(23.966789593663,64.4669913817583,209.810416665711));
#35025=CARTESIAN_POINT('Ctrl Pts',(24.577346537413,64.819496597588,209.752083332377));
#35026=CARTESIAN_POINT('Ctrl Pts',(25.187903481163,65.1720018134176,209.693749999044));
#35027=CARTESIAN_POINT('Ctrl Pts',(25.798460424913,64.819496597588,209.635416665711));
#35028=CARTESIAN_POINT('Ctrl Pts',(26.409017368663,64.4669913817583,209.577083332377));
#35029=CARTESIAN_POINT('Ctrl Pts',(26.409017368663,63.761980950099,209.518749999044));
#35030=CARTESIAN_POINT('Ctrl Pts',(26.409017368663,63.0569705184397,209.460416665711));
#35031=CARTESIAN_POINT('Ctrl Pts',(25.798460424913,62.70446530261,209.402083332377));
#35032=CARTESIAN_POINT('Ctrl Pts',(25.187903481163,62.3519600867804,209.343749999044));
#35033=CARTESIAN_POINT('Ctrl Pts',(24.577346537413,62.70446530261,209.285416665711));
#35034=CARTESIAN_POINT('Ctrl Pts',(23.966789593663,63.0569705184397,209.227083332377));
#35035=CARTESIAN_POINT('Ctrl Pts',(23.966789593663,63.761980950099,209.168749999044));
#35036=CARTESIAN_POINT('Ctrl Pts',(23.966789593663,63.761980950099,210.043749999044));
#35037=CARTESIAN_POINT('Ctrl Pts',(23.966789593663,64.4669913817583,209.985416665711));
#35038=CARTESIAN_POINT('Ctrl Pts',(24.577346537413,64.819496597588,209.927083332377));
#35039=CARTESIAN_POINT('Ctrl Pts',(25.187903481163,65.1720018134176,209.868749999044));
#35040=CARTESIAN_POINT('Ctrl Pts',(25.798460424913,64.819496597588,209.810416665711));
#35041=CARTESIAN_POINT('Ctrl Pts',(26.409017368663,64.4669913817583,209.752083332377));
#35042=CARTESIAN_POINT('Ctrl Pts',(26.409017368663,63.761980950099,209.693749999044));
#35043=CARTESIAN_POINT('Ctrl Pts',(26.409017368663,63.0569705184397,209.635416665711));
#35044=CARTESIAN_POINT('Ctrl Pts',(25.798460424913,62.70446530261,209.577083332377));
#35045=CARTESIAN_POINT('Ctrl Pts',(25.187903481163,62.3519600867804,209.518749999044));
#35046=CARTESIAN_POINT('Ctrl Pts',(24.577346537413,62.70446530261,209.460416665711));
#35047=CARTESIAN_POINT('Ctrl Pts',(23.966789593663,63.0569705184397,209.402083332377));
#35048=CARTESIAN_POINT('Ctrl Pts',(23.966789593663,63.761980950099,209.343749999044));
#35049=CARTESIAN_POINT('Origin',(25.1879034811629,63.761980950099,212.406249999044));
#35050=CARTESIAN_POINT('',(23.966789593663,63.761980950099,210.743749999044));
#35051=CARTESIAN_POINT('',(23.966789593663,63.761980950099,210.568749999044));
#35052=CARTESIAN_POINT('',(23.9667895936629,63.761980950099,212.406249999044));
#35053=CARTESIAN_POINT('Ctrl Pts',(23.966789593663,63.761980950099,210.568749999044));
#35054=CARTESIAN_POINT('Ctrl Pts',(23.966789593663,64.4669913817583,210.510416665711));
#35055=CARTESIAN_POINT('Ctrl Pts',(24.577346537413,64.819496597588,210.452083332377));
#35056=CARTESIAN_POINT('Ctrl Pts',(25.187903481163,65.1720018134176,210.393749999044));
#35057=CARTESIAN_POINT('Ctrl Pts',(25.798460424913,64.819496597588,210.335416665711));
#35058=CARTESIAN_POINT('Ctrl Pts',(26.409017368663,64.4669913817583,210.277083332377));
#35059=CARTESIAN_POINT('Ctrl Pts',(26.409017368663,63.761980950099,210.218749999044));
#35060=CARTESIAN_POINT('Ctrl Pts',(26.409017368663,63.0569705184397,210.160416665711));
#35061=CARTESIAN_POINT('Ctrl Pts',(25.798460424913,62.70446530261,210.102083332377));
#35062=CARTESIAN_POINT('Ctrl Pts',(25.187903481163,62.3519600867804,210.043749999044));
#35063=CARTESIAN_POINT('Ctrl Pts',(24.577346537413,62.70446530261,209.985416665711));
#35064=CARTESIAN_POINT('Ctrl Pts',(23.966789593663,63.0569705184397,209.927083332377));
#35065=CARTESIAN_POINT('Ctrl Pts',(23.966789593663,63.761980950099,209.868749999044));
#35066=CARTESIAN_POINT('Ctrl Pts',(23.966789593663,63.761980950099,210.743749999044));
#35067=CARTESIAN_POINT('Ctrl Pts',(23.966789593663,64.4669913817583,210.685416665711));
#35068=CARTESIAN_POINT('Ctrl Pts',(24.577346537413,64.819496597588,210.627083332377));
#35069=CARTESIAN_POINT('Ctrl Pts',(25.187903481163,65.1720018134176,210.568749999044));
#35070=CARTESIAN_POINT('Ctrl Pts',(25.798460424913,64.819496597588,210.510416665711));
#35071=CARTESIAN_POINT('Ctrl Pts',(26.409017368663,64.4669913817583,210.452083332377));
#35072=CARTESIAN_POINT('Ctrl Pts',(26.409017368663,63.761980950099,210.393749999044));
#35073=CARTESIAN_POINT('Ctrl Pts',(26.409017368663,63.0569705184397,210.335416665711));
#35074=CARTESIAN_POINT('Ctrl Pts',(25.798460424913,62.70446530261,210.277083332377));
#35075=CARTESIAN_POINT('Ctrl Pts',(25.187903481163,62.3519600867804,210.218749999044));
#35076=CARTESIAN_POINT('Ctrl Pts',(24.577346537413,62.70446530261,210.160416665711));
#35077=CARTESIAN_POINT('Ctrl Pts',(23.966789593663,63.0569705184397,210.102083332377));
#35078=CARTESIAN_POINT('Ctrl Pts',(23.966789593663,63.761980950099,210.043749999044));
#35079=CARTESIAN_POINT('Origin',(25.1879034811629,63.761980950099,212.406249999044));
#35080=CARTESIAN_POINT('',(23.966789593663,63.761980950099,211.443749999044));
#35081=CARTESIAN_POINT('',(23.966789593663,63.761980950099,211.268749999044));
#35082=CARTESIAN_POINT('',(23.9667895936629,63.761980950099,212.406249999044));
#35083=CARTESIAN_POINT('Ctrl Pts',(23.966789593663,63.761980950099,211.268749999044));
#35084=CARTESIAN_POINT('Ctrl Pts',(23.966789593663,64.4669913817583,211.210416665711));
#35085=CARTESIAN_POINT('Ctrl Pts',(24.577346537413,64.819496597588,211.152083332377));
#35086=CARTESIAN_POINT('Ctrl Pts',(25.187903481163,65.1720018134176,211.093749999044));
#35087=CARTESIAN_POINT('Ctrl Pts',(25.798460424913,64.819496597588,211.035416665711));
#35088=CARTESIAN_POINT('Ctrl Pts',(26.409017368663,64.4669913817583,210.977083332377));
#35089=CARTESIAN_POINT('Ctrl Pts',(26.409017368663,63.761980950099,210.918749999044));
#35090=CARTESIAN_POINT('Ctrl Pts',(26.409017368663,63.0569705184397,210.860416665711));
#35091=CARTESIAN_POINT('Ctrl Pts',(25.798460424913,62.70446530261,210.802083332377));
#35092=CARTESIAN_POINT('Ctrl Pts',(25.187903481163,62.3519600867804,210.743749999044));
#35093=CARTESIAN_POINT('Ctrl Pts',(24.577346537413,62.70446530261,210.685416665711));
#35094=CARTESIAN_POINT('Ctrl Pts',(23.966789593663,63.0569705184397,210.627083332377));
#35095=CARTESIAN_POINT('Ctrl Pts',(23.966789593663,63.761980950099,210.568749999044));
#35096=CARTESIAN_POINT('Ctrl Pts',(23.966789593663,63.761980950099,211.443749999044));
#35097=CARTESIAN_POINT('Ctrl Pts',(23.966789593663,64.4669913817583,211.385416665711));
#35098=CARTESIAN_POINT('Ctrl Pts',(24.577346537413,64.819496597588,211.327083332377));
#35099=CARTESIAN_POINT('Ctrl Pts',(25.187903481163,65.1720018134176,211.268749999044));
#35100=CARTESIAN_POINT('Ctrl Pts',(25.798460424913,64.819496597588,211.210416665711));
#35101=CARTESIAN_POINT('Ctrl Pts',(26.409017368663,64.4669913817583,211.152083332377));
#35102=CARTESIAN_POINT('Ctrl Pts',(26.409017368663,63.761980950099,211.093749999044));
#35103=CARTESIAN_POINT('Ctrl Pts',(26.409017368663,63.0569705184397,211.035416665711));
#35104=CARTESIAN_POINT('Ctrl Pts',(25.798460424913,62.70446530261,210.977083332377));
#35105=CARTESIAN_POINT('Ctrl Pts',(25.187903481163,62.3519600867804,210.918749999044));
#35106=CARTESIAN_POINT('Ctrl Pts',(24.577346537413,62.70446530261,210.860416665711));
#35107=CARTESIAN_POINT('Ctrl Pts',(23.966789593663,63.0569705184397,210.802083332377));
#35108=CARTESIAN_POINT('Ctrl Pts',(23.966789593663,63.761980950099,210.743749999044));
#35109=CARTESIAN_POINT('Origin',(25.1879034811629,63.761980950099,212.406249999044));
#35110=CARTESIAN_POINT('',(23.966789593663,63.761980950099,212.143749999044));
#35111=CARTESIAN_POINT('',(23.966789593663,63.761980950099,211.968749999044));
#35112=CARTESIAN_POINT('',(23.9667895936629,63.761980950099,212.406249999044));
#35113=CARTESIAN_POINT('',(26.409017368663,63.761980950099,212.493749999044));
#35114=CARTESIAN_POINT('Ctrl Pts',(26.409017368663,63.761980950099,212.493749999044));
#35115=CARTESIAN_POINT('Ctrl Pts',(26.409017368663,63.0569705184397,212.435416665711));
#35116=CARTESIAN_POINT('Ctrl Pts',(25.798460424913,62.70446530261,212.377083332377));
#35117=CARTESIAN_POINT('Ctrl Pts',(25.187903481163,62.3519600867804,212.318749999044));
#35118=CARTESIAN_POINT('Ctrl Pts',(24.577346537413,62.70446530261,212.260416665711));
#35119=CARTESIAN_POINT('Ctrl Pts',(23.966789593663,63.0569705184397,212.202083332377));
#35120=CARTESIAN_POINT('Ctrl Pts',(23.966789593663,63.761980950099,212.143749999044));
#35121=CARTESIAN_POINT('',(26.409017368663,63.761980950099,212.318749999044));
#35122=CARTESIAN_POINT('',(26.409017368663,63.761980950099,212.406249999044));
#35123=CARTESIAN_POINT('Ctrl Pts',(26.409017368663,63.761980950099,212.318749999044));
#35124=CARTESIAN_POINT('Ctrl Pts',(26.409017368663,63.0569705184397,212.260416665711));
#35125=CARTESIAN_POINT('Ctrl Pts',(25.798460424913,62.70446530261,212.202083332377));
#35126=CARTESIAN_POINT('Ctrl Pts',(25.187903481163,62.3519600867804,212.143749999044));
#35127=CARTESIAN_POINT('Ctrl Pts',(24.577346537413,62.70446530261,212.085416665711));
#35128=CARTESIAN_POINT('Ctrl Pts',(23.966789593663,63.0569705184397,212.027083332377));
#35129=CARTESIAN_POINT('Ctrl Pts',(23.966789593663,63.761980950099,211.968749999044));
#35130=CARTESIAN_POINT('Origin',(43.0811453810944,77.1117683798101,211.));
#35131=CARTESIAN_POINT('',(41.4811453810944,77.1117683798101,212.));
#35132=CARTESIAN_POINT('Origin',(43.0811453810944,77.1117683798101,212.));
#35133=CARTESIAN_POINT('',(41.4811453810944,77.1117683798101,211.8));
#35134=CARTESIAN_POINT('',(41.4811453810944,77.1117683798101,211.));
#35135=CARTESIAN_POINT('Origin',(43.0811453810944,77.1117683798101,211.8));
#35136=CARTESIAN_POINT('Origin',(19.9513700273636,43.5818784659284,205.8));
#35137=CARTESIAN_POINT('',(18.4596441794768,43.5818784659284,212.8));
#35138=CARTESIAN_POINT('Origin',(19.9513700273636,43.5818784659284,212.8));
#35139=CARTESIAN_POINT('',(18.4596441794768,43.5818784659284,205.8));
#35140=CARTESIAN_POINT('',(18.4596441794768,43.5818784659284,205.8));
#35141=CARTESIAN_POINT('Origin',(19.9513700273636,43.5818784659284,205.8));
#35142=CARTESIAN_POINT('Origin',(43.0811453810902,77.1117683798122,214.746949994782));
#35143=CARTESIAN_POINT('',(44.1230495436541,77.1117683798122,210.3));
#35144=CARTESIAN_POINT('Origin',(43.0811453810904,77.1117683798123,210.3));
#35145=CARTESIAN_POINT('',(44.1230495436541,77.1117683798122,211.));
#35146=CARTESIAN_POINT('',(44.1230495436541,77.1117683798122,214.746949994782));
#35147=CARTESIAN_POINT('Origin',(43.0811453810902,77.1117683798122,211.));
#35148=CARTESIAN_POINT('Origin',(25.187903481163,63.761980950099,202.));
#35149=CARTESIAN_POINT('',(13.387903481163,63.761980950099,202.2));
#35150=CARTESIAN_POINT('Origin',(25.187903481163,63.761980950099,202.2));
#35151=CARTESIAN_POINT('',(13.187903481163,63.761980950099,202.));
#35152=CARTESIAN_POINT('Origin',(13.387903481163,63.761980950099,202.));
#35153=CARTESIAN_POINT('',(37.187903481163,63.761980950099,202.));
#35154=CARTESIAN_POINT('Origin',(25.187903481163,63.761980950099,202.));
#35155=CARTESIAN_POINT('Origin',(25.187903481163,63.761980950099,202.));
#35156=CARTESIAN_POINT('Origin',(25.187903481163,63.761980950099,201.4));
#35157=CARTESIAN_POINT('',(37.187903481163,63.761980950099,201.4));
#35158=CARTESIAN_POINT('',(13.187903481163,63.761980950099,201.4));
#35159=CARTESIAN_POINT('Origin',(25.187903481163,63.761980950099,201.4));
#35160=CARTESIAN_POINT('Origin',(25.187903481163,63.761980950099,201.4));
#35161=CARTESIAN_POINT('',(13.387903481163,63.761980950099,201.2));
#35162=CARTESIAN_POINT('Origin',(13.387903481163,63.761980950099,201.4));
#35163=CARTESIAN_POINT('Origin',(25.187903481163,63.761980950099,201.2));
#35164=CARTESIAN_POINT('Origin',(25.187903481163,63.761980950099,202.));
#35165=CARTESIAN_POINT('',(28.437903481163,63.761980950099,202.));
#35166=CARTESIAN_POINT('',(21.937903481163,63.761980950099,202.));
#35167=CARTESIAN_POINT('Origin',(25.187903481163,63.761980950099,202.));
#35168=CARTESIAN_POINT('Origin',(25.187903481163,63.761980950099,202.));
#35169=CARTESIAN_POINT('',(21.737903481163,63.761980950099,202.2));
#35170=CARTESIAN_POINT('Origin',(21.737903481163,63.761980950099,202.));
#35171=CARTESIAN_POINT('Origin',(25.187903481163,63.761980950099,202.2));
#35172=CARTESIAN_POINT('Origin',(25.187903481163,63.761980950099,201.4));
#35173=CARTESIAN_POINT('',(21.737903481163,63.761980950099,201.2));
#35174=CARTESIAN_POINT('Origin',(25.187903481163,63.761980950099,201.2));
#35175=CARTESIAN_POINT('',(21.937903481163,63.761980950099,201.4));
#35176=CARTESIAN_POINT('Origin',(21.737903481163,63.761980950099,201.4));
#35177=CARTESIAN_POINT('',(28.437903481163,63.761980950099,201.4));
#35178=CARTESIAN_POINT('Origin',(25.187903481163,63.761980950099,201.4));
#35179=CARTESIAN_POINT('Origin',(25.187903481163,63.761980950099,201.4));
#35180=CARTESIAN_POINT('Origin',(25.187903481163,63.761980950099,202.2));
#35181=CARTESIAN_POINT('',(28.437903481163,63.761980950099,202.2));
#35182=CARTESIAN_POINT('Origin',(25.187903481163,63.761980950099,202.2));
#35183=CARTESIAN_POINT('',(37.187903481163,63.761980950099,202.2));
#35184=CARTESIAN_POINT('Origin',(25.187903481163,63.761980950099,201.2));
#35185=CARTESIAN_POINT('Origin',(25.187903481163,63.761980950099,202.2));
#35186=CARTESIAN_POINT('',(18.2509458845758,64.6993278993105,202.2));
#35187=CARTESIAN_POINT('Origin',(25.18790348116,63.761980950101,202.2));
#35188=CARTESIAN_POINT('Origin',(25.187903481163,63.761980950099,202.2));
#35189=CARTESIAN_POINT('',(27.187903481163,63.761980950099,202.2));
#35190=CARTESIAN_POINT('Origin',(25.187903481163,63.761980950099,202.2));
#35191=CARTESIAN_POINT('Origin',(25.1879034811632,63.761980950099,212.406249999044));
#35192=CARTESIAN_POINT('',(26.787903481163,63.761980950099,212.712499998088));
#35193=CARTESIAN_POINT('Ctrl Pts',(26.787903481163,63.761980950099,212.712499998088));
#35194=CARTESIAN_POINT('Ctrl Pts',(26.787903481163,62.8382205193956,212.654166664755));
#35195=CARTESIAN_POINT('Ctrl Pts',(25.987903481163,62.3763403040439,212.595833331421));
#35196=CARTESIAN_POINT('Ctrl Pts',(25.187903481163,61.9144600886922,212.537499998088));
#35197=CARTESIAN_POINT('Ctrl Pts',(24.387903481163,62.3763403040439,212.479166664755));
#35198=CARTESIAN_POINT('Ctrl Pts',(23.587903481163,62.8382205193956,212.420833331421));
#35199=CARTESIAN_POINT('Ctrl Pts',(23.587903481163,63.761980950099,212.362499998088));
#35200=CARTESIAN_POINT('Ctrl Pts',(23.587903481163,64.6857413808024,212.304166664755));
#35201=CARTESIAN_POINT('Ctrl Pts',(24.387903481163,65.1476215961541,212.245833331421));
#35202=CARTESIAN_POINT('Ctrl Pts',(25.187903481163,65.6095018115058,212.187499998088));
#35203=CARTESIAN_POINT('Ctrl Pts',(25.987903481163,65.1476215961541,212.129166664755));
#35204=CARTESIAN_POINT('Ctrl Pts',(26.1767578512194,65.0385864747644,212.115396033605));
#35205=CARTESIAN_POINT('Ctrl Pts',(26.3295442486903,64.882987800176,212.1));
#35206=CARTESIAN_POINT('',(23.587903481163,63.761980950099,212.1));
#35207=CARTESIAN_POINT('Origin',(25.187903481163,63.761980950099,212.1));
#35208=CARTESIAN_POINT('Origin',(25.187903481163,63.761980950099,212.1));
#35209=CARTESIAN_POINT('',(26.787903481163,63.761980950099,212.406249999044));
#35210=CARTESIAN_POINT('Ctrl Pts',(26.787903481163,63.761980950099,212.712499998088));
#35211=CARTESIAN_POINT('Ctrl Pts',(26.787903481163,62.8382205193956,212.654166664755));
#35212=CARTESIAN_POINT('Ctrl Pts',(25.987903481163,62.3763403040439,212.595833331421));
#35213=CARTESIAN_POINT('Ctrl Pts',(25.187903481163,61.9144600886922,212.537499998088));
#35214=CARTESIAN_POINT('Ctrl Pts',(24.387903481163,62.3763403040439,212.479166664755));
#35215=CARTESIAN_POINT('Ctrl Pts',(23.587903481163,62.8382205193956,212.420833331421));
#35216=CARTESIAN_POINT('Ctrl Pts',(23.587903481163,63.761980950099,212.362499998088));
#35217=CARTESIAN_POINT('Ctrl Pts',(23.587903481163,64.6857413808024,212.304166664755));
#35218=CARTESIAN_POINT('Ctrl Pts',(24.387903481163,65.1476215961541,212.245833331421));
#35219=CARTESIAN_POINT('Ctrl Pts',(25.187903481163,65.6095018115058,212.187499998088));
#35220=CARTESIAN_POINT('Ctrl Pts',(25.987903481163,65.1476215961541,212.129166664755));
#35221=CARTESIAN_POINT('Ctrl Pts',(26.787903481163,64.6857413808024,212.070833331422));
#35222=CARTESIAN_POINT('Ctrl Pts',(26.787903481163,63.761980950099,212.012499998088));
#35223=CARTESIAN_POINT('Ctrl Pts',(26.787903481163,62.8382205193956,211.954166664755));
#35224=CARTESIAN_POINT('Ctrl Pts',(25.987903481163,62.3763403040439,211.895833331421));
#35225=CARTESIAN_POINT('Ctrl Pts',(25.187903481163,61.9144600886922,211.837499998088));
#35226=CARTESIAN_POINT('Ctrl Pts',(24.387903481163,62.3763403040439,211.779166664755));
#35227=CARTESIAN_POINT('Ctrl Pts',(23.587903481163,62.8382205193956,211.720833331422));
#35228=CARTESIAN_POINT('Ctrl Pts',(23.587903481163,63.761980950099,211.662499998088));
#35229=CARTESIAN_POINT('Ctrl Pts',(23.587903481163,64.6857413808024,211.604166664755));
#35230=CARTESIAN_POINT('Ctrl Pts',(24.387903481163,65.1476215961541,211.545833331421));
#35231=CARTESIAN_POINT('Ctrl Pts',(25.187903481163,65.6095018115058,211.487499998088));
#35232=CARTESIAN_POINT('Ctrl Pts',(25.987903481163,65.1476215961541,211.429166664755));
#35233=CARTESIAN_POINT('Ctrl Pts',(26.787903481163,64.6857413808024,211.370833331422));
#35234=CARTESIAN_POINT('Ctrl Pts',(26.787903481163,63.761980950099,211.312499998088));
#35235=CARTESIAN_POINT('Ctrl Pts',(26.787903481163,62.8382205193956,211.254166664755));
#35236=CARTESIAN_POINT('Ctrl Pts',(25.987903481163,62.3763403040439,211.195833331421));
#35237=CARTESIAN_POINT('Ctrl Pts',(25.187903481163,61.9144600886922,211.137499998088));
#35238=CARTESIAN_POINT('Ctrl Pts',(24.387903481163,62.3763403040439,211.079166664755));
#35239=CARTESIAN_POINT('Ctrl Pts',(23.587903481163,62.8382205193956,211.020833331422));
#35240=CARTESIAN_POINT('Ctrl Pts',(23.587903481163,63.761980950099,210.962499998088));
#35241=CARTESIAN_POINT('Ctrl Pts',(23.587903481163,64.6857413808024,210.904166664755));
#35242=CARTESIAN_POINT('Ctrl Pts',(24.387903481163,65.1476215961541,210.845833331421));
#35243=CARTESIAN_POINT('Ctrl Pts',(25.187903481163,65.6095018115058,210.787499998088));
#35244=CARTESIAN_POINT('Ctrl Pts',(25.987903481163,65.1476215961541,210.729166664755));
#35245=CARTESIAN_POINT('Ctrl Pts',(26.787903481163,64.6857413808024,210.670833331422));
#35246=CARTESIAN_POINT('Ctrl Pts',(26.787903481163,63.761980950099,210.612499998088));
#35247=CARTESIAN_POINT('Ctrl Pts',(26.787903481163,62.8382205193956,210.554166664755));
#35248=CARTESIAN_POINT('Ctrl Pts',(25.987903481163,62.3763403040439,210.495833331421));
#35249=CARTESIAN_POINT('Ctrl Pts',(25.187903481163,61.9144600886922,210.437499998088));
#35250=CARTESIAN_POINT('Ctrl Pts',(24.387903481163,62.3763403040439,210.379166664755));
#35251=CARTESIAN_POINT('Ctrl Pts',(23.587903481163,62.8382205193956,210.320833331422));
#35252=CARTESIAN_POINT('Ctrl Pts',(23.587903481163,63.761980950099,210.262499998088));
#35253=CARTESIAN_POINT('Ctrl Pts',(23.587903481163,64.6857413808024,210.204166664755));
#35254=CARTESIAN_POINT('Ctrl Pts',(24.387903481163,65.1476215961541,210.145833331421));
#35255=CARTESIAN_POINT('Ctrl Pts',(25.187903481163,65.6095018115058,210.087499998088));
#35256=CARTESIAN_POINT('Ctrl Pts',(25.987903481163,65.1476215961541,210.029166664755));
#35257=CARTESIAN_POINT('Ctrl Pts',(26.787903481163,64.6857413808024,209.970833331421));
#35258=CARTESIAN_POINT('Ctrl Pts',(26.787903481163,63.761980950099,209.912499998088));
#35259=CARTESIAN_POINT('Ctrl Pts',(26.787903481163,62.8382205193956,209.854166664755));
#35260=CARTESIAN_POINT('Ctrl Pts',(25.987903481163,62.3763403040439,209.795833331421));
#35261=CARTESIAN_POINT('Ctrl Pts',(25.187903481163,61.9144600886922,209.737499998088));
#35262=CARTESIAN_POINT('Ctrl Pts',(24.387903481163,62.3763403040439,209.679166664755));
#35263=CARTESIAN_POINT('Ctrl Pts',(23.587903481163,62.8382205193956,209.620833331422));
#35264=CARTESIAN_POINT('Ctrl Pts',(23.587903481163,63.761980950099,209.562499998088));
#35265=CARTESIAN_POINT('Ctrl Pts',(23.587903481163,64.6857413808024,209.504166664755));
#35266=CARTESIAN_POINT('Ctrl Pts',(24.387903481163,65.1476215961541,209.445833331422));
#35267=CARTESIAN_POINT('Ctrl Pts',(25.187903481163,65.6095018115058,209.387499998088));
#35268=CARTESIAN_POINT('Ctrl Pts',(25.987903481163,65.1476215961541,209.329166664755));
#35269=CARTESIAN_POINT('Ctrl Pts',(26.787903481163,64.6857413808024,209.270833331422));
#35270=CARTESIAN_POINT('Ctrl Pts',(26.787903481163,63.761980950099,209.212499998088));
#35271=CARTESIAN_POINT('Ctrl Pts',(26.787903481163,62.8382205193956,209.154166664755));
#35272=CARTESIAN_POINT('Ctrl Pts',(25.987903481163,62.3763403040439,209.095833331422));
#35273=CARTESIAN_POINT('Ctrl Pts',(25.187903481163,61.9144600886922,209.037499998088));
#35274=CARTESIAN_POINT('Ctrl Pts',(24.387903481163,62.3763403040439,208.979166664755));
#35275=CARTESIAN_POINT('Ctrl Pts',(23.587903481163,62.8382205193956,208.920833331422));
#35276=CARTESIAN_POINT('Ctrl Pts',(23.587903481163,63.761980950099,208.862499998088));
#35277=CARTESIAN_POINT('Ctrl Pts',(23.587903481163,64.6857413808024,208.804166664755));
#35278=CARTESIAN_POINT('Ctrl Pts',(24.387903481163,65.1476215961541,208.745833331422));
#35279=CARTESIAN_POINT('Ctrl Pts',(25.187903481163,65.6095018115058,208.687499998088));
#35280=CARTESIAN_POINT('Ctrl Pts',(25.987903481163,65.1476215961541,208.629166664755));
#35281=CARTESIAN_POINT('Ctrl Pts',(26.787903481163,64.6857413808024,208.570833331422));
#35282=CARTESIAN_POINT('Ctrl Pts',(26.787903481163,63.761980950099,208.512499998088));
#35283=CARTESIAN_POINT('Ctrl Pts',(26.787903481163,62.8382205193956,208.454166664755));
#35284=CARTESIAN_POINT('Ctrl Pts',(25.987903481163,62.3763403040439,208.395833331421));
#35285=CARTESIAN_POINT('Ctrl Pts',(25.187903481163,61.9144600886922,208.337499998088));
#35286=CARTESIAN_POINT('Ctrl Pts',(24.387903481163,62.3763403040439,208.279166664755));
#35287=CARTESIAN_POINT('Ctrl Pts',(23.587903481163,62.8382205193956,208.220833331421));
#35288=CARTESIAN_POINT('Ctrl Pts',(23.587903481163,63.761980950099,208.162499998088));
#35289=CARTESIAN_POINT('Ctrl Pts',(23.587903481163,64.6857413808024,208.104166664755));
#35290=CARTESIAN_POINT('Ctrl Pts',(24.387903481163,65.1476215961541,208.045833331421));
#35291=CARTESIAN_POINT('Ctrl Pts',(25.187903481163,65.6095018115058,207.987499998088));
#35292=CARTESIAN_POINT('Ctrl Pts',(25.987903481163,65.1476215961541,207.929166664755));
#35293=CARTESIAN_POINT('Ctrl Pts',(26.787903481163,64.6857413808024,207.870833331422));
#35294=CARTESIAN_POINT('Ctrl Pts',(26.787903481163,63.761980950099,207.812499998088));
#35295=CARTESIAN_POINT('Ctrl Pts',(26.787903481163,62.8382205193956,207.754166664755));
#35296=CARTESIAN_POINT('Ctrl Pts',(25.987903481163,62.3763403040439,207.695833331422));
#35297=CARTESIAN_POINT('Ctrl Pts',(25.187903481163,61.9144600886922,207.637499998088));
#35298=CARTESIAN_POINT('Ctrl Pts',(24.387903481163,62.3763403040439,207.579166664755));
#35299=CARTESIAN_POINT('Ctrl Pts',(23.587903481163,62.8382205193956,207.520833331422));
#35300=CARTESIAN_POINT('Ctrl Pts',(23.587903481163,63.761980950099,207.462499998088));
#35301=CARTESIAN_POINT('Ctrl Pts',(23.587903481163,64.6857413808024,207.404166664755));
#35302=CARTESIAN_POINT('Ctrl Pts',(24.387903481163,65.1476215961541,207.345833331422));
#35303=CARTESIAN_POINT('Ctrl Pts',(25.187903481163,65.6095018115058,207.287499998088));
#35304=CARTESIAN_POINT('Ctrl Pts',(25.987903481163,65.1476215961541,207.229166664755));
#35305=CARTESIAN_POINT('Ctrl Pts',(26.787903481163,64.6857413808024,207.170833331422));
#35306=CARTESIAN_POINT('Ctrl Pts',(26.787903481163,63.761980950099,207.112499998088));
#35307=CARTESIAN_POINT('Ctrl Pts',(26.787903481163,62.8382205193956,207.054166664755));
#35308=CARTESIAN_POINT('Ctrl Pts',(25.987903481163,62.3763403040439,206.995833331422));
#35309=CARTESIAN_POINT('Ctrl Pts',(25.187903481163,61.9144600886922,206.937499998088));
#35310=CARTESIAN_POINT('Ctrl Pts',(24.387903481163,62.3763403040439,206.879166664755));
#35311=CARTESIAN_POINT('Ctrl Pts',(23.587903481163,62.8382205193956,206.820833331422));
#35312=CARTESIAN_POINT('Ctrl Pts',(23.587903481163,63.761980950099,206.762499998088));
#35313=CARTESIAN_POINT('Ctrl Pts',(23.587903481163,64.6857413808024,206.704166664755));
#35314=CARTESIAN_POINT('Ctrl Pts',(24.387903481163,65.1476215961541,206.645833331421));
#35315=CARTESIAN_POINT('Ctrl Pts',(25.187903481163,65.6095018115058,206.587499998088));
#35316=CARTESIAN_POINT('Ctrl Pts',(25.987903481163,65.1476215961541,206.529166664755));
#35317=CARTESIAN_POINT('Ctrl Pts',(26.787903481163,64.6857413808024,206.470833331422));
#35318=CARTESIAN_POINT('Ctrl Pts',(26.787903481163,63.761980950099,206.412499998088));
#35319=CARTESIAN_POINT('Ctrl Pts',(26.787903481163,62.8382205193956,206.354166664755));
#35320=CARTESIAN_POINT('Ctrl Pts',(25.987903481163,62.3763403040439,206.295833331422));
#35321=CARTESIAN_POINT('Ctrl Pts',(25.187903481163,61.9144600886922,206.237499998088));
#35322=CARTESIAN_POINT('Ctrl Pts',(24.387903481163,62.3763403040439,206.179166664755));
#35323=CARTESIAN_POINT('Ctrl Pts',(23.587903481163,62.8382205193956,206.120833331422));
#35324=CARTESIAN_POINT('Ctrl Pts',(23.587903481163,63.761980950099,206.062499998088));
#35325=CARTESIAN_POINT('Ctrl Pts',(23.587903481163,64.6857413808024,206.004166664755));
#35326=CARTESIAN_POINT('Ctrl Pts',(24.387903481163,65.1476215961541,205.945833331422));
#35327=CARTESIAN_POINT('Ctrl Pts',(25.187903481163,65.6095018115058,205.887499998088));
#35328=CARTESIAN_POINT('Ctrl Pts',(25.987903481163,65.1476215961541,205.829166664755));
#35329=CARTESIAN_POINT('Ctrl Pts',(26.787903481163,64.6857413808024,205.770833331422));
#35330=CARTESIAN_POINT('Ctrl Pts',(26.787903481163,63.761980950099,205.712499998088));
#35331=CARTESIAN_POINT('Ctrl Pts',(26.787903481163,62.8382205193956,205.654166664755));
#35332=CARTESIAN_POINT('Ctrl Pts',(25.987903481163,62.3763403040439,205.595833331421));
#35333=CARTESIAN_POINT('Ctrl Pts',(25.187903481163,61.9144600886922,205.537499998088));
#35334=CARTESIAN_POINT('Ctrl Pts',(24.387903481163,62.3763403040439,205.479166664755));
#35335=CARTESIAN_POINT('Ctrl Pts',(23.587903481163,62.8382205193956,205.420833331422));
#35336=CARTESIAN_POINT('Ctrl Pts',(23.587903481163,63.761980950099,205.362499998088));
#35337=CARTESIAN_POINT('Ctrl Pts',(23.587903481163,64.6857413808024,205.304166664755));
#35338=CARTESIAN_POINT('Ctrl Pts',(24.387903481163,65.1476215961541,205.245833331421));
#35339=CARTESIAN_POINT('Ctrl Pts',(25.187903481163,65.6095018115058,205.187499998088));
#35340=CARTESIAN_POINT('Ctrl Pts',(25.987903481163,65.1476215961541,205.129166664755));
#35341=CARTESIAN_POINT('Ctrl Pts',(26.787903481163,64.6857413808024,205.070833331422));
#35342=CARTESIAN_POINT('Ctrl Pts',(26.787903481163,63.761980950099,205.012499998088));
#35343=CARTESIAN_POINT('Ctrl Pts',(26.787903481163,62.8382205193956,204.954166664755));
#35344=CARTESIAN_POINT('Ctrl Pts',(25.987903481163,62.3763403040439,204.895833331421));
#35345=CARTESIAN_POINT('Ctrl Pts',(25.187903481163,61.9144600886922,204.837499998088));
#35346=CARTESIAN_POINT('Ctrl Pts',(24.387903481163,62.3763403040439,204.779166664755));
#35347=CARTESIAN_POINT('Ctrl Pts',(23.587903481163,62.8382205193956,204.720833331422));
#35348=CARTESIAN_POINT('Ctrl Pts',(23.587903481163,63.761980950099,204.662499998088));
#35349=CARTESIAN_POINT('Ctrl Pts',(23.587903481163,64.6857413808024,204.604166664755));
#35350=CARTESIAN_POINT('Ctrl Pts',(24.387903481163,65.1476215961541,204.545833331422));
#35351=CARTESIAN_POINT('Ctrl Pts',(25.187903481163,65.6095018115058,204.487499998088));
#35352=CARTESIAN_POINT('Ctrl Pts',(25.987903481163,65.1476215961541,204.429166664755));
#35353=CARTESIAN_POINT('Ctrl Pts',(26.787903481163,64.6857413808024,204.370833331422));
#35354=CARTESIAN_POINT('Ctrl Pts',(26.787903481163,63.761980950099,204.312499998088));
#35355=CARTESIAN_POINT('Ctrl Pts',(26.787903481163,62.8382205193956,204.254166664755));
#35356=CARTESIAN_POINT('Ctrl Pts',(25.987903481163,62.3763403040439,204.195833331422));
#35357=CARTESIAN_POINT('Ctrl Pts',(25.187903481163,61.9144600886922,204.137499998088));
#35358=CARTESIAN_POINT('Ctrl Pts',(24.387903481163,62.3763403040439,204.079166664755));
#35359=CARTESIAN_POINT('Ctrl Pts',(23.587903481163,62.8382205193956,204.020833331421));
#35360=CARTESIAN_POINT('Ctrl Pts',(23.587903481163,63.761980950099,203.962499998088));
#35361=CARTESIAN_POINT('Ctrl Pts',(23.587903481163,64.6857413808024,203.904166664755));
#35362=CARTESIAN_POINT('Ctrl Pts',(24.387903481163,65.1476215961541,203.845833331421));
#35363=CARTESIAN_POINT('Ctrl Pts',(25.187903481163,65.6095018115058,203.787499998088));
#35364=CARTESIAN_POINT('Ctrl Pts',(25.987903481163,65.1476215961541,203.729166664755));
#35365=CARTESIAN_POINT('Ctrl Pts',(26.787903481163,64.6857413808024,203.670833331421));
#35366=CARTESIAN_POINT('Ctrl Pts',(26.787903481163,63.761980950099,203.612499998088));
#35367=CARTESIAN_POINT('Ctrl Pts',(26.787903481163,62.8382205193956,203.554166664755));
#35368=CARTESIAN_POINT('Ctrl Pts',(25.987903481163,62.3763403040439,203.495833331421));
#35369=CARTESIAN_POINT('Ctrl Pts',(25.187903481163,61.9144600886922,203.437499998088));
#35370=CARTESIAN_POINT('Ctrl Pts',(24.387903481163,62.3763403040439,203.379166664755));
#35371=CARTESIAN_POINT('Ctrl Pts',(23.587903481163,62.8382205193956,203.320833331422));
#35372=CARTESIAN_POINT('Ctrl Pts',(23.587903481163,63.761980950099,203.262499998088));
#35373=CARTESIAN_POINT('Ctrl Pts',(23.587903481163,64.6857413808024,203.204166664755));
#35374=CARTESIAN_POINT('Ctrl Pts',(24.387903481163,65.1476215961541,203.145833331421));
#35375=CARTESIAN_POINT('Ctrl Pts',(25.187903481163,65.6095018115058,203.087499998088));
#35376=CARTESIAN_POINT('Ctrl Pts',(25.987903481163,65.1476215961541,203.029166664755));
#35377=CARTESIAN_POINT('Ctrl Pts',(26.787903481163,64.6857413808024,202.970833331422));
#35378=CARTESIAN_POINT('Ctrl Pts',(26.787903481163,63.761980950099,202.912499998088));
#35379=CARTESIAN_POINT('Ctrl Pts',(26.409017368663,63.761980950099,212.493749999044));
#35380=CARTESIAN_POINT('Ctrl Pts',(26.409017368663,63.0569705184397,212.435416665711));
#35381=CARTESIAN_POINT('Ctrl Pts',(25.798460424913,62.70446530261,212.377083332377));
#35382=CARTESIAN_POINT('Ctrl Pts',(25.187903481163,62.3519600867804,212.318749999044));
#35383=CARTESIAN_POINT('Ctrl Pts',(24.577346537413,62.70446530261,212.260416665711));
#35384=CARTESIAN_POINT('Ctrl Pts',(23.966789593663,63.0569705184397,212.202083332377));
#35385=CARTESIAN_POINT('Ctrl Pts',(23.966789593663,63.761980950099,212.143749999044));
#35386=CARTESIAN_POINT('Ctrl Pts',(23.966789593663,64.4669913817583,212.085416665711));
#35387=CARTESIAN_POINT('Ctrl Pts',(24.577346537413,64.819496597588,212.027083332377));
#35388=CARTESIAN_POINT('Ctrl Pts',(25.187903481163,65.1720018134176,211.968749999044));
#35389=CARTESIAN_POINT('Ctrl Pts',(25.798460424913,64.819496597588,211.910416665711));
#35390=CARTESIAN_POINT('Ctrl Pts',(26.409017368663,64.4669913817583,211.852083332377));
#35391=CARTESIAN_POINT('Ctrl Pts',(26.409017368663,63.761980950099,211.793749999044));
#35392=CARTESIAN_POINT('Ctrl Pts',(26.409017368663,63.0569705184397,211.735416665711));
#35393=CARTESIAN_POINT('Ctrl Pts',(25.798460424913,62.70446530261,211.677083332377));
#35394=CARTESIAN_POINT('Ctrl Pts',(25.187903481163,62.3519600867804,211.618749999044));
#35395=CARTESIAN_POINT('Ctrl Pts',(24.577346537413,62.70446530261,211.560416665711));
#35396=CARTESIAN_POINT('Ctrl Pts',(23.966789593663,63.0569705184397,211.502083332377));
#35397=CARTESIAN_POINT('Ctrl Pts',(23.966789593663,63.761980950099,211.443749999044));
#35398=CARTESIAN_POINT('Ctrl Pts',(23.966789593663,64.4669913817583,211.385416665711));
#35399=CARTESIAN_POINT('Ctrl Pts',(24.577346537413,64.819496597588,211.327083332377));
#35400=CARTESIAN_POINT('Ctrl Pts',(25.187903481163,65.1720018134176,211.268749999044));
#35401=CARTESIAN_POINT('Ctrl Pts',(25.798460424913,64.819496597588,211.210416665711));
#35402=CARTESIAN_POINT('Ctrl Pts',(26.409017368663,64.4669913817583,211.152083332377));
#35403=CARTESIAN_POINT('Ctrl Pts',(26.409017368663,63.761980950099,211.093749999044));
#35404=CARTESIAN_POINT('Ctrl Pts',(26.409017368663,63.0569705184397,211.035416665711));
#35405=CARTESIAN_POINT('Ctrl Pts',(25.798460424913,62.70446530261,210.977083332377));
#35406=CARTESIAN_POINT('Ctrl Pts',(25.187903481163,62.3519600867804,210.918749999044));
#35407=CARTESIAN_POINT('Ctrl Pts',(24.577346537413,62.70446530261,210.860416665711));
#35408=CARTESIAN_POINT('Ctrl Pts',(23.966789593663,63.0569705184397,210.802083332377));
#35409=CARTESIAN_POINT('Ctrl Pts',(23.966789593663,63.761980950099,210.743749999044));
#35410=CARTESIAN_POINT('Ctrl Pts',(23.966789593663,64.4669913817583,210.685416665711));
#35411=CARTESIAN_POINT('Ctrl Pts',(24.577346537413,64.819496597588,210.627083332377));
#35412=CARTESIAN_POINT('Ctrl Pts',(25.187903481163,65.1720018134176,210.568749999044));
#35413=CARTESIAN_POINT('Ctrl Pts',(25.798460424913,64.819496597588,210.510416665711));
#35414=CARTESIAN_POINT('Ctrl Pts',(26.409017368663,64.4669913817583,210.452083332377));
#35415=CARTESIAN_POINT('Ctrl Pts',(26.409017368663,63.761980950099,210.393749999044));
#35416=CARTESIAN_POINT('Ctrl Pts',(26.409017368663,63.0569705184397,210.335416665711));
#35417=CARTESIAN_POINT('Ctrl Pts',(25.798460424913,62.70446530261,210.277083332377));
#35418=CARTESIAN_POINT('Ctrl Pts',(25.187903481163,62.3519600867804,210.218749999044));
#35419=CARTESIAN_POINT('Ctrl Pts',(24.577346537413,62.70446530261,210.160416665711));
#35420=CARTESIAN_POINT('Ctrl Pts',(23.966789593663,63.0569705184397,210.102083332377));
#35421=CARTESIAN_POINT('Ctrl Pts',(23.966789593663,63.761980950099,210.043749999044));
#35422=CARTESIAN_POINT('Ctrl Pts',(23.966789593663,64.4669913817583,209.985416665711));
#35423=CARTESIAN_POINT('Ctrl Pts',(24.577346537413,64.819496597588,209.927083332377));
#35424=CARTESIAN_POINT('Ctrl Pts',(25.187903481163,65.1720018134176,209.868749999044));
#35425=CARTESIAN_POINT('Ctrl Pts',(25.798460424913,64.819496597588,209.810416665711));
#35426=CARTESIAN_POINT('Ctrl Pts',(26.409017368663,64.4669913817583,209.752083332377));
#35427=CARTESIAN_POINT('Ctrl Pts',(26.409017368663,63.761980950099,209.693749999044));
#35428=CARTESIAN_POINT('Ctrl Pts',(26.409017368663,63.0569705184397,209.635416665711));
#35429=CARTESIAN_POINT('Ctrl Pts',(25.798460424913,62.70446530261,209.577083332377));
#35430=CARTESIAN_POINT('Ctrl Pts',(25.187903481163,62.3519600867804,209.518749999044));
#35431=CARTESIAN_POINT('Ctrl Pts',(24.577346537413,62.70446530261,209.460416665711));
#35432=CARTESIAN_POINT('Ctrl Pts',(23.966789593663,63.0569705184397,209.402083332377));
#35433=CARTESIAN_POINT('Ctrl Pts',(23.966789593663,63.761980950099,209.343749999044));
#35434=CARTESIAN_POINT('Ctrl Pts',(23.966789593663,64.4669913817583,209.285416665711));
#35435=CARTESIAN_POINT('Ctrl Pts',(24.577346537413,64.819496597588,209.227083332377));
#35436=CARTESIAN_POINT('Ctrl Pts',(25.187903481163,65.1720018134176,209.168749999044));
#35437=CARTESIAN_POINT('Ctrl Pts',(25.798460424913,64.819496597588,209.110416665711));
#35438=CARTESIAN_POINT('Ctrl Pts',(26.409017368663,64.4669913817583,209.052083332377));
#35439=CARTESIAN_POINT('Ctrl Pts',(26.409017368663,63.761980950099,208.993749999044));
#35440=CARTESIAN_POINT('Ctrl Pts',(26.409017368663,63.0569705184397,208.935416665711));
#35441=CARTESIAN_POINT('Ctrl Pts',(25.798460424913,62.70446530261,208.877083332377));
#35442=CARTESIAN_POINT('Ctrl Pts',(25.187903481163,62.3519600867804,208.818749999044));
#35443=CARTESIAN_POINT('Ctrl Pts',(24.577346537413,62.70446530261,208.760416665711));
#35444=CARTESIAN_POINT('Ctrl Pts',(23.966789593663,63.0569705184397,208.702083332377));
#35445=CARTESIAN_POINT('Ctrl Pts',(23.966789593663,63.761980950099,208.643749999044));
#35446=CARTESIAN_POINT('Ctrl Pts',(23.966789593663,64.4669913817583,208.585416665711));
#35447=CARTESIAN_POINT('Ctrl Pts',(24.577346537413,64.819496597588,208.527083332377));
#35448=CARTESIAN_POINT('Ctrl Pts',(25.187903481163,65.1720018134176,208.468749999044));
#35449=CARTESIAN_POINT('Ctrl Pts',(25.798460424913,64.819496597588,208.410416665711));
#35450=CARTESIAN_POINT('Ctrl Pts',(26.409017368663,64.4669913817583,208.352083332377));
#35451=CARTESIAN_POINT('Ctrl Pts',(26.409017368663,63.761980950099,208.293749999044));
#35452=CARTESIAN_POINT('Ctrl Pts',(26.409017368663,63.0569705184397,208.235416665711));
#35453=CARTESIAN_POINT('Ctrl Pts',(25.798460424913,62.70446530261,208.177083332377));
#35454=CARTESIAN_POINT('Ctrl Pts',(25.187903481163,62.3519600867804,208.118749999044));
#35455=CARTESIAN_POINT('Ctrl Pts',(24.577346537413,62.70446530261,208.060416665711));
#35456=CARTESIAN_POINT('Ctrl Pts',(23.966789593663,63.0569705184397,208.002083332377));
#35457=CARTESIAN_POINT('Ctrl Pts',(23.966789593663,63.761980950099,207.943749999044));
#35458=CARTESIAN_POINT('Ctrl Pts',(23.966789593663,64.4669913817583,207.885416665711));
#35459=CARTESIAN_POINT('Ctrl Pts',(24.577346537413,64.819496597588,207.827083332377));
#35460=CARTESIAN_POINT('Ctrl Pts',(25.187903481163,65.1720018134176,207.768749999044));
#35461=CARTESIAN_POINT('Ctrl Pts',(25.798460424913,64.819496597588,207.710416665711));
#35462=CARTESIAN_POINT('Ctrl Pts',(26.409017368663,64.4669913817583,207.652083332377));
#35463=CARTESIAN_POINT('Ctrl Pts',(26.409017368663,63.761980950099,207.593749999044));
#35464=CARTESIAN_POINT('Ctrl Pts',(26.409017368663,63.0569705184397,207.535416665711));
#35465=CARTESIAN_POINT('Ctrl Pts',(25.798460424913,62.70446530261,207.477083332377));
#35466=CARTESIAN_POINT('Ctrl Pts',(25.187903481163,62.3519600867804,207.418749999044));
#35467=CARTESIAN_POINT('Ctrl Pts',(24.577346537413,62.70446530261,207.360416665711));
#35468=CARTESIAN_POINT('Ctrl Pts',(23.966789593663,63.0569705184397,207.302083332377));
#35469=CARTESIAN_POINT('Ctrl Pts',(23.966789593663,63.761980950099,207.243749999044));
#35470=CARTESIAN_POINT('Ctrl Pts',(23.966789593663,64.4669913817583,207.185416665711));
#35471=CARTESIAN_POINT('Ctrl Pts',(24.577346537413,64.819496597588,207.127083332377));
#35472=CARTESIAN_POINT('Ctrl Pts',(25.187903481163,65.1720018134176,207.068749999044));
#35473=CARTESIAN_POINT('Ctrl Pts',(25.798460424913,64.819496597588,207.010416665711));
#35474=CARTESIAN_POINT('Ctrl Pts',(26.409017368663,64.4669913817583,206.952083332377));
#35475=CARTESIAN_POINT('Ctrl Pts',(26.409017368663,63.761980950099,206.893749999044));
#35476=CARTESIAN_POINT('Ctrl Pts',(26.409017368663,63.0569705184397,206.835416665711));
#35477=CARTESIAN_POINT('Ctrl Pts',(25.798460424913,62.70446530261,206.777083332377));
#35478=CARTESIAN_POINT('Ctrl Pts',(25.187903481163,62.3519600867804,206.718749999044));
#35479=CARTESIAN_POINT('Ctrl Pts',(24.577346537413,62.70446530261,206.660416665711));
#35480=CARTESIAN_POINT('Ctrl Pts',(23.966789593663,63.0569705184397,206.602083332377));
#35481=CARTESIAN_POINT('Ctrl Pts',(23.966789593663,63.761980950099,206.543749999044));
#35482=CARTESIAN_POINT('Ctrl Pts',(23.966789593663,64.4669913817583,206.485416665711));
#35483=CARTESIAN_POINT('Ctrl Pts',(24.577346537413,64.819496597588,206.427083332377));
#35484=CARTESIAN_POINT('Ctrl Pts',(25.187903481163,65.1720018134176,206.368749999044));
#35485=CARTESIAN_POINT('Ctrl Pts',(25.798460424913,64.819496597588,206.310416665711));
#35486=CARTESIAN_POINT('Ctrl Pts',(26.409017368663,64.4669913817583,206.252083332377));
#35487=CARTESIAN_POINT('Ctrl Pts',(26.409017368663,63.761980950099,206.193749999044));
#35488=CARTESIAN_POINT('Ctrl Pts',(26.409017368663,63.0569705184397,206.135416665711));
#35489=CARTESIAN_POINT('Ctrl Pts',(25.798460424913,62.70446530261,206.077083332377));
#35490=CARTESIAN_POINT('Ctrl Pts',(25.187903481163,62.3519600867804,206.018749999044));
#35491=CARTESIAN_POINT('Ctrl Pts',(24.577346537413,62.70446530261,205.960416665711));
#35492=CARTESIAN_POINT('Ctrl Pts',(23.966789593663,63.0569705184397,205.902083332377));
#35493=CARTESIAN_POINT('Ctrl Pts',(23.966789593663,63.761980950099,205.843749999044));
#35494=CARTESIAN_POINT('Ctrl Pts',(23.966789593663,64.4669913817583,205.785416665711));
#35495=CARTESIAN_POINT('Ctrl Pts',(24.577346537413,64.819496597588,205.727083332377));
#35496=CARTESIAN_POINT('Ctrl Pts',(25.187903481163,65.1720018134176,205.668749999044));
#35497=CARTESIAN_POINT('Ctrl Pts',(25.798460424913,64.819496597588,205.610416665711));
#35498=CARTESIAN_POINT('Ctrl Pts',(26.409017368663,64.4669913817583,205.552083332377));
#35499=CARTESIAN_POINT('Ctrl Pts',(26.409017368663,63.761980950099,205.493749999044));
#35500=CARTESIAN_POINT('Ctrl Pts',(26.409017368663,63.0569705184397,205.435416665711));
#35501=CARTESIAN_POINT('Ctrl Pts',(25.798460424913,62.70446530261,205.377083332377));
#35502=CARTESIAN_POINT('Ctrl Pts',(25.187903481163,62.3519600867804,205.318749999044));
#35503=CARTESIAN_POINT('Ctrl Pts',(24.577346537413,62.70446530261,205.260416665711));
#35504=CARTESIAN_POINT('Ctrl Pts',(23.966789593663,63.0569705184397,205.202083332377));
#35505=CARTESIAN_POINT('Ctrl Pts',(23.966789593663,63.761980950099,205.143749999044));
#35506=CARTESIAN_POINT('Ctrl Pts',(23.966789593663,64.4669913817583,205.085416665711));
#35507=CARTESIAN_POINT('Ctrl Pts',(24.577346537413,64.819496597588,205.027083332377));
#35508=CARTESIAN_POINT('Ctrl Pts',(25.187903481163,65.1720018134176,204.968749999044));
#35509=CARTESIAN_POINT('Ctrl Pts',(25.798460424913,64.819496597588,204.910416665711));
#35510=CARTESIAN_POINT('Ctrl Pts',(26.409017368663,64.4669913817583,204.852083332377));
#35511=CARTESIAN_POINT('Ctrl Pts',(26.409017368663,63.761980950099,204.793749999044));
#35512=CARTESIAN_POINT('Ctrl Pts',(26.409017368663,63.0569705184397,204.735416665711));
#35513=CARTESIAN_POINT('Ctrl Pts',(25.798460424913,62.70446530261,204.677083332377));
#35514=CARTESIAN_POINT('Ctrl Pts',(25.187903481163,62.3519600867804,204.618749999044));
#35515=CARTESIAN_POINT('Ctrl Pts',(24.577346537413,62.70446530261,204.560416665711));
#35516=CARTESIAN_POINT('Ctrl Pts',(23.966789593663,63.0569705184397,204.502083332377));
#35517=CARTESIAN_POINT('Ctrl Pts',(23.966789593663,63.761980950099,204.443749999044));
#35518=CARTESIAN_POINT('Ctrl Pts',(23.966789593663,64.4669913817583,204.385416665711));
#35519=CARTESIAN_POINT('Ctrl Pts',(24.577346537413,64.819496597588,204.327083332377));
#35520=CARTESIAN_POINT('Ctrl Pts',(25.187903481163,65.1720018134176,204.268749999044));
#35521=CARTESIAN_POINT('Ctrl Pts',(25.798460424913,64.819496597588,204.210416665711));
#35522=CARTESIAN_POINT('Ctrl Pts',(26.409017368663,64.4669913817583,204.152083332377));
#35523=CARTESIAN_POINT('Ctrl Pts',(26.409017368663,63.761980950099,204.093749999044));
#35524=CARTESIAN_POINT('Ctrl Pts',(26.409017368663,63.0569705184397,204.035416665711));
#35525=CARTESIAN_POINT('Ctrl Pts',(25.798460424913,62.70446530261,203.977083332377));
#35526=CARTESIAN_POINT('Ctrl Pts',(25.187903481163,62.3519600867804,203.918749999044));
#35527=CARTESIAN_POINT('Ctrl Pts',(24.577346537413,62.70446530261,203.860416665711));
#35528=CARTESIAN_POINT('Ctrl Pts',(23.966789593663,63.0569705184397,203.802083332377));
#35529=CARTESIAN_POINT('Ctrl Pts',(23.966789593663,63.761980950099,203.743749999044));
#35530=CARTESIAN_POINT('Ctrl Pts',(23.966789593663,64.4669913817583,203.685416665711));
#35531=CARTESIAN_POINT('Ctrl Pts',(24.577346537413,64.819496597588,203.627083332377));
#35532=CARTESIAN_POINT('Ctrl Pts',(25.187903481163,65.1720018134176,203.568749999044));
#35533=CARTESIAN_POINT('Ctrl Pts',(25.798460424913,64.819496597588,203.510416665711));
#35534=CARTESIAN_POINT('Ctrl Pts',(26.409017368663,64.4669913817583,203.452083332377));
#35535=CARTESIAN_POINT('Ctrl Pts',(26.409017368663,63.761980950099,203.393749999044));
#35536=CARTESIAN_POINT('Ctrl Pts',(26.409017368663,63.0569705184397,203.335416665711));
#35537=CARTESIAN_POINT('Ctrl Pts',(25.798460424913,62.70446530261,203.277083332377));
#35538=CARTESIAN_POINT('Ctrl Pts',(25.187903481163,62.3519600867804,203.218749999044));
#35539=CARTESIAN_POINT('Ctrl Pts',(24.577346537413,62.70446530261,203.160416665711));
#35540=CARTESIAN_POINT('Ctrl Pts',(23.966789593663,63.0569705184397,203.102083332377));
#35541=CARTESIAN_POINT('Ctrl Pts',(23.966789593663,63.761980950099,203.043749999044));
#35542=CARTESIAN_POINT('Ctrl Pts',(23.966789593663,64.4669913817583,202.985416665711));
#35543=CARTESIAN_POINT('Ctrl Pts',(24.577346537413,64.819496597588,202.927083332377));
#35544=CARTESIAN_POINT('Ctrl Pts',(25.187903481163,65.1720018134176,202.868749999044));
#35545=CARTESIAN_POINT('Ctrl Pts',(25.798460424913,64.819496597588,202.810416665711));
#35546=CARTESIAN_POINT('Ctrl Pts',(26.409017368663,64.4669913817583,202.752083332377));
#35547=CARTESIAN_POINT('Ctrl Pts',(26.409017368663,63.761980950099,202.693749999044));
#35548=CARTESIAN_POINT('',(26.598460424913,63.761980950099,212.603124998566));
#35549=CARTESIAN_POINT('Ctrl Pts',(23.966789593663,63.761980950099,212.143749999044));
#35550=CARTESIAN_POINT('Ctrl Pts',(23.966789593663,64.4669913817583,212.085416665711));
#35551=CARTESIAN_POINT('Ctrl Pts',(24.577346537413,64.819496597588,212.027083332377));
#35552=CARTESIAN_POINT('Ctrl Pts',(25.187903481163,65.1720018134176,211.968749999044));
#35553=CARTESIAN_POINT('Ctrl Pts',(25.798460424913,64.819496597588,211.910416665711));
#35554=CARTESIAN_POINT('Ctrl Pts',(26.409017368663,64.4669913817583,211.852083332377));
#35555=CARTESIAN_POINT('Ctrl Pts',(26.409017368663,63.761980950099,211.793749999044));
#35556=CARTESIAN_POINT('Ctrl Pts',(26.409017368663,63.0569705184397,211.735416665711));
#35557=CARTESIAN_POINT('Ctrl Pts',(25.798460424913,62.70446530261,211.677083332377));
#35558=CARTESIAN_POINT('Ctrl Pts',(25.187903481163,62.3519600867804,211.618749999044));
#35559=CARTESIAN_POINT('Ctrl Pts',(24.577346537413,62.70446530261,211.560416665711));
#35560=CARTESIAN_POINT('Ctrl Pts',(23.966789593663,63.0569705184397,211.502083332377));
#35561=CARTESIAN_POINT('Ctrl Pts',(23.966789593663,63.761980950099,211.443749999044));
#35562=CARTESIAN_POINT('',(26.598460424913,63.761980950099,202.803124998566));
#35563=CARTESIAN_POINT('Ctrl Pts',(26.787903481163,63.761980950099,211.312499998088));
#35564=CARTESIAN_POINT('Ctrl Pts',(26.787903481163,63.8741171554749,211.31958113994));
#35565=CARTESIAN_POINT('Ctrl Pts',(26.7761195543677,63.9861700545367,211.327086643522));
#35566=CARTESIAN_POINT('Ctrl Pts',(26.7081426976078,64.3042786309023,211.349652786821));
#35567=CARTESIAN_POINT('Ctrl Pts',(26.6227037454562,64.5012658582677,211.365207036137));
#35568=CARTESIAN_POINT('Ctrl Pts',(26.3844510384125,64.8437047737,211.395517557749));
#35569=CARTESIAN_POINT('Ctrl Pts',(26.2364517101797,64.9877218095493,211.410007709105));
#35570=CARTESIAN_POINT('Ctrl Pts',(25.8878489096898,65.2163196275864,211.43715260937));
#35571=CARTESIAN_POINT('Ctrl Pts',(25.6889946080725,65.2962516439341,211.450962103418));
#35572=CARTESIAN_POINT('Ctrl Pts',(25.2738293345874,65.3734083731304,211.481234571276));
#35573=CARTESIAN_POINT('Ctrl Pts',(25.0618583522795,65.3707681781366,211.496690788736));
#35574=CARTESIAN_POINT('Ctrl Pts',(24.658014157987,65.2852538654097,211.526137761236));
#35575=CARTESIAN_POINT('Ctrl Pts',(24.4694561743753,65.2059105467147,211.539179243819));
#35576=CARTESIAN_POINT('Ctrl Pts',(24.1240235923046,64.9757575818482,211.566306767127));
#35577=CARTESIAN_POINT('Ctrl Pts',(23.9725451147546,64.8240328301937,211.581410486883));
#35578=CARTESIAN_POINT('Ctrl Pts',(23.7403019497449,64.4743774588544,211.611957613098));
#35579=CARTESIAN_POINT('Ctrl Pts',(23.6601932823326,64.2808084410836,211.627101677091));
#35580=CARTESIAN_POINT('Ctrl Pts',(23.5789696508475,63.8767726017523,211.655576883513));
#35581=CARTESIAN_POINT('Ctrl Pts',(23.5774814489119,63.6704113360506,211.667902437369));
#35582=CARTESIAN_POINT('Ctrl Pts',(23.6538984231461,63.259704709123,211.696623645877));
#35583=CARTESIAN_POINT('Ctrl Pts',(23.7343932347138,63.0600292555202,211.712167395334));
#35584=CARTESIAN_POINT('Ctrl Pts',(23.9644062950721,62.7107366852901,211.742610305599));
#35585=CARTESIAN_POINT('Ctrl Pts',(24.1091112487229,62.5626871708893,211.757234991236));
#35586=CARTESIAN_POINT('Ctrl Pts',(24.4509406583139,62.326305836117,211.784624456026));
#35587=CARTESIAN_POINT('Ctrl Pts',(24.6459233339367,62.241925135792,211.797980612353));
#35588=CARTESIAN_POINT('Ctrl Pts',(25.0575582231217,62.1534622407589,211.827995656356));
#35589=CARTESIAN_POINT('Ctrl Pts',(25.2701052598562,62.1502853772832,211.843493877785));
#35590=CARTESIAN_POINT('Ctrl Pts',(25.6768194963091,62.2250449198287,211.873150124193));
#35591=CARTESIAN_POINT('Ctrl Pts',(25.8675789383445,62.2993855707684,211.886586985822));
#35592=CARTESIAN_POINT('Ctrl Pts',(26.2190795897561,62.5203062212873,211.91335274154));
#35593=CARTESIAN_POINT('Ctrl Pts',(26.3745177920632,62.6679156807696,211.928340955085));
#35594=CARTESIAN_POINT('Ctrl Pts',(26.6162914621394,63.0116546221704,211.958861938772));
#35595=CARTESIAN_POINT('Ctrl Pts',(26.7016619877479,63.2035596364255,211.974092763374));
#35596=CARTESIAN_POINT('Ctrl Pts',(26.7745478971648,63.523360725262,211.996944760797));
#35597=CARTESIAN_POINT('Ctrl Pts',(26.787903481163,63.6425978678265,212.004961232732));
#35598=CARTESIAN_POINT('Ctrl Pts',(26.787903481163,63.7619809500991,212.012499998088));
#35599=CARTESIAN_POINT('Origin',(25.1879034811629,63.761980950099,212.406249999044));
#35600=CARTESIAN_POINT('Ctrl Pts',(23.966789593663,63.761980950099,211.968749999044));
#35601=CARTESIAN_POINT('Ctrl Pts',(23.966789593663,64.4669913817583,211.910416665711));
#35602=CARTESIAN_POINT('Ctrl Pts',(24.577346537413,64.819496597588,211.852083332377));
#35603=CARTESIAN_POINT('Ctrl Pts',(25.187903481163,65.1720018134176,211.793749999044));
#35604=CARTESIAN_POINT('Ctrl Pts',(25.798460424913,64.819496597588,211.735416665711));
#35605=CARTESIAN_POINT('Ctrl Pts',(26.409017368663,64.4669913817583,211.677083332377));
#35606=CARTESIAN_POINT('Ctrl Pts',(26.409017368663,63.761980950099,211.618749999044));
#35607=CARTESIAN_POINT('Ctrl Pts',(26.409017368663,63.0569705184397,211.560416665711));
#35608=CARTESIAN_POINT('Ctrl Pts',(25.798460424913,62.70446530261,211.502083332377));
#35609=CARTESIAN_POINT('Ctrl Pts',(25.187903481163,62.3519600867804,211.443749999044));
#35610=CARTESIAN_POINT('Ctrl Pts',(24.577346537413,62.70446530261,211.385416665711));
#35611=CARTESIAN_POINT('Ctrl Pts',(23.966789593663,63.0569705184397,211.327083332377));
#35612=CARTESIAN_POINT('Ctrl Pts',(23.966789593663,63.761980950099,211.268749999044));
#35613=CARTESIAN_POINT('Ctrl Pts',(26.409017368663,63.761980950099,212.318749999044));
#35614=CARTESIAN_POINT('Ctrl Pts',(26.409017368663,63.0569705184397,212.260416665711));
#35615=CARTESIAN_POINT('Ctrl Pts',(25.798460424913,62.70446530261,212.202083332377));
#35616=CARTESIAN_POINT('Ctrl Pts',(25.187903481163,62.3519600867804,212.143749999044));
#35617=CARTESIAN_POINT('Ctrl Pts',(24.577346537413,62.70446530261,212.085416665711));
#35618=CARTESIAN_POINT('Ctrl Pts',(23.966789593663,63.0569705184397,212.027083332377));
#35619=CARTESIAN_POINT('Ctrl Pts',(23.966789593663,63.761980950099,211.968749999044));
#35620=CARTESIAN_POINT('Ctrl Pts',(23.966789593663,64.4669913817583,211.910416665711));
#35621=CARTESIAN_POINT('Ctrl Pts',(24.577346537413,64.819496597588,211.852083332377));
#35622=CARTESIAN_POINT('Ctrl Pts',(25.187903481163,65.1720018134176,211.793749999044));
#35623=CARTESIAN_POINT('Ctrl Pts',(25.798460424913,64.819496597588,211.735416665711));
#35624=CARTESIAN_POINT('Ctrl Pts',(26.409017368663,64.4669913817583,211.677083332377));
#35625=CARTESIAN_POINT('Ctrl Pts',(26.409017368663,63.761980950099,211.618749999044));
#35626=CARTESIAN_POINT('Ctrl Pts',(26.409017368663,63.0569705184397,211.560416665711));
#35627=CARTESIAN_POINT('Ctrl Pts',(25.798460424913,62.70446530261,211.502083332377));
#35628=CARTESIAN_POINT('Ctrl Pts',(25.187903481163,62.3519600867804,211.443749999044));
#35629=CARTESIAN_POINT('Ctrl Pts',(24.577346537413,62.70446530261,211.385416665711));
#35630=CARTESIAN_POINT('Ctrl Pts',(23.966789593663,63.0569705184397,211.327083332377));
#35631=CARTESIAN_POINT('Ctrl Pts',(23.966789593663,63.761980950099,211.268749999044));
#35632=CARTESIAN_POINT('Ctrl Pts',(23.966789593663,64.4669913817583,211.210416665711));
#35633=CARTESIAN_POINT('Ctrl Pts',(24.577346537413,64.819496597588,211.152083332377));
#35634=CARTESIAN_POINT('Ctrl Pts',(25.187903481163,65.1720018134176,211.093749999044));
#35635=CARTESIAN_POINT('Ctrl Pts',(25.798460424913,64.819496597588,211.035416665711));
#35636=CARTESIAN_POINT('Ctrl Pts',(26.409017368663,64.4669913817583,210.977083332377));
#35637=CARTESIAN_POINT('Ctrl Pts',(26.409017368663,63.761980950099,210.918749999044));
#35638=CARTESIAN_POINT('Ctrl Pts',(26.409017368663,63.0569705184397,210.860416665711));
#35639=CARTESIAN_POINT('Ctrl Pts',(25.798460424913,62.70446530261,210.802083332377));
#35640=CARTESIAN_POINT('Ctrl Pts',(25.187903481163,62.3519600867804,210.743749999044));
#35641=CARTESIAN_POINT('Ctrl Pts',(24.577346537413,62.70446530261,210.685416665711));
#35642=CARTESIAN_POINT('Ctrl Pts',(23.966789593663,63.0569705184397,210.627083332377));
#35643=CARTESIAN_POINT('Ctrl Pts',(23.966789593663,63.761980950099,210.568749999044));
#35644=CARTESIAN_POINT('Ctrl Pts',(23.966789593663,64.4669913817583,210.510416665711));
#35645=CARTESIAN_POINT('Ctrl Pts',(24.577346537413,64.819496597588,210.452083332377));
#35646=CARTESIAN_POINT('Ctrl Pts',(25.187903481163,65.1720018134176,210.393749999044));
#35647=CARTESIAN_POINT('Ctrl Pts',(25.798460424913,64.819496597588,210.335416665711));
#35648=CARTESIAN_POINT('Ctrl Pts',(26.409017368663,64.4669913817583,210.277083332377));
#35649=CARTESIAN_POINT('Ctrl Pts',(26.409017368663,63.761980950099,210.218749999044));
#35650=CARTESIAN_POINT('Ctrl Pts',(26.409017368663,63.0569705184397,210.160416665711));
#35651=CARTESIAN_POINT('Ctrl Pts',(25.798460424913,62.70446530261,210.102083332377));
#35652=CARTESIAN_POINT('Ctrl Pts',(25.187903481163,62.3519600867804,210.043749999044));
#35653=CARTESIAN_POINT('Ctrl Pts',(24.577346537413,62.70446530261,209.985416665711));
#35654=CARTESIAN_POINT('Ctrl Pts',(23.966789593663,63.0569705184397,209.927083332377));
#35655=CARTESIAN_POINT('Ctrl Pts',(23.966789593663,63.761980950099,209.868749999044));
#35656=CARTESIAN_POINT('Ctrl Pts',(23.966789593663,64.4669913817583,209.810416665711));
#35657=CARTESIAN_POINT('Ctrl Pts',(24.577346537413,64.819496597588,209.752083332377));
#35658=CARTESIAN_POINT('Ctrl Pts',(25.187903481163,65.1720018134176,209.693749999044));
#35659=CARTESIAN_POINT('Ctrl Pts',(25.798460424913,64.819496597588,209.635416665711));
#35660=CARTESIAN_POINT('Ctrl Pts',(26.409017368663,64.4669913817583,209.577083332377));
#35661=CARTESIAN_POINT('Ctrl Pts',(26.409017368663,63.761980950099,209.518749999044));
#35662=CARTESIAN_POINT('Ctrl Pts',(26.409017368663,63.0569705184397,209.460416665711));
#35663=CARTESIAN_POINT('Ctrl Pts',(25.798460424913,62.70446530261,209.402083332377));
#35664=CARTESIAN_POINT('Ctrl Pts',(25.187903481163,62.3519600867804,209.343749999044));
#35665=CARTESIAN_POINT('Ctrl Pts',(24.577346537413,62.70446530261,209.285416665711));
#35666=CARTESIAN_POINT('Ctrl Pts',(23.966789593663,63.0569705184397,209.227083332377));
#35667=CARTESIAN_POINT('Ctrl Pts',(23.966789593663,63.761980950099,209.168749999044));
#35668=CARTESIAN_POINT('Ctrl Pts',(23.966789593663,64.4669913817583,209.110416665711));
#35669=CARTESIAN_POINT('Ctrl Pts',(24.577346537413,64.819496597588,209.052083332377));
#35670=CARTESIAN_POINT('Ctrl Pts',(25.187903481163,65.1720018134176,208.993749999044));
#35671=CARTESIAN_POINT('Ctrl Pts',(25.798460424913,64.819496597588,208.935416665711));
#35672=CARTESIAN_POINT('Ctrl Pts',(26.409017368663,64.4669913817583,208.877083332377));
#35673=CARTESIAN_POINT('Ctrl Pts',(26.409017368663,63.761980950099,208.818749999044));
#35674=CARTESIAN_POINT('Ctrl Pts',(26.409017368663,63.0569705184397,208.760416665711));
#35675=CARTESIAN_POINT('Ctrl Pts',(25.798460424913,62.70446530261,208.702083332377));
#35676=CARTESIAN_POINT('Ctrl Pts',(25.187903481163,62.3519600867804,208.643749999044));
#35677=CARTESIAN_POINT('Ctrl Pts',(24.577346537413,62.70446530261,208.585416665711));
#35678=CARTESIAN_POINT('Ctrl Pts',(23.966789593663,63.0569705184397,208.527083332377));
#35679=CARTESIAN_POINT('Ctrl Pts',(23.966789593663,63.761980950099,208.468749999044));
#35680=CARTESIAN_POINT('Ctrl Pts',(23.966789593663,64.4669913817583,208.410416665711));
#35681=CARTESIAN_POINT('Ctrl Pts',(24.577346537413,64.819496597588,208.352083332377));
#35682=CARTESIAN_POINT('Ctrl Pts',(25.187903481163,65.1720018134176,208.293749999044));
#35683=CARTESIAN_POINT('Ctrl Pts',(25.798460424913,64.819496597588,208.235416665711));
#35684=CARTESIAN_POINT('Ctrl Pts',(26.409017368663,64.4669913817583,208.177083332377));
#35685=CARTESIAN_POINT('Ctrl Pts',(26.409017368663,63.761980950099,208.118749999044));
#35686=CARTESIAN_POINT('Ctrl Pts',(26.409017368663,63.0569705184397,208.060416665711));
#35687=CARTESIAN_POINT('Ctrl Pts',(25.798460424913,62.70446530261,208.002083332377));
#35688=CARTESIAN_POINT('Ctrl Pts',(25.187903481163,62.3519600867804,207.943749999044));
#35689=CARTESIAN_POINT('Ctrl Pts',(24.577346537413,62.70446530261,207.885416665711));
#35690=CARTESIAN_POINT('Ctrl Pts',(23.966789593663,63.0569705184397,207.827083332377));
#35691=CARTESIAN_POINT('Ctrl Pts',(23.966789593663,63.761980950099,207.768749999044));
#35692=CARTESIAN_POINT('Ctrl Pts',(23.966789593663,64.4669913817583,207.710416665711));
#35693=CARTESIAN_POINT('Ctrl Pts',(24.577346537413,64.819496597588,207.652083332377));
#35694=CARTESIAN_POINT('Ctrl Pts',(25.187903481163,65.1720018134176,207.593749999044));
#35695=CARTESIAN_POINT('Ctrl Pts',(25.798460424913,64.819496597588,207.535416665711));
#35696=CARTESIAN_POINT('Ctrl Pts',(26.409017368663,64.4669913817583,207.477083332377));
#35697=CARTESIAN_POINT('Ctrl Pts',(26.409017368663,63.761980950099,207.418749999044));
#35698=CARTESIAN_POINT('Ctrl Pts',(26.409017368663,63.0569705184397,207.360416665711));
#35699=CARTESIAN_POINT('Ctrl Pts',(25.798460424913,62.70446530261,207.302083332377));
#35700=CARTESIAN_POINT('Ctrl Pts',(25.187903481163,62.3519600867804,207.243749999044));
#35701=CARTESIAN_POINT('Ctrl Pts',(24.577346537413,62.70446530261,207.185416665711));
#35702=CARTESIAN_POINT('Ctrl Pts',(23.966789593663,63.0569705184397,207.127083332377));
#35703=CARTESIAN_POINT('Ctrl Pts',(23.966789593663,63.761980950099,207.068749999044));
#35704=CARTESIAN_POINT('Ctrl Pts',(23.966789593663,64.4669913817583,207.010416665711));
#35705=CARTESIAN_POINT('Ctrl Pts',(24.577346537413,64.819496597588,206.952083332377));
#35706=CARTESIAN_POINT('Ctrl Pts',(25.187903481163,65.1720018134176,206.893749999044));
#35707=CARTESIAN_POINT('Ctrl Pts',(25.798460424913,64.819496597588,206.835416665711));
#35708=CARTESIAN_POINT('Ctrl Pts',(26.409017368663,64.4669913817583,206.777083332377));
#35709=CARTESIAN_POINT('Ctrl Pts',(26.409017368663,63.761980950099,206.718749999044));
#35710=CARTESIAN_POINT('Ctrl Pts',(26.409017368663,63.0569705184397,206.660416665711));
#35711=CARTESIAN_POINT('Ctrl Pts',(25.798460424913,62.70446530261,206.602083332377));
#35712=CARTESIAN_POINT('Ctrl Pts',(25.187903481163,62.3519600867804,206.543749999044));
#35713=CARTESIAN_POINT('Ctrl Pts',(24.577346537413,62.70446530261,206.485416665711));
#35714=CARTESIAN_POINT('Ctrl Pts',(23.966789593663,63.0569705184397,206.427083332377));
#35715=CARTESIAN_POINT('Ctrl Pts',(23.966789593663,63.761980950099,206.368749999044));
#35716=CARTESIAN_POINT('Ctrl Pts',(23.966789593663,64.4669913817583,206.310416665711));
#35717=CARTESIAN_POINT('Ctrl Pts',(24.577346537413,64.819496597588,206.252083332377));
#35718=CARTESIAN_POINT('Ctrl Pts',(25.187903481163,65.1720018134176,206.193749999044));
#35719=CARTESIAN_POINT('Ctrl Pts',(25.798460424913,64.819496597588,206.135416665711));
#35720=CARTESIAN_POINT('Ctrl Pts',(26.409017368663,64.4669913817583,206.077083332377));
#35721=CARTESIAN_POINT('Ctrl Pts',(26.409017368663,63.761980950099,206.018749999044));
#35722=CARTESIAN_POINT('Ctrl Pts',(26.409017368663,63.0569705184397,205.960416665711));
#35723=CARTESIAN_POINT('Ctrl Pts',(25.798460424913,62.70446530261,205.902083332377));
#35724=CARTESIAN_POINT('Ctrl Pts',(25.187903481163,62.3519600867804,205.843749999044));
#35725=CARTESIAN_POINT('Ctrl Pts',(24.577346537413,62.70446530261,205.785416665711));
#35726=CARTESIAN_POINT('Ctrl Pts',(23.966789593663,63.0569705184397,205.727083332377));
#35727=CARTESIAN_POINT('Ctrl Pts',(23.966789593663,63.761980950099,205.668749999044));
#35728=CARTESIAN_POINT('Ctrl Pts',(23.966789593663,64.4669913817583,205.610416665711));
#35729=CARTESIAN_POINT('Ctrl Pts',(24.577346537413,64.819496597588,205.552083332377));
#35730=CARTESIAN_POINT('Ctrl Pts',(25.187903481163,65.1720018134176,205.493749999044));
#35731=CARTESIAN_POINT('Ctrl Pts',(25.798460424913,64.819496597588,205.435416665711));
#35732=CARTESIAN_POINT('Ctrl Pts',(26.409017368663,64.4669913817583,205.377083332377));
#35733=CARTESIAN_POINT('Ctrl Pts',(26.409017368663,63.761980950099,205.318749999044));
#35734=CARTESIAN_POINT('Ctrl Pts',(26.409017368663,63.0569705184397,205.260416665711));
#35735=CARTESIAN_POINT('Ctrl Pts',(25.798460424913,62.70446530261,205.202083332377));
#35736=CARTESIAN_POINT('Ctrl Pts',(25.187903481163,62.3519600867804,205.143749999044));
#35737=CARTESIAN_POINT('Ctrl Pts',(24.577346537413,62.70446530261,205.085416665711));
#35738=CARTESIAN_POINT('Ctrl Pts',(23.966789593663,63.0569705184397,205.027083332377));
#35739=CARTESIAN_POINT('Ctrl Pts',(23.966789593663,63.761980950099,204.968749999044));
#35740=CARTESIAN_POINT('Ctrl Pts',(23.966789593663,64.4669913817583,204.910416665711));
#35741=CARTESIAN_POINT('Ctrl Pts',(24.577346537413,64.819496597588,204.852083332377));
#35742=CARTESIAN_POINT('Ctrl Pts',(25.187903481163,65.1720018134176,204.793749999044));
#35743=CARTESIAN_POINT('Ctrl Pts',(25.798460424913,64.819496597588,204.735416665711));
#35744=CARTESIAN_POINT('Ctrl Pts',(26.409017368663,64.4669913817583,204.677083332377));
#35745=CARTESIAN_POINT('Ctrl Pts',(26.409017368663,63.761980950099,204.618749999044));
#35746=CARTESIAN_POINT('Ctrl Pts',(26.409017368663,63.0569705184397,204.560416665711));
#35747=CARTESIAN_POINT('Ctrl Pts',(25.798460424913,62.70446530261,204.502083332377));
#35748=CARTESIAN_POINT('Ctrl Pts',(25.187903481163,62.3519600867804,204.443749999044));
#35749=CARTESIAN_POINT('Ctrl Pts',(24.577346537413,62.70446530261,204.385416665711));
#35750=CARTESIAN_POINT('Ctrl Pts',(23.966789593663,63.0569705184397,204.327083332377));
#35751=CARTESIAN_POINT('Ctrl Pts',(23.966789593663,63.761980950099,204.268749999044));
#35752=CARTESIAN_POINT('Ctrl Pts',(23.966789593663,64.4669913817583,204.210416665711));
#35753=CARTESIAN_POINT('Ctrl Pts',(24.577346537413,64.819496597588,204.152083332377));
#35754=CARTESIAN_POINT('Ctrl Pts',(25.187903481163,65.1720018134176,204.093749999044));
#35755=CARTESIAN_POINT('Ctrl Pts',(25.798460424913,64.819496597588,204.035416665711));
#35756=CARTESIAN_POINT('Ctrl Pts',(26.409017368663,64.4669913817583,203.977083332377));
#35757=CARTESIAN_POINT('Ctrl Pts',(26.409017368663,63.761980950099,203.918749999044));
#35758=CARTESIAN_POINT('Ctrl Pts',(26.409017368663,63.0569705184397,203.860416665711));
#35759=CARTESIAN_POINT('Ctrl Pts',(25.798460424913,62.70446530261,203.802083332377));
#35760=CARTESIAN_POINT('Ctrl Pts',(25.187903481163,62.3519600867804,203.743749999044));
#35761=CARTESIAN_POINT('Ctrl Pts',(24.577346537413,62.70446530261,203.685416665711));
#35762=CARTESIAN_POINT('Ctrl Pts',(23.966789593663,63.0569705184397,203.627083332377));
#35763=CARTESIAN_POINT('Ctrl Pts',(23.966789593663,63.761980950099,203.568749999044));
#35764=CARTESIAN_POINT('Ctrl Pts',(23.966789593663,64.4669913817583,203.510416665711));
#35765=CARTESIAN_POINT('Ctrl Pts',(24.577346537413,64.819496597588,203.452083332377));
#35766=CARTESIAN_POINT('Ctrl Pts',(25.187903481163,65.1720018134176,203.393749999044));
#35767=CARTESIAN_POINT('Ctrl Pts',(25.798460424913,64.819496597588,203.335416665711));
#35768=CARTESIAN_POINT('Ctrl Pts',(26.409017368663,64.4669913817583,203.277083332377));
#35769=CARTESIAN_POINT('Ctrl Pts',(26.409017368663,63.761980950099,203.218749999044));
#35770=CARTESIAN_POINT('Ctrl Pts',(26.409017368663,63.0569705184397,203.160416665711));
#35771=CARTESIAN_POINT('Ctrl Pts',(25.798460424913,62.70446530261,203.102083332377));
#35772=CARTESIAN_POINT('Ctrl Pts',(25.187903481163,62.3519600867804,203.043749999044));
#35773=CARTESIAN_POINT('Ctrl Pts',(24.577346537413,62.70446530261,202.985416665711));
#35774=CARTESIAN_POINT('Ctrl Pts',(23.966789593663,63.0569705184397,202.927083332377));
#35775=CARTESIAN_POINT('Ctrl Pts',(23.966789593663,63.761980950099,202.868749999044));
#35776=CARTESIAN_POINT('Ctrl Pts',(23.966789593663,64.4669913817583,202.810416665711));
#35777=CARTESIAN_POINT('Ctrl Pts',(24.577346537413,64.819496597588,202.752083332377));
#35778=CARTESIAN_POINT('Ctrl Pts',(25.187903481163,65.1720018134176,202.693749999044));
#35779=CARTESIAN_POINT('Ctrl Pts',(25.798460424913,64.819496597588,202.635416665711));
#35780=CARTESIAN_POINT('Ctrl Pts',(26.409017368663,64.4669913817583,202.577083332377));
#35781=CARTESIAN_POINT('Ctrl Pts',(26.409017368663,63.761980950099,202.518749999044));
#35782=CARTESIAN_POINT('Ctrl Pts',(26.787903481163,63.761980950099,212.1));
#35783=CARTESIAN_POINT('Ctrl Pts',(26.787903481163,62.8382205193956,212.041666666667));
#35784=CARTESIAN_POINT('Ctrl Pts',(25.987903481163,62.3763403040439,211.983333333333));
#35785=CARTESIAN_POINT('Ctrl Pts',(25.187903481163,61.9144600886922,211.925));
#35786=CARTESIAN_POINT('Ctrl Pts',(24.387903481163,62.3763403040439,211.866666666667));
#35787=CARTESIAN_POINT('Ctrl Pts',(23.587903481163,62.8382205193956,211.808333333333));
#35788=CARTESIAN_POINT('Ctrl Pts',(23.587903481163,63.761980950099,211.75));
#35789=CARTESIAN_POINT('Ctrl Pts',(23.587903481163,64.6857413808024,211.691666666667));
#35790=CARTESIAN_POINT('Ctrl Pts',(24.387903481163,65.1476215961541,211.633333333333));
#35791=CARTESIAN_POINT('Ctrl Pts',(25.187903481163,65.6095018115058,211.575));
#35792=CARTESIAN_POINT('Ctrl Pts',(25.987903481163,65.1476215961541,211.516666666667));
#35793=CARTESIAN_POINT('Ctrl Pts',(26.787903481163,64.6857413808024,211.458333333333));
#35794=CARTESIAN_POINT('Ctrl Pts',(26.787903481163,63.761980950099,211.4));
#35795=CARTESIAN_POINT('Ctrl Pts',(26.787903481163,62.8382205193956,211.341666666667));
#35796=CARTESIAN_POINT('Ctrl Pts',(25.987903481163,62.3763403040439,211.283333333333));
#35797=CARTESIAN_POINT('Ctrl Pts',(25.187903481163,61.9144600886922,211.225));
#35798=CARTESIAN_POINT('Ctrl Pts',(24.387903481163,62.3763403040439,211.166666666667));
#35799=CARTESIAN_POINT('Ctrl Pts',(23.587903481163,62.8382205193956,211.108333333333));
#35800=CARTESIAN_POINT('Ctrl Pts',(23.587903481163,63.761980950099,211.05));
#35801=CARTESIAN_POINT('Ctrl Pts',(23.587903481163,64.6857413808024,210.991666666667));
#35802=CARTESIAN_POINT('Ctrl Pts',(24.387903481163,65.1476215961541,210.933333333333));
#35803=CARTESIAN_POINT('Ctrl Pts',(25.187903481163,65.6095018115058,210.875));
#35804=CARTESIAN_POINT('Ctrl Pts',(25.987903481163,65.1476215961541,210.816666666667));
#35805=CARTESIAN_POINT('Ctrl Pts',(26.787903481163,64.6857413808024,210.758333333333));
#35806=CARTESIAN_POINT('Ctrl Pts',(26.787903481163,63.761980950099,210.7));
#35807=CARTESIAN_POINT('Ctrl Pts',(26.787903481163,62.8382205193956,210.641666666667));
#35808=CARTESIAN_POINT('Ctrl Pts',(25.987903481163,62.3763403040439,210.583333333333));
#35809=CARTESIAN_POINT('Ctrl Pts',(25.187903481163,61.9144600886922,210.525));
#35810=CARTESIAN_POINT('Ctrl Pts',(24.387903481163,62.3763403040439,210.466666666667));
#35811=CARTESIAN_POINT('Ctrl Pts',(23.587903481163,62.8382205193956,210.408333333333));
#35812=CARTESIAN_POINT('Ctrl Pts',(23.587903481163,63.761980950099,210.35));
#35813=CARTESIAN_POINT('Ctrl Pts',(23.587903481163,64.6857413808024,210.291666666667));
#35814=CARTESIAN_POINT('Ctrl Pts',(24.387903481163,65.1476215961541,210.233333333333));
#35815=CARTESIAN_POINT('Ctrl Pts',(25.187903481163,65.6095018115058,210.175));
#35816=CARTESIAN_POINT('Ctrl Pts',(25.987903481163,65.1476215961541,210.116666666667));
#35817=CARTESIAN_POINT('Ctrl Pts',(26.787903481163,64.6857413808024,210.058333333333));
#35818=CARTESIAN_POINT('Ctrl Pts',(26.787903481163,63.761980950099,210.));
#35819=CARTESIAN_POINT('Ctrl Pts',(26.787903481163,62.8382205193956,209.941666666667));
#35820=CARTESIAN_POINT('Ctrl Pts',(25.987903481163,62.3763403040439,209.883333333333));
#35821=CARTESIAN_POINT('Ctrl Pts',(25.187903481163,61.9144600886922,209.825));
#35822=CARTESIAN_POINT('Ctrl Pts',(24.387903481163,62.3763403040439,209.766666666667));
#35823=CARTESIAN_POINT('Ctrl Pts',(23.587903481163,62.8382205193956,209.708333333333));
#35824=CARTESIAN_POINT('Ctrl Pts',(23.587903481163,63.761980950099,209.65));
#35825=CARTESIAN_POINT('Ctrl Pts',(23.587903481163,64.6857413808024,209.591666666667));
#35826=CARTESIAN_POINT('Ctrl Pts',(24.387903481163,65.1476215961541,209.533333333333));
#35827=CARTESIAN_POINT('Ctrl Pts',(25.187903481163,65.6095018115058,209.475));
#35828=CARTESIAN_POINT('Ctrl Pts',(25.987903481163,65.1476215961541,209.416666666667));
#35829=CARTESIAN_POINT('Ctrl Pts',(26.787903481163,64.6857413808024,209.358333333333));
#35830=CARTESIAN_POINT('Ctrl Pts',(26.787903481163,63.761980950099,209.3));
#35831=CARTESIAN_POINT('Ctrl Pts',(26.787903481163,62.8382205193956,209.241666666667));
#35832=CARTESIAN_POINT('Ctrl Pts',(25.987903481163,62.3763403040439,209.183333333333));
#35833=CARTESIAN_POINT('Ctrl Pts',(25.187903481163,61.9144600886922,209.125));
#35834=CARTESIAN_POINT('Ctrl Pts',(24.387903481163,62.3763403040439,209.066666666667));
#35835=CARTESIAN_POINT('Ctrl Pts',(23.587903481163,62.8382205193956,209.008333333333));
#35836=CARTESIAN_POINT('Ctrl Pts',(23.587903481163,63.761980950099,208.95));
#35837=CARTESIAN_POINT('Ctrl Pts',(23.587903481163,64.6857413808024,208.891666666667));
#35838=CARTESIAN_POINT('Ctrl Pts',(24.387903481163,65.1476215961541,208.833333333333));
#35839=CARTESIAN_POINT('Ctrl Pts',(25.187903481163,65.6095018115058,208.775));
#35840=CARTESIAN_POINT('Ctrl Pts',(25.987903481163,65.1476215961541,208.716666666667));
#35841=CARTESIAN_POINT('Ctrl Pts',(26.787903481163,64.6857413808024,208.658333333333));
#35842=CARTESIAN_POINT('Ctrl Pts',(26.787903481163,63.761980950099,208.6));
#35843=CARTESIAN_POINT('Ctrl Pts',(26.787903481163,62.8382205193956,208.541666666667));
#35844=CARTESIAN_POINT('Ctrl Pts',(25.987903481163,62.3763403040439,208.483333333333));
#35845=CARTESIAN_POINT('Ctrl Pts',(25.187903481163,61.9144600886922,208.425));
#35846=CARTESIAN_POINT('Ctrl Pts',(24.387903481163,62.3763403040439,208.366666666667));
#35847=CARTESIAN_POINT('Ctrl Pts',(23.587903481163,62.8382205193956,208.308333333333));
#35848=CARTESIAN_POINT('Ctrl Pts',(23.587903481163,63.761980950099,208.25));
#35849=CARTESIAN_POINT('Ctrl Pts',(23.587903481163,64.6857413808024,208.191666666667));
#35850=CARTESIAN_POINT('Ctrl Pts',(24.387903481163,65.1476215961541,208.133333333333));
#35851=CARTESIAN_POINT('Ctrl Pts',(25.187903481163,65.6095018115058,208.075));
#35852=CARTESIAN_POINT('Ctrl Pts',(25.987903481163,65.1476215961541,208.016666666667));
#35853=CARTESIAN_POINT('Ctrl Pts',(26.787903481163,64.6857413808024,207.958333333333));
#35854=CARTESIAN_POINT('Ctrl Pts',(26.787903481163,63.761980950099,207.9));
#35855=CARTESIAN_POINT('Ctrl Pts',(26.787903481163,62.8382205193956,207.841666666667));
#35856=CARTESIAN_POINT('Ctrl Pts',(25.987903481163,62.3763403040439,207.783333333333));
#35857=CARTESIAN_POINT('Ctrl Pts',(25.187903481163,61.9144600886922,207.725));
#35858=CARTESIAN_POINT('Ctrl Pts',(24.387903481163,62.3763403040439,207.666666666667));
#35859=CARTESIAN_POINT('Ctrl Pts',(23.587903481163,62.8382205193956,207.608333333333));
#35860=CARTESIAN_POINT('Ctrl Pts',(23.587903481163,63.761980950099,207.55));
#35861=CARTESIAN_POINT('Ctrl Pts',(23.587903481163,64.6857413808024,207.491666666667));
#35862=CARTESIAN_POINT('Ctrl Pts',(24.387903481163,65.1476215961541,207.433333333333));
#35863=CARTESIAN_POINT('Ctrl Pts',(25.187903481163,65.6095018115058,207.375));
#35864=CARTESIAN_POINT('Ctrl Pts',(25.987903481163,65.1476215961541,207.316666666667));
#35865=CARTESIAN_POINT('Ctrl Pts',(26.787903481163,64.6857413808024,207.258333333333));
#35866=CARTESIAN_POINT('Ctrl Pts',(26.787903481163,63.761980950099,207.2));
#35867=CARTESIAN_POINT('Ctrl Pts',(26.787903481163,62.8382205193956,207.141666666667));
#35868=CARTESIAN_POINT('Ctrl Pts',(25.987903481163,62.3763403040439,207.083333333333));
#35869=CARTESIAN_POINT('Ctrl Pts',(25.187903481163,61.9144600886922,207.025));
#35870=CARTESIAN_POINT('Ctrl Pts',(24.387903481163,62.3763403040439,206.966666666667));
#35871=CARTESIAN_POINT('Ctrl Pts',(23.587903481163,62.8382205193956,206.908333333333));
#35872=CARTESIAN_POINT('Ctrl Pts',(23.587903481163,63.761980950099,206.85));
#35873=CARTESIAN_POINT('Ctrl Pts',(23.587903481163,64.6857413808024,206.791666666667));
#35874=CARTESIAN_POINT('Ctrl Pts',(24.387903481163,65.1476215961541,206.733333333333));
#35875=CARTESIAN_POINT('Ctrl Pts',(25.187903481163,65.6095018115058,206.675));
#35876=CARTESIAN_POINT('Ctrl Pts',(25.987903481163,65.1476215961541,206.616666666667));
#35877=CARTESIAN_POINT('Ctrl Pts',(26.787903481163,64.6857413808024,206.558333333333));
#35878=CARTESIAN_POINT('Ctrl Pts',(26.787903481163,63.761980950099,206.5));
#35879=CARTESIAN_POINT('Ctrl Pts',(26.787903481163,62.8382205193956,206.441666666667));
#35880=CARTESIAN_POINT('Ctrl Pts',(25.987903481163,62.3763403040439,206.383333333333));
#35881=CARTESIAN_POINT('Ctrl Pts',(25.187903481163,61.9144600886922,206.325));
#35882=CARTESIAN_POINT('Ctrl Pts',(24.387903481163,62.3763403040439,206.266666666667));
#35883=CARTESIAN_POINT('Ctrl Pts',(23.587903481163,62.8382205193956,206.208333333333));
#35884=CARTESIAN_POINT('Ctrl Pts',(23.587903481163,63.761980950099,206.15));
#35885=CARTESIAN_POINT('Ctrl Pts',(23.587903481163,64.6857413808024,206.091666666667));
#35886=CARTESIAN_POINT('Ctrl Pts',(24.387903481163,65.1476215961541,206.033333333333));
#35887=CARTESIAN_POINT('Ctrl Pts',(25.187903481163,65.6095018115058,205.975));
#35888=CARTESIAN_POINT('Ctrl Pts',(25.987903481163,65.1476215961541,205.916666666667));
#35889=CARTESIAN_POINT('Ctrl Pts',(26.787903481163,64.6857413808024,205.858333333333));
#35890=CARTESIAN_POINT('Ctrl Pts',(26.787903481163,63.761980950099,205.8));
#35891=CARTESIAN_POINT('Ctrl Pts',(26.787903481163,62.8382205193956,205.741666666667));
#35892=CARTESIAN_POINT('Ctrl Pts',(25.987903481163,62.3763403040439,205.683333333333));
#35893=CARTESIAN_POINT('Ctrl Pts',(25.187903481163,61.9144600886922,205.625));
#35894=CARTESIAN_POINT('Ctrl Pts',(24.387903481163,62.3763403040439,205.566666666667));
#35895=CARTESIAN_POINT('Ctrl Pts',(23.587903481163,62.8382205193956,205.508333333333));
#35896=CARTESIAN_POINT('Ctrl Pts',(23.587903481163,63.761980950099,205.45));
#35897=CARTESIAN_POINT('Ctrl Pts',(23.587903481163,64.6857413808024,205.391666666667));
#35898=CARTESIAN_POINT('Ctrl Pts',(24.387903481163,65.1476215961541,205.333333333333));
#35899=CARTESIAN_POINT('Ctrl Pts',(25.187903481163,65.6095018115058,205.275));
#35900=CARTESIAN_POINT('Ctrl Pts',(25.987903481163,65.1476215961541,205.216666666667));
#35901=CARTESIAN_POINT('Ctrl Pts',(26.787903481163,64.6857413808024,205.158333333333));
#35902=CARTESIAN_POINT('Ctrl Pts',(26.787903481163,63.761980950099,205.1));
#35903=CARTESIAN_POINT('Ctrl Pts',(26.787903481163,62.8382205193956,205.041666666667));
#35904=CARTESIAN_POINT('Ctrl Pts',(25.987903481163,62.3763403040439,204.983333333333));
#35905=CARTESIAN_POINT('Ctrl Pts',(25.187903481163,61.9144600886922,204.925));
#35906=CARTESIAN_POINT('Ctrl Pts',(24.387903481163,62.3763403040439,204.866666666667));
#35907=CARTESIAN_POINT('Ctrl Pts',(23.587903481163,62.8382205193956,204.808333333333));
#35908=CARTESIAN_POINT('Ctrl Pts',(23.587903481163,63.761980950099,204.75));
#35909=CARTESIAN_POINT('Ctrl Pts',(23.587903481163,64.6857413808024,204.691666666667));
#35910=CARTESIAN_POINT('Ctrl Pts',(24.387903481163,65.1476215961541,204.633333333333));
#35911=CARTESIAN_POINT('Ctrl Pts',(25.187903481163,65.6095018115058,204.575));
#35912=CARTESIAN_POINT('Ctrl Pts',(25.987903481163,65.1476215961541,204.516666666667));
#35913=CARTESIAN_POINT('Ctrl Pts',(26.787903481163,64.6857413808024,204.458333333333));
#35914=CARTESIAN_POINT('Ctrl Pts',(26.787903481163,63.761980950099,204.4));
#35915=CARTESIAN_POINT('Ctrl Pts',(26.787903481163,62.8382205193956,204.341666666667));
#35916=CARTESIAN_POINT('Ctrl Pts',(25.987903481163,62.3763403040439,204.283333333333));
#35917=CARTESIAN_POINT('Ctrl Pts',(25.187903481163,61.9144600886922,204.225));
#35918=CARTESIAN_POINT('Ctrl Pts',(24.387903481163,62.3763403040439,204.166666666667));
#35919=CARTESIAN_POINT('Ctrl Pts',(23.587903481163,62.8382205193956,204.108333333333));
#35920=CARTESIAN_POINT('Ctrl Pts',(23.587903481163,63.761980950099,204.05));
#35921=CARTESIAN_POINT('Ctrl Pts',(23.587903481163,64.6857413808024,203.991666666667));
#35922=CARTESIAN_POINT('Ctrl Pts',(24.387903481163,65.1476215961541,203.933333333333));
#35923=CARTESIAN_POINT('Ctrl Pts',(25.187903481163,65.6095018115058,203.875));
#35924=CARTESIAN_POINT('Ctrl Pts',(25.987903481163,65.1476215961541,203.816666666667));
#35925=CARTESIAN_POINT('Ctrl Pts',(26.787903481163,64.6857413808024,203.758333333333));
#35926=CARTESIAN_POINT('Ctrl Pts',(26.787903481163,63.761980950099,203.7));
#35927=CARTESIAN_POINT('Ctrl Pts',(26.787903481163,62.8382205193956,203.641666666667));
#35928=CARTESIAN_POINT('Ctrl Pts',(25.987903481163,62.3763403040439,203.583333333333));
#35929=CARTESIAN_POINT('Ctrl Pts',(25.187903481163,61.9144600886922,203.525));
#35930=CARTESIAN_POINT('Ctrl Pts',(24.387903481163,62.3763403040439,203.466666666667));
#35931=CARTESIAN_POINT('Ctrl Pts',(23.587903481163,62.8382205193956,203.408333333333));
#35932=CARTESIAN_POINT('Ctrl Pts',(23.587903481163,63.761980950099,203.35));
#35933=CARTESIAN_POINT('Ctrl Pts',(23.587903481163,64.6857413808024,203.291666666667));
#35934=CARTESIAN_POINT('Ctrl Pts',(24.387903481163,65.1476215961541,203.233333333333));
#35935=CARTESIAN_POINT('Ctrl Pts',(25.187903481163,65.6095018115058,203.175));
#35936=CARTESIAN_POINT('Ctrl Pts',(25.987903481163,65.1476215961541,203.116666666667));
#35937=CARTESIAN_POINT('Ctrl Pts',(26.787903481163,64.6857413808024,203.058333333333));
#35938=CARTESIAN_POINT('Ctrl Pts',(26.787903481163,63.761980950099,203.));
#35939=CARTESIAN_POINT('Ctrl Pts',(26.787903481163,62.8382205193956,202.941666666667));
#35940=CARTESIAN_POINT('Ctrl Pts',(25.987903481163,62.3763403040439,202.883333333333));
#35941=CARTESIAN_POINT('Ctrl Pts',(25.187903481163,61.9144600886922,202.825));
#35942=CARTESIAN_POINT('Ctrl Pts',(24.387903481163,62.3763403040439,202.766666666667));
#35943=CARTESIAN_POINT('Ctrl Pts',(23.587903481163,62.8382205193956,202.708333333333));
#35944=CARTESIAN_POINT('Ctrl Pts',(23.587903481163,63.761980950099,202.65));
#35945=CARTESIAN_POINT('Ctrl Pts',(23.587903481163,64.6857413808024,202.591666666667));
#35946=CARTESIAN_POINT('Ctrl Pts',(24.387903481163,65.1476215961541,202.533333333333));
#35947=CARTESIAN_POINT('Ctrl Pts',(25.187903481163,65.6095018115058,202.475));
#35948=CARTESIAN_POINT('Ctrl Pts',(25.987903481163,65.1476215961541,202.416666666667));
#35949=CARTESIAN_POINT('Ctrl Pts',(26.787903481163,64.6857413808024,202.358333333333));
#35950=CARTESIAN_POINT('Ctrl Pts',(26.787903481163,63.761980950099,202.3));
#35951=CARTESIAN_POINT('',(26.598460424913,63.761980950099,212.209374999522));
#35952=CARTESIAN_POINT('Ctrl Pts',(26.787903481163,63.761980950099,212.1));
#35953=CARTESIAN_POINT('Ctrl Pts',(26.787903481163,63.5528822225132,212.086795899272));
#35954=CARTESIAN_POINT('Ctrl Pts',(26.7469152133774,63.3458641356268,212.072228822259));
#35955=CARTESIAN_POINT('Ctrl Pts',(26.5867614174791,62.957027061243,212.041835720424));
#35956=CARTESIAN_POINT('Ctrl Pts',(26.4681877346425,62.7793122371604,212.026290441717));
#35957=CARTESIAN_POINT('Ctrl Pts',(26.1715229442533,62.4830672025603,211.996767349568));
#35958=CARTESIAN_POINT('Ctrl Pts',(25.9974726268862,62.3663763860522,211.984031083542));
#35959=CARTESIAN_POINT('Ctrl Pts',(25.6158431081187,62.2065561348171,211.956203931132));
#35960=CARTESIAN_POINT('Ctrl Pts',(25.412171684918,62.1644358549729,211.941352889857));
#35961=CARTESIAN_POINT('Ctrl Pts',(24.9920026023566,62.159641416223,211.91071556092));
#35962=CARTESIAN_POINT('Ctrl Pts',(24.7794798571627,62.2002214897408,211.89521911075));
#35963=CARTESIAN_POINT('Ctrl Pts',(24.3930591021861,62.358565076682,211.867042597366));
#35964=CARTESIAN_POINT('Ctrl Pts',(24.2213486307701,62.4708047689436,211.854629142074));
#35965=CARTESIAN_POINT('Ctrl Pts',(23.9253596763751,62.7572595686795,211.825748920453));
#35966=CARTESIAN_POINT('Ctrl Pts',(23.8053148587378,62.9301656277874,211.810453669002));
#35967=CARTESIAN_POINT('Ctrl Pts',(23.6368471212299,63.3156176230095,211.779971214628));
#35968=CARTESIAN_POINT('Ctrl Pts',(23.5913649953638,63.5250588476194,211.7650872835));
#35969=CARTESIAN_POINT('Ctrl Pts',(23.5849639057201,63.9403798129072,211.738627352662));
#35970=CARTESIAN_POINT('Ctrl Pts',(23.6205201181075,64.1423015128207,211.724794488421));
#35971=CARTESIAN_POINT('Ctrl Pts',(23.7681882652492,64.5293978139233,211.694966518335));
#35972=CARTESIAN_POINT('Ctrl Pts',(23.8816542499166,64.7097359091757,211.679441804286));
#35973=CARTESIAN_POINT('Ctrl Pts',(24.1707256249538,65.0146100844818,211.64965064514));
#35974=CARTESIAN_POINT('Ctrl Pts',(24.3429020179363,65.1366372748414,211.636614690027));
#35975=CARTESIAN_POINT('Ctrl Pts',(24.7213214416994,65.3061875351901,211.609021607044));
#35976=CARTESIAN_POINT('Ctrl Pts',(24.9233666896425,65.3532878029956,211.594289141048));
#35977=CARTESIAN_POINT('Ctrl Pts',(25.3422082252478,65.3687851666763,211.56374861241));
#35978=CARTESIAN_POINT('Ctrl Pts',(25.5551431832926,65.3338567177254,211.548222105053));
#35979=CARTESIAN_POINT('Ctrl Pts',(25.9456448926417,65.1858542596342,211.51974802208));
#35980=CARTESIAN_POINT('Ctrl Pts',(26.1207180230927,65.0778263003631,211.507417058424));
#35981=CARTESIAN_POINT('Ctrl Pts',(26.4239592468199,64.7990100221814,211.478754786108));
#35982=CARTESIAN_POINT('Ctrl Pts',(26.5481450116235,64.6297298167745,211.463537526895));
#35983=CARTESIAN_POINT('Ctrl Pts',(26.726580176644,64.249330335995,211.43301073132));
#35984=CARTESIAN_POINT('Ctrl Pts',(26.7776079136368,64.0411270257476,211.41800278788));
#35985=CARTESIAN_POINT('Ctrl Pts',(26.7874362346422,63.8066458051222,211.402837517256));
#35986=CARTESIAN_POINT('Ctrl Pts',(26.787903481163,63.7843058451588,211.401409765456));
#35987=CARTESIAN_POINT('Ctrl Pts',(26.787903481163,63.7619809500992,211.4));
#35988=CARTESIAN_POINT('',(26.787903481163,63.761980950099,202.3));
#35989=CARTESIAN_POINT('Ctrl Pts',(23.7486592957405,64.4609631921677,202.6));
#35990=CARTESIAN_POINT('Ctrl Pts',(23.9630003818437,64.9023036773826,202.564315850992));
#35991=CARTESIAN_POINT('Ctrl Pts',(24.387903481163,65.1476215961541,202.533333333333));
#35992=CARTESIAN_POINT('Ctrl Pts',(25.187903481163,65.6095018115058,202.475));
#35993=CARTESIAN_POINT('Ctrl Pts',(25.987903481163,65.1476215961541,202.416666666667));
#35994=CARTESIAN_POINT('Ctrl Pts',(26.787903481163,64.6857413808024,202.358333333333));
#35995=CARTESIAN_POINT('Ctrl Pts',(26.787903481163,63.761980950099,202.3));
#35996=CARTESIAN_POINT('',(26.598460424913,63.761980950099,202.409374999522));
#35997=CARTESIAN_POINT('Origin',(26.598460424913,63.761980950099,202.409374999522));
#35998=CARTESIAN_POINT('',(26.787903481163,63.761980950099,202.606249999044));
#35999=CARTESIAN_POINT('Origin',(26.598460424913,63.761980950099,212.209374999522));
#36000=CARTESIAN_POINT('Origin',(25.1879034811632,63.761980950099,212.406249999044));
#36001=CARTESIAN_POINT('Origin',(25.187903481163,63.761980950099,202.6));
#36002=CARTESIAN_POINT('Origin',(25.187903481163,63.761980950099,212.1));
#36003=CARTESIAN_POINT('',(23.187903481163,63.761980950099,212.5));
#36004=CARTESIAN_POINT('',(23.587903481163,63.761980950099,212.1));
#36005=CARTESIAN_POINT('Origin',(25.187903481163,63.761980950099,212.5));
#36006=CARTESIAN_POINT('Origin',(25.187903481163,63.761980950099,202.2));
#36007=CARTESIAN_POINT('',(27.187903481163,63.761980950099,202.2));
#36008=CARTESIAN_POINT('Origin',(25.187903481163,63.761980950099,212.5));
#36009=CARTESIAN_POINT('',(21.2239277116833,64.2976077782208,212.1));
#36010=CARTESIAN_POINT('',(29.187903481163,63.761980950099,212.1));
#36011=CARTESIAN_POINT('Origin',(25.187903481163,63.761980950099,212.1));
#36012=CARTESIAN_POINT('Origin',(25.187903481163,63.761980950099,212.1));
#36013=CARTESIAN_POINT('',(28.787903481163,63.761980950099,212.5));
#36014=CARTESIAN_POINT('',(28.787903481163,63.761980950099,212.5));
#36015=CARTESIAN_POINT('Origin',(25.187903481163,63.761980950099,212.5));
#36016=CARTESIAN_POINT('Origin',(25.187903481163,63.761980950099,212.5));
#36017=CARTESIAN_POINT('Origin',(25.187903481163,63.761980950099,212.5));
#36018=CARTESIAN_POINT('Origin',(19.9513700273636,43.5818784659284,205.8));
#36019=CARTESIAN_POINT('Origin',(-18.1629964860985,83.0516975441391,209.8));
#36020=CARTESIAN_POINT('',(-13.2080267742527,82.3821640089894,209.8));
#36021=CARTESIAN_POINT('Origin',(-18.1629964860985,83.0516975441391,209.8));
#36022=CARTESIAN_POINT('',(-13.7035237454372,82.4491173625044,210.3));
#36023=CARTESIAN_POINT('Origin',(-13.7035237454372,82.4491173625044,209.8));
#36024=CARTESIAN_POINT('Origin',(-18.1629964860985,83.0516975441391,210.3));
#36025=CARTESIAN_POINT('Origin',(-18.1629964860985,83.0516975441391,201.8));
#36026=CARTESIAN_POINT('',(-13.7035237454372,82.4491173625044,201.3));
#36027=CARTESIAN_POINT('Origin',(-18.1629964860985,83.0516975441391,201.3));
#36028=CARTESIAN_POINT('',(-13.2080267742527,82.3821640089894,201.8));
#36029=CARTESIAN_POINT('Origin',(-13.7035237454372,82.4491173625044,201.8));
#36030=CARTESIAN_POINT('Origin',(-18.1629964860985,83.0516975441391,201.8));
#36031=CARTESIAN_POINT('Origin',(-18.1629964860985,83.0516975441391,210.3));
#36032=CARTESIAN_POINT('',(-13.2080267742527,82.3821640089894,210.3));
#36033=CARTESIAN_POINT('Origin',(25.18790348116,63.761980950101,201.3));
#36034=CARTESIAN_POINT('',(18.2509458845758,64.6993278993105,211.3));
#36035=CARTESIAN_POINT('Origin',(25.18790348116,63.761980950101,211.3));
#36036=CARTESIAN_POINT('',(18.2509458845758,64.6993278993105,201.3));
#36037=CARTESIAN_POINT('Origin',(43.0811453810906,77.1117683798125,211.3));
#36038=CARTESIAN_POINT('',(40.5678791273553,80.5028251540171,209.3));
#36039=CARTESIAN_POINT('',(45.6182378895769,73.7385006893635,209.3));
#36040=CARTESIAN_POINT('Origin',(43.0811453810902,77.1117683798122,209.3));
#36041=CARTESIAN_POINT('',(40.5678791273553,80.5028251540171,210.3));
#36042=CARTESIAN_POINT('',(40.5678791273553,80.5028251540171,211.3));
#36043=CARTESIAN_POINT('',(45.6182378895769,73.7385006893635,210.3));
#36044=CARTESIAN_POINT('Origin',(43.0811453810904,77.1117683798123,210.3));
#36045=CARTESIAN_POINT('',(45.6182378895769,73.7385006893635,211.3));
#36046=CARTESIAN_POINT('Origin',(-18.1629964860985,83.0516975441391,214.3));
#36047=CARTESIAN_POINT('',(-16.5774061783079,82.8374468128912,210.3));
#36048=CARTESIAN_POINT('Origin',(-18.1629964860985,83.0516975441391,210.3));
#36049=CARTESIAN_POINT('',(-16.5774061783079,82.8374468128912,211.3));
#36050=CARTESIAN_POINT('',(-16.5774061783079,82.8374468128912,214.3));
#36051=CARTESIAN_POINT('Origin',(-18.1629964860985,83.0516975441391,211.3));
#36052=CARTESIAN_POINT('Origin',(19.9513700273636,43.5818784659284,211.3));
#36053=CARTESIAN_POINT('',(33.0886175986719,60.6545323126593,211.3));
#36054=CARTESIAN_POINT('',(27.3961507532244,48.8565674904361,211.3));
#36055=CARTESIAN_POINT('',(33.0886175986719,60.6545323126593,211.3));
#36056=CARTESIAN_POINT('',(16.5874683335563,50.6796992602564,211.3));
#36057=CARTESIAN_POINT('',(16.5874683335563,50.6796992602564,211.3));
#36058=CARTESIAN_POINT('',(17.9737067090166,58.898200306828,211.3));
#36059=CARTESIAN_POINT('',(17.9737067090166,58.898200306828,211.3));
#36060=CARTESIAN_POINT('',(17.1520153223208,60.475703333365,211.3));
#36061=CARTESIAN_POINT('',(17.9737067090166,58.898200306828,211.3));
#36062=CARTESIAN_POINT('',(15.7499363351254,62.4777857800405,211.3));
#36063=CARTESIAN_POINT('',(17.1520153223208,60.475703333365,211.3));
#36064=CARTESIAN_POINT('',(-15.5987525505707,76.8301353719087,211.3));
#36065=CARTESIAN_POINT('',(15.7499363351254,62.4777857800405,211.3));
#36066=CARTESIAN_POINT('',(-20.5710649571149,78.5071727628224,211.3));
#36067=CARTESIAN_POINT('',(-15.5987525505707,76.8301353719087,211.3));
#36068=CARTESIAN_POINT('',(-14.5190710707069,86.6812025814917,211.3));
#36069=CARTESIAN_POINT('Origin',(-18.1629964860985,83.0516975441391,211.3));
#36070=CARTESIAN_POINT('',(-11.7413224523512,83.8924176965482,211.3));
#36071=CARTESIAN_POINT('',(-14.5190710707069,86.6812025814917,211.3));
#36072=CARTESIAN_POINT('',(8.52323991612264,75.4822066097016,211.3));
#36073=CARTESIAN_POINT('',(-11.7413224523512,83.8924176965482,211.3));
#36074=CARTESIAN_POINT('',(26.4178380401533,73.0642234051985,211.3));
#36075=CARTESIAN_POINT('',(8.52323991612264,75.4822066097016,211.3));
#36076=CARTESIAN_POINT('',(30.5560117383973,75.2396394283021,211.3));
#36077=CARTESIAN_POINT('',(26.4178380401533,73.0642234051985,211.3));
#36078=CARTESIAN_POINT('',(38.4831850337045,66.2877716357375,211.3));
#36079=CARTESIAN_POINT('',(41.6077496400986,62.7593147414841,211.3));
#36080=CARTESIAN_POINT('',(45.6182378895769,73.7385006893635,211.3));
#36081=CARTESIAN_POINT('Origin',(19.9513700273636,43.5818784659284,211.3));
#36082=CARTESIAN_POINT('',(23.5430846542788,40.8708664706021,212.8));
#36083=CARTESIAN_POINT('',(15.4918972867023,44.1844586475632,212.8));
#36084=CARTESIAN_POINT('Origin',(19.9513700273636,43.5818784659284,212.8));
#36085=CARTESIAN_POINT('',(23.5430846542788,40.8708664706021,213.8));
#36086=CARTESIAN_POINT('',(23.5430846542788,40.8708664706021,211.3));
#36087=CARTESIAN_POINT('',(15.4918972867023,44.1844586475632,213.8));
#36088=CARTESIAN_POINT('Origin',(19.9513700273636,43.5818784659284,213.8));
#36089=CARTESIAN_POINT('',(15.4918972867023,44.1844586475632,211.3));
#36090=CARTESIAN_POINT('Origin',(19.9513700273636,43.5818784659284,212.3));
#36091=CARTESIAN_POINT('',(16.8325960933951,52.1329722228591,212.3));
#36092=CARTESIAN_POINT('',(17.9737067090166,58.898200306828,212.3));
#36093=CARTESIAN_POINT('',(17.9737067090166,58.898200306828,212.3));
#36094=CARTESIAN_POINT('',(28.0630252423339,50.2387032106721,212.3));
#36095=CARTESIAN_POINT('',(27.8913277021599,50.2676639320753,212.3));
#36096=CARTESIAN_POINT('',(33.0886175986719,60.6545323126593,212.3));
#36097=CARTESIAN_POINT('',(33.0886175986719,60.6545323126593,212.3));
#36098=CARTESIAN_POINT('',(39.0756626604441,66.9064622546218,212.3));
#36099=CARTESIAN_POINT('',(45.6182378895769,73.7385006893635,212.3));
#36100=CARTESIAN_POINT('',(31.6613562950968,75.8207132147201,212.3));
#36101=CARTESIAN_POINT('',(42.7226967777198,62.5216181735379,212.3));
#36102=CARTESIAN_POINT('',(26.4178380401533,73.0642234051985,212.3));
#36103=CARTESIAN_POINT('',(26.4178380401533,73.0642234051985,212.3));
#36104=CARTESIAN_POINT('',(8.52323991612264,75.4822066097016,212.3));
#36105=CARTESIAN_POINT('',(8.52323991612264,75.4822066097016,212.3));
#36106=CARTESIAN_POINT('',(-11.7413224523512,83.8924176965482,212.3));
#36107=CARTESIAN_POINT('',(-11.7413224523512,83.8924176965482,212.3));
#36108=CARTESIAN_POINT('',(-14.5190710707069,86.6812025814917,212.3));
#36109=CARTESIAN_POINT('',(-14.5190710707069,86.6812025814917,212.3));
#36110=CARTESIAN_POINT('',(-20.5710649571149,78.5071727628224,212.3));
#36111=CARTESIAN_POINT('Origin',(-18.1629964860985,83.0516975441391,212.3));
#36112=CARTESIAN_POINT('',(-15.5987525505707,76.8301353719087,212.3));
#36113=CARTESIAN_POINT('',(-15.5987525505707,76.8301353719087,212.3));
#36114=CARTESIAN_POINT('',(15.7499363351254,62.4777857800405,212.3));
#36115=CARTESIAN_POINT('',(15.7499363351254,62.4777857800405,212.3));
#36116=CARTESIAN_POINT('',(17.1520153223208,60.475703333365,212.3));
#36117=CARTESIAN_POINT('',(17.1520153223208,60.475703333365,212.3));
#36118=CARTESIAN_POINT('',(17.9737067090166,58.898200306828,212.3));
#36119=CARTESIAN_POINT('',(21.2239277116833,64.2976077782208,212.3));
#36120=CARTESIAN_POINT('Origin',(25.18790348116,63.761980950101,212.3));
#36121=CARTESIAN_POINT('',(-15.7623923893876,80.4345282249253,212.3));
#36122=CARTESIAN_POINT('',(-14.7228500730009,83.7738348943986,212.3));
#36123=CARTESIAN_POINT('',(-15.7623923893876,80.4345282249253,212.3));
#36124=CARTESIAN_POINT('',(-19.1740879543717,79.6651449444885,212.3));
#36125=CARTESIAN_POINT('',(-19.1740879543717,79.6651449444885,212.3));
#36126=CARTESIAN_POINT('',(-21.546241202969,82.235068333525,212.3));
#36127=CARTESIAN_POINT('',(-21.546241202969,82.235068333525,212.3));
#36128=CARTESIAN_POINT('',(-20.5066988865823,85.5743750029983,212.3));
#36129=CARTESIAN_POINT('',(-20.5066988865823,85.5743750029983,212.3));
#36130=CARTESIAN_POINT('',(-17.0950033215982,86.3437582834351,212.3));
#36131=CARTESIAN_POINT('',(-17.0950033215982,86.3437582834351,212.3));
#36132=CARTESIAN_POINT('',(-14.7228500730009,83.7738348943986,212.3));
#36133=CARTESIAN_POINT('Origin',(17.9737067090166,58.898200306828,211.3));
#36134=CARTESIAN_POINT('',(16.6330079023238,50.9496867315321,213.8));
#36135=CARTESIAN_POINT('',(15.4918972867023,44.1844586475632,213.8));
#36136=CARTESIAN_POINT('',(16.7328019978594,51.5413294771956,213.2));
#36137=CARTESIAN_POINT('Origin',(16.6330079023238,50.9496867315321,213.2));
#36138=CARTESIAN_POINT('',(16.7328019978594,51.5413294771956,212.9));
#36139=CARTESIAN_POINT('',(16.7328019978594,51.5413294771956,213.8));
#36140=CARTESIAN_POINT('Origin',(16.8325960933951,52.1329722228591,212.9));
#36141=CARTESIAN_POINT('',(17.9737067090166,58.898200306828,211.3));
#36142=CARTESIAN_POINT('',(16.4876742380207,50.088056514593,211.9));
#36143=CARTESIAN_POINT('Origin',(16.5874683335563,50.6796992602564,211.9));
#36144=CARTESIAN_POINT('',(16.4876742380207,50.088056514593,212.2));
#36145=CARTESIAN_POINT('',(16.4876742380207,50.088056514593,212.8));
#36146=CARTESIAN_POINT('',(16.387880142485,49.4964137689295,212.8));
#36147=CARTESIAN_POINT('Origin',(16.387880142485,49.4964137689295,212.2));
#36148=CARTESIAN_POINT('',(16.4876742380207,50.088056514593,212.8));
#36149=CARTESIAN_POINT('Origin',(17.9737067090166,58.898200306828,211.3));
#36150=CARTESIAN_POINT('',(17.1520153223208,60.475703333365,211.3));
#36151=CARTESIAN_POINT('Origin',(17.1520153223208,60.475703333365,211.3));
#36152=CARTESIAN_POINT('',(15.7499363351254,62.4777857800405,211.3));
#36153=CARTESIAN_POINT('Origin',(15.7499363351254,62.4777857800405,211.3));
#36154=CARTESIAN_POINT('',(-15.5987525505707,76.8301353719087,211.3));
#36155=CARTESIAN_POINT('Origin',(-15.5987525505707,76.8301353719087,211.3));
#36156=CARTESIAN_POINT('',(-20.5710649571149,78.5071727628224,211.3));
#36157=CARTESIAN_POINT('Origin',(-18.1629964860985,83.0516975441391,211.3));
#36158=CARTESIAN_POINT('',(-14.5190710707069,86.6812025814917,211.3));
#36159=CARTESIAN_POINT('Origin',(-14.5190710707069,86.6812025814917,211.3));
#36160=CARTESIAN_POINT('',(-11.7413224523512,83.8924176965482,211.3));
#36161=CARTESIAN_POINT('Origin',(-11.7413224523512,83.8924176965482,211.3));
#36162=CARTESIAN_POINT('',(8.52323991612264,75.4822066097016,211.3));
#36163=CARTESIAN_POINT('Origin',(8.52323991612264,75.4822066097016,211.3));
#36164=CARTESIAN_POINT('',(26.4178380401533,73.0642234051985,211.3));
#36165=CARTESIAN_POINT('Origin',(26.4178380401533,73.0642234051985,211.3));
#36166=CARTESIAN_POINT('',(32.2948489085972,76.1537369305954,211.6));
#36167=CARTESIAN_POINT('Origin',(31.6613562950993,75.8207132147214,211.600000000003));
#36168=CARTESIAN_POINT('',(32.2948489085972,76.1537369305954,211.));
#36169=CARTESIAN_POINT('',(32.2948489085972,76.1537369305954,210.3));
#36170=CARTESIAN_POINT('',(32.9283415220976,76.4867606464707,210.3));
#36171=CARTESIAN_POINT('Origin',(32.9283415220973,76.4867606464705,211.));
#36172=CARTESIAN_POINT('',(32.2948489085972,76.1537369305954,210.3));
#36173=CARTESIAN_POINT('',(31.8320221920213,75.9104313739469,209.3));
#36174=CARTESIAN_POINT('',(31.1940169652093,75.5750354011245,209.3));
#36175=CARTESIAN_POINT('',(31.1940169652093,75.5750354011245,210.));
#36176=CARTESIAN_POINT('Origin',(31.8320221920246,75.9104313739487,210.000000000003));
#36177=CARTESIAN_POINT('',(31.1940169652093,75.5750354011245,210.6));
#36178=CARTESIAN_POINT('',(31.1940169652093,75.5750354011245,209.3));
#36179=CARTESIAN_POINT('Origin',(30.5560117383975,75.2396394283022,210.6));
#36180=CARTESIAN_POINT('Origin',(45.6182378895769,73.7385006893635,211.3));
#36181=CARTESIAN_POINT('',(39.56293242615,67.4152903002768,211.));
#36182=CARTESIAN_POINT('',(39.56293242615,67.4152903002768,211.6));
#36183=CARTESIAN_POINT('',(39.56293242615,67.4152903002768,210.3));
#36184=CARTESIAN_POINT('Origin',(39.0756626604456,66.9064622546234,211.600000000002));
#36185=CARTESIAN_POINT('',(33.0886175986719,60.6545323126593,211.3));
#36186=CARTESIAN_POINT('',(38.9689769974974,66.7950564970781,210.6));
#36187=CARTESIAN_POINT('Origin',(38.4831850337063,66.2877716357394,210.600000000002));
#36188=CARTESIAN_POINT('',(38.9689769974974,66.7950564970781,210.));
#36189=CARTESIAN_POINT('',(38.9689769974974,66.7950564970781,209.3));
#36190=CARTESIAN_POINT('',(39.4547689612902,67.3023413584188,209.3));
#36191=CARTESIAN_POINT('Origin',(39.454768961292,67.3023413584207,210.000000000003));
#36192=CARTESIAN_POINT('',(45.6182378895769,73.7385006893635,209.3));
#36193=CARTESIAN_POINT('',(40.0502021918559,67.9241183459317,210.3));
#36194=CARTESIAN_POINT('',(39.56293242615,67.4152903002768,210.3));
#36195=CARTESIAN_POINT('Origin',(40.0502021918592,67.9241183459352,211.000000000005));
#36196=CARTESIAN_POINT('Origin',(33.0886175986719,60.6545323126593,211.3));
#36197=CARTESIAN_POINT('',(27.7915336066242,49.6760211864118,213.2));
#36198=CARTESIAN_POINT('',(27.7915336066242,49.6760211864118,212.9));
#36199=CARTESIAN_POINT('',(27.7915336066242,49.6760211864118,213.8));
#36200=CARTESIAN_POINT('',(27.5200419709145,49.1133391621515,213.8));
#36201=CARTESIAN_POINT('Origin',(27.5200419709149,49.1133391621524,213.200000000001));
#36202=CARTESIAN_POINT('',(27.7915336066242,49.6760211864118,213.8));
#36203=CARTESIAN_POINT('',(26.853167481805,47.7312034419155,212.8));
#36204=CARTESIAN_POINT('',(23.5430846542788,40.8708664706021,212.8));
#36205=CARTESIAN_POINT('',(27.1246591175147,48.2938854661758,212.2));
#36206=CARTESIAN_POINT('Origin',(26.8531674818047,47.7312034419149,212.199999999999));
#36207=CARTESIAN_POINT('',(27.1246591175147,48.2938854661758,211.9));
#36208=CARTESIAN_POINT('',(27.1246591175147,48.2938854661758,212.8));
#36209=CARTESIAN_POINT('Origin',(27.3961507532234,48.856567490434,211.899999999998));
#36210=CARTESIAN_POINT('Origin',(28.0630252423357,50.2387032106758,212.900000000004));
#36211=CARTESIAN_POINT('Origin',(43.0811453810902,77.1117683798122,209.3));
#36212=CARTESIAN_POINT('',(31.7180758735483,76.03910679713,209.3));
#36213=CARTESIAN_POINT('Origin',(38.9689769974974,66.7950564970781,209.3));
#36214=CARTESIAN_POINT('',(38.9689769974974,66.7950564970781,210.6));
#36215=CARTESIAN_POINT('',(38.9689769974974,66.7950564970781,210.));
#36216=CARTESIAN_POINT('Origin',(32.2948489085972,76.1537369305954,210.3));
#36217=CARTESIAN_POINT('',(32.2948489085972,76.1537369305954,211.));
#36218=CARTESIAN_POINT('',(32.2948489085972,76.1537369305954,211.6));
#36219=CARTESIAN_POINT('Origin',(43.0811453810904,77.1117683798123,210.3));
#36220=CARTESIAN_POINT('',(40.1011097736976,67.8629119514361,210.3));
#36221=CARTESIAN_POINT('Origin',(36.7726348574482,71.8647509982436,211.));
#36222=CARTESIAN_POINT('Origin',(31.7566715610496,75.7061152794361,211.6));
#36223=CARTESIAN_POINT('Origin',(38.4449180891584,66.3309851010726,210.6));
#36224=CARTESIAN_POINT('Origin',(36.179921252864,71.0005074807578,210.));
#36225=CARTESIAN_POINT('Origin',(19.9513700273636,43.5818784659284,213.8));
#36226=CARTESIAN_POINT('',(16.6330079023238,50.9496867315321,213.8));
#36227=CARTESIAN_POINT('Origin',(16.7328019978594,51.5413294771956,213.8));
#36228=CARTESIAN_POINT('',(27.7915336066242,49.6760211864118,213.2));
#36229=CARTESIAN_POINT('',(16.7328019978594,51.5413294771956,212.9));
#36230=CARTESIAN_POINT('Origin',(27.1246591175147,48.2938854661758,212.8));
#36231=CARTESIAN_POINT('',(27.1246591175147,48.2938854661758,212.2));
#36232=CARTESIAN_POINT('',(27.1246591175147,48.2938854661758,211.9));
#36233=CARTESIAN_POINT('Origin',(19.9513700273636,43.5818784659284,212.8));
#36234=CARTESIAN_POINT('',(20.8228154955302,48.7483603776555,212.8));
#36235=CARTESIAN_POINT('Origin',(21.0679432553689,50.2016333402581,213.2));
#36236=CARTESIAN_POINT('Origin',(16.8325960933951,52.1329722228591,212.9));
#36237=CARTESIAN_POINT('Origin',(20.8228154955302,48.7483603776555,212.2));
#36238=CARTESIAN_POINT('Origin',(27.2244532130503,48.8855282118392,211.9));
#36239=CARTESIAN_POINT('Origin',(-18.1629964860985,83.0516975441391,210.3));
#36240=CARTESIAN_POINT('Origin',(-18.1629964860985,83.0516975441391,201.3));
#36241=CARTESIAN_POINT('Origin',(-19.1740879543717,79.6651449444885,202.784409248129));
#36242=CARTESIAN_POINT('',(-15.7623923893876,80.4345282249253,213.8));
#36243=CARTESIAN_POINT('',(-15.7623923893876,80.4345282249253,202.784409248129));
#36244=CARTESIAN_POINT('',(-19.1740879543717,79.6651449444885,213.8));
#36245=CARTESIAN_POINT('',(-19.1740879543717,79.6651449444885,213.8));
#36246=CARTESIAN_POINT('',(-19.1740879543717,79.6651449444885,202.784409248129));
#36247=CARTESIAN_POINT('Origin',(-15.7623923893876,80.4345282249253,202.784409248129));
#36248=CARTESIAN_POINT('',(-14.7228500730009,83.7738348943986,213.8));
#36249=CARTESIAN_POINT('',(-14.7228500730009,83.7738348943986,202.784409248129));
#36250=CARTESIAN_POINT('',(-15.7623923893876,80.4345282249253,213.8));
#36251=CARTESIAN_POINT('Origin',(-14.7228500730009,83.7738348943986,202.784409248129));
#36252=CARTESIAN_POINT('',(-17.0950033215982,86.3437582834351,213.8));
#36253=CARTESIAN_POINT('',(-17.0950033215982,86.3437582834351,202.784409248129));
#36254=CARTESIAN_POINT('',(-14.7228500730009,83.7738348943986,213.8));
#36255=CARTESIAN_POINT('Origin',(-17.0950033215982,86.3437582834351,202.784409248129));
#36256=CARTESIAN_POINT('',(-20.5066988865823,85.5743750029983,213.8));
#36257=CARTESIAN_POINT('',(-20.5066988865823,85.5743750029983,202.784409248129));
#36258=CARTESIAN_POINT('',(-17.0950033215982,86.3437582834351,213.8));
#36259=CARTESIAN_POINT('Origin',(-20.5066988865823,85.5743750029983,202.784409248129));
#36260=CARTESIAN_POINT('',(-21.546241202969,82.235068333525,213.8));
#36261=CARTESIAN_POINT('',(-21.546241202969,82.235068333525,202.784409248129));
#36262=CARTESIAN_POINT('',(-20.5066988865823,85.5743750029983,213.8));
#36263=CARTESIAN_POINT('Origin',(-21.546241202969,82.235068333525,202.784409248129));
#36264=CARTESIAN_POINT('',(-21.546241202969,82.235068333525,213.8));
#36265=CARTESIAN_POINT('Origin',(-18.1629964860985,83.0516975441391,214.3));
#36266=CARTESIAN_POINT('',(-17.2666121411095,85.7925017674652,214.3));
#36267=CARTESIAN_POINT('',(-20.1151011495063,85.1501291478031,214.3));
#36268=CARTESIAN_POINT('',(-20.3967044277999,85.0866238174157,214.3));
#36269=CARTESIAN_POINT('',(-20.9830346463817,82.3620789942997,214.3));
#36270=CARTESIAN_POINT('',(-21.0688390561374,82.0864507363147,214.3));
#36271=CARTESIAN_POINT('',(-19.0024791348604,80.2164014604584,214.3));
#36272=CARTESIAN_POINT('',(-18.8066802663224,80.0042785328608,214.3));
#36273=CARTESIAN_POINT('',(-16.1539901264636,80.8587740801205,214.3));
#36274=CARTESIAN_POINT('',(-15.87238684817,80.9222794105078,214.3));
#36275=CARTESIAN_POINT('',(-15.2860566295882,83.6468242336239,214.3));
#36276=CARTESIAN_POINT('',(-15.2002522198325,83.9224524916089,214.3));
#36277=CARTESIAN_POINT('',(-17.4624110096475,86.0046246950628,214.3));
#36278=CARTESIAN_POINT('Origin',(-15.7091285121886,82.2877965760055,213.8));
#36279=CARTESIAN_POINT('Origin',(-16.153990126463,80.8587740801198,213.800000000001));
#36280=CARTESIAN_POINT('Origin',(-15.2860566295866,83.6468242336243,213.800000000001));
#36281=CARTESIAN_POINT('Origin',(-16.3129705205095,84.7593535478096,213.8));
#36282=CARTESIAN_POINT('Origin',(-17.2666121411088,85.7925017674677,213.800000000002));
#36283=CARTESIAN_POINT('Origin',(-17.595169633509,80.5337686991571,213.8));
#36284=CARTESIAN_POINT('Origin',(-19.0024791348609,80.2164014604572,213.800000000001));
#36285=CARTESIAN_POINT('Origin',(-18.7077916481549,85.4674963865018,213.8));
#36286=CARTESIAN_POINT('Origin',(-20.1151011495067,85.1501291478035,213.8));
#36287=CARTESIAN_POINT('Origin',(-20.0293930257817,81.328930774644,213.8));
#36288=CARTESIAN_POINT('Origin',(-20.98303464638,82.3620789943001,213.799999999999));
#36289=CARTESIAN_POINT('Origin',(-20.5381730321068,83.7911014901847,213.8));
#36290=CARTESIAN_POINT('Origin',(25.18790348116,63.761980950101,211.3));
#36291=CARTESIAN_POINT('',(21.2239277116833,64.2976077782208,211.3));
#36292=CARTESIAN_POINT('Origin',(43.0811453810944,77.1117683798101,211.));
#36293=CARTESIAN_POINT('',(44.680857697675,77.0814285680054,211.));
#36294=CARTESIAN_POINT('Origin',(43.0811453810944,77.1117683798101,211.));
#36295=CARTESIAN_POINT('Origin',(43.0811453810944,77.1117683798101,211.8));
#36296=CARTESIAN_POINT('',(44.680857697675,77.0814285680054,210.6));
#36297=CARTESIAN_POINT('',(44.680857697675,77.0814285680054,211.8));
#36298=CARTESIAN_POINT('Origin',(43.0811453810944,77.1117683798101,210.6));
#36299=CARTESIAN_POINT('Origin',(50.0785666549903,74.1079361245165,211.8));
#36300=CARTESIAN_POINT('',(47.2162408553341,75.3366668562564,210.6));
#36301=CARTESIAN_POINT('',(50.0785666549903,74.1079361245165,210.6));
#36302=CARTESIAN_POINT('',(50.0785666549903,74.1079361245165,210.6));
#36303=CARTESIAN_POINT('',(50.0785666549903,74.1079361245165,211.8));
#36304=CARTESIAN_POINT('',(50.0785666549903,74.1079361245165,211.8));
#36305=CARTESIAN_POINT('',(47.2162408553341,75.3366668562564,211.8));
#36306=CARTESIAN_POINT('',(50.0785666549903,74.1079361245165,211.8));
#36307=CARTESIAN_POINT('',(47.2162408553341,75.3366668562564,211.8));
#36308=CARTESIAN_POINT('Origin',(43.0811453810944,77.1117683798101,211.8));
#36309=CARTESIAN_POINT('',(44.9906970300894,81.1865214397907,211.8));
#36310=CARTESIAN_POINT('Origin',(43.0811453810944,77.1117683798101,211.8));
#36311=CARTESIAN_POINT('',(44.9906970300894,81.1865214397907,210.6));
#36312=CARTESIAN_POINT('',(44.9906970300894,81.1865214397907,211.8));
#36313=CARTESIAN_POINT('Origin',(43.0811453810944,77.1117683798101,210.6));
#36314=CARTESIAN_POINT('Origin',(44.9906970300894,81.1865214397907,211.8));
#36315=CARTESIAN_POINT('',(57.6817429296641,75.6575754701734,210.6));
#36316=CARTESIAN_POINT('',(44.9906970300894,81.1865214397907,210.6));
#36317=CARTESIAN_POINT('',(57.6817429296641,75.6575754701734,211.8));
#36318=CARTESIAN_POINT('',(44.9906970300894,81.1865214397907,211.8));
#36319=CARTESIAN_POINT('',(57.6817429296641,75.6575754701734,211.8));
#36320=CARTESIAN_POINT('Origin',(57.6817429296641,75.6575754701734,211.8));
#36321=CARTESIAN_POINT('',(59.0214390284855,73.5468375985269,210.6));
#36322=CARTESIAN_POINT('',(57.6817429296641,75.6575754701734,210.6));
#36323=CARTESIAN_POINT('',(59.0214390284855,73.5468375985269,211.8));
#36324=CARTESIAN_POINT('',(57.6817429296641,75.6575754701734,211.8));
#36325=CARTESIAN_POINT('',(59.0214390284855,73.5468375985269,211.8));
#36326=CARTESIAN_POINT('Origin',(59.0214390284855,73.5468375985269,211.8));
#36327=CARTESIAN_POINT('',(61.3888699102512,74.0630844855977,210.6));
#36328=CARTESIAN_POINT('',(59.0214390284855,73.5468375985269,210.6));
#36329=CARTESIAN_POINT('',(61.3888699102512,74.0630844855977,211.8));
#36330=CARTESIAN_POINT('',(59.0214390284855,73.5468375985269,211.8));
#36331=CARTESIAN_POINT('',(61.3888699102512,74.0630844855977,211.8));
#36332=CARTESIAN_POINT('Origin',(61.3888699102512,74.0630844855977,211.8));
#36333=CARTESIAN_POINT('',(60.8221863677775,72.7623289912252,210.6));
#36334=CARTESIAN_POINT('',(61.3888699102512,74.0630844855977,210.6));
#36335=CARTESIAN_POINT('',(60.8221863677775,72.7623289912252,211.8));
#36336=CARTESIAN_POINT('',(61.3888699102512,74.0630844855977,211.8));
#36337=CARTESIAN_POINT('',(60.8221863677775,72.7623289912252,211.8));
#36338=CARTESIAN_POINT('Origin',(60.8221863677775,72.7623289912252,211.8));
#36339=CARTESIAN_POINT('',(61.1303665930493,72.6323913325213,210.6));
#36340=CARTESIAN_POINT('',(60.8221863677775,72.7623289912252,210.6));
#36341=CARTESIAN_POINT('',(61.1303665930493,72.6323913325213,211.8));
#36342=CARTESIAN_POINT('',(60.8221863677775,72.7623289912252,211.8));
#36343=CARTESIAN_POINT('',(61.1303665930493,72.6323913325213,211.8));
#36344=CARTESIAN_POINT('Origin',(61.1303665930493,72.6323913325213,211.8));
#36345=CARTESIAN_POINT('',(63.4977974748151,73.148638219592,210.6));
#36346=CARTESIAN_POINT('',(61.1303665930493,72.6323913325213,210.6));
#36347=CARTESIAN_POINT('',(63.4977974748151,73.148638219592,211.8));
#36348=CARTESIAN_POINT('',(61.1303665930493,72.6323913325213,211.8));
#36349=CARTESIAN_POINT('',(63.4977974748151,73.148638219592,211.8));
#36350=CARTESIAN_POINT('Origin',(63.4977974748151,73.148638219592,211.8));
#36351=CARTESIAN_POINT('',(62.9311139323413,71.8478827252195,210.6));
#36352=CARTESIAN_POINT('',(63.4977974748151,73.148638219592,210.6));
#36353=CARTESIAN_POINT('',(62.9311139323413,71.8478827252195,211.8));
#36354=CARTESIAN_POINT('',(63.4977974748151,73.148638219592,211.8));
#36355=CARTESIAN_POINT('',(62.9311139323413,71.8478827252195,211.8));
#36356=CARTESIAN_POINT('Origin',(62.9311139323413,71.8478827252195,211.8));
#36357=CARTESIAN_POINT('',(63.2392941576131,71.7179450665156,210.6));
#36358=CARTESIAN_POINT('',(62.9311139323413,71.8478827252195,210.6));
#36359=CARTESIAN_POINT('',(63.2392941576131,71.7179450665156,211.8));
#36360=CARTESIAN_POINT('',(62.9311139323413,71.8478827252195,211.8));
#36361=CARTESIAN_POINT('',(63.2392941576131,71.7179450665156,211.8));
#36362=CARTESIAN_POINT('Origin',(63.2392941576131,71.7179450665156,211.8));
#36363=CARTESIAN_POINT('',(65.6067250393788,72.2341919535864,210.6));
#36364=CARTESIAN_POINT('',(63.2392941576131,71.7179450665156,210.6));
#36365=CARTESIAN_POINT('',(65.6067250393788,72.2341919535864,211.8));
#36366=CARTESIAN_POINT('',(63.2392941576131,71.7179450665156,211.8));
#36367=CARTESIAN_POINT('',(65.6067250393788,72.2341919535864,211.8));
#36368=CARTESIAN_POINT('Origin',(65.6067250393788,72.2341919535864,211.8));
#36369=CARTESIAN_POINT('',(65.040041496905,70.9334364592139,210.6));
#36370=CARTESIAN_POINT('',(65.6067250393788,72.2341919535864,210.6));
#36371=CARTESIAN_POINT('',(65.040041496905,70.9334364592139,211.8));
#36372=CARTESIAN_POINT('',(65.6067250393788,72.2341919535864,211.8));
#36373=CARTESIAN_POINT('',(65.040041496905,70.9334364592139,211.8));
#36374=CARTESIAN_POINT('Origin',(65.040041496905,70.9334364592139,211.8));
#36375=CARTESIAN_POINT('',(65.3482217221768,70.8034988005099,210.6));
#36376=CARTESIAN_POINT('',(65.040041496905,70.9334364592139,210.6));
#36377=CARTESIAN_POINT('',(65.3482217221768,70.8034988005099,211.8));
#36378=CARTESIAN_POINT('',(65.040041496905,70.9334364592139,211.8));
#36379=CARTESIAN_POINT('',(65.3482217221768,70.8034988005099,211.8));
#36380=CARTESIAN_POINT('Origin',(65.3482217221768,70.8034988005099,211.8));
#36381=CARTESIAN_POINT('',(67.7156526039426,71.3197456875807,210.6));
#36382=CARTESIAN_POINT('',(65.3482217221768,70.8034988005099,210.6));
#36383=CARTESIAN_POINT('',(67.7156526039426,71.3197456875807,211.8));
#36384=CARTESIAN_POINT('',(65.3482217221768,70.8034988005099,211.8));
#36385=CARTESIAN_POINT('',(67.7156526039426,71.3197456875807,211.8));
#36386=CARTESIAN_POINT('Origin',(67.7156526039426,71.3197456875807,211.8));
#36387=CARTESIAN_POINT('',(67.1489690614688,70.0189901932082,210.6));
#36388=CARTESIAN_POINT('',(67.7156526039426,71.3197456875807,210.6));
#36389=CARTESIAN_POINT('',(67.1489690614688,70.0189901932082,211.8));
#36390=CARTESIAN_POINT('',(67.7156526039426,71.3197456875807,211.8));
#36391=CARTESIAN_POINT('',(67.1489690614688,70.0189901932082,211.8));
#36392=CARTESIAN_POINT('Origin',(67.1489690614688,70.0189901932082,211.8));
#36393=CARTESIAN_POINT('',(67.4571492867406,69.8890525345043,210.6));
#36394=CARTESIAN_POINT('',(67.1489690614688,70.0189901932082,210.6));
#36395=CARTESIAN_POINT('',(67.4571492867406,69.8890525345043,211.8));
#36396=CARTESIAN_POINT('',(67.1489690614688,70.0189901932082,211.8));
#36397=CARTESIAN_POINT('',(67.4571492867406,69.8890525345043,211.8));
#36398=CARTESIAN_POINT('Origin',(67.4571492867406,69.8890525345043,211.8));
#36399=CARTESIAN_POINT('',(69.8245801685064,70.4052994215751,210.6));
#36400=CARTESIAN_POINT('',(67.4571492867406,69.8890525345043,210.6));
#36401=CARTESIAN_POINT('',(69.8245801685064,70.4052994215751,211.8));
#36402=CARTESIAN_POINT('',(67.4571492867406,69.8890525345043,211.8));
#36403=CARTESIAN_POINT('',(69.8245801685064,70.4052994215751,211.8));
#36404=CARTESIAN_POINT('Origin',(69.8245801685064,70.4052994215751,211.8));
#36405=CARTESIAN_POINT('',(69.2578966260326,69.1045439272026,210.6));
#36406=CARTESIAN_POINT('',(69.8245801685064,70.4052994215751,210.6));
#36407=CARTESIAN_POINT('',(69.2578966260326,69.1045439272026,211.8));
#36408=CARTESIAN_POINT('',(69.8245801685064,70.4052994215751,211.8));
#36409=CARTESIAN_POINT('',(69.2578966260326,69.1045439272026,211.8));
#36410=CARTESIAN_POINT('Origin',(69.2578966260326,69.1045439272026,211.8));
#36411=CARTESIAN_POINT('',(69.5660768513044,68.9746062684986,210.6));
#36412=CARTESIAN_POINT('',(69.2578966260326,69.1045439272026,210.6));
#36413=CARTESIAN_POINT('',(69.5660768513044,68.9746062684986,211.8));
#36414=CARTESIAN_POINT('',(69.2578966260326,69.1045439272026,211.8));
#36415=CARTESIAN_POINT('',(69.5660768513044,68.9746062684986,211.8));
#36416=CARTESIAN_POINT('Origin',(69.5660768513044,68.9746062684986,211.8));
#36417=CARTESIAN_POINT('',(71.9335077330702,69.4908531555695,210.6));
#36418=CARTESIAN_POINT('',(69.5660768513044,68.9746062684986,210.6));
#36419=CARTESIAN_POINT('',(71.9335077330702,69.4908531555695,211.8));
#36420=CARTESIAN_POINT('',(69.5660768513044,68.9746062684986,211.8));
#36421=CARTESIAN_POINT('',(71.9335077330702,69.4908531555695,211.8));
#36422=CARTESIAN_POINT('Origin',(71.9335077330702,69.4908531555695,211.8));
#36423=CARTESIAN_POINT('',(71.3668241905964,68.1900976611969,210.6));
#36424=CARTESIAN_POINT('',(71.9335077330702,69.4908531555695,210.6));
#36425=CARTESIAN_POINT('',(71.3668241905964,68.1900976611969,211.8));
#36426=CARTESIAN_POINT('',(71.9335077330702,69.4908531555695,211.8));
#36427=CARTESIAN_POINT('',(71.3668241905964,68.1900976611969,211.8));
#36428=CARTESIAN_POINT('Origin',(71.3668241905964,68.1900976611969,211.8));
#36429=CARTESIAN_POINT('',(71.6750044158682,68.060160002493,210.6));
#36430=CARTESIAN_POINT('',(71.3668241905964,68.1900976611969,210.6));
#36431=CARTESIAN_POINT('',(71.6750044158682,68.060160002493,211.8));
#36432=CARTESIAN_POINT('',(71.3668241905964,68.1900976611969,211.8));
#36433=CARTESIAN_POINT('',(71.6750044158682,68.060160002493,211.8));
#36434=CARTESIAN_POINT('Origin',(71.6750044158682,68.060160002493,211.8));
#36435=CARTESIAN_POINT('',(74.042435297634,68.5764068895638,210.6));
#36436=CARTESIAN_POINT('',(71.6750044158682,68.060160002493,210.6));
#36437=CARTESIAN_POINT('',(74.042435297634,68.5764068895638,211.8));
#36438=CARTESIAN_POINT('',(71.6750044158682,68.060160002493,211.8));
#36439=CARTESIAN_POINT('',(74.042435297634,68.5764068895638,211.8));
#36440=CARTESIAN_POINT('Origin',(74.042435297634,68.5764068895638,211.8));
#36441=CARTESIAN_POINT('',(73.4757517551602,67.2756513951913,210.6));
#36442=CARTESIAN_POINT('',(74.042435297634,68.5764068895638,210.6));
#36443=CARTESIAN_POINT('',(73.4757517551602,67.2756513951913,211.8));
#36444=CARTESIAN_POINT('',(74.042435297634,68.5764068895638,211.8));
#36445=CARTESIAN_POINT('',(73.4757517551602,67.2756513951913,211.8));
#36446=CARTESIAN_POINT('Origin',(73.4757517551602,67.2756513951913,211.8));
#36447=CARTESIAN_POINT('',(73.783931980432,67.1457137364874,210.6));
#36448=CARTESIAN_POINT('',(73.4757517551602,67.2756513951913,210.6));
#36449=CARTESIAN_POINT('',(73.783931980432,67.1457137364874,211.8));
#36450=CARTESIAN_POINT('',(73.4757517551602,67.2756513951913,211.8));
#36451=CARTESIAN_POINT('',(73.783931980432,67.1457137364874,211.8));
#36452=CARTESIAN_POINT('Origin',(73.783931980432,67.1457137364874,211.8));
#36453=CARTESIAN_POINT('',(76.1513628621978,67.6619606235582,210.6));
#36454=CARTESIAN_POINT('',(73.783931980432,67.1457137364874,210.6));
#36455=CARTESIAN_POINT('',(76.1513628621978,67.6619606235582,211.8));
#36456=CARTESIAN_POINT('',(73.783931980432,67.1457137364874,211.8));
#36457=CARTESIAN_POINT('',(76.1513628621978,67.6619606235582,211.8));
#36458=CARTESIAN_POINT('Origin',(76.1513628621978,67.6619606235582,211.8));
#36459=CARTESIAN_POINT('',(75.584679319724,66.3612051291856,210.6));
#36460=CARTESIAN_POINT('',(76.1513628621978,67.6619606235582,210.6));
#36461=CARTESIAN_POINT('',(75.584679319724,66.3612051291856,211.8));
#36462=CARTESIAN_POINT('',(76.1513628621978,67.6619606235582,211.8));
#36463=CARTESIAN_POINT('',(75.584679319724,66.3612051291856,211.8));
#36464=CARTESIAN_POINT('Origin',(75.584679319724,66.3612051291856,211.8));
#36465=CARTESIAN_POINT('',(75.8928595449958,66.2312674704817,210.6));
#36466=CARTESIAN_POINT('',(75.584679319724,66.3612051291856,210.6));
#36467=CARTESIAN_POINT('',(75.8928595449958,66.2312674704817,211.8));
#36468=CARTESIAN_POINT('',(75.584679319724,66.3612051291856,211.8));
#36469=CARTESIAN_POINT('',(75.8928595449958,66.2312674704817,211.8));
#36470=CARTESIAN_POINT('Origin',(75.8928595449958,66.2312674704817,211.8));
#36471=CARTESIAN_POINT('',(78.2602904267616,66.7475143575525,210.6));
#36472=CARTESIAN_POINT('',(75.8928595449958,66.2312674704817,210.6));
#36473=CARTESIAN_POINT('',(78.2602904267616,66.7475143575525,211.8));
#36474=CARTESIAN_POINT('',(75.8928595449958,66.2312674704817,211.8));
#36475=CARTESIAN_POINT('',(78.2602904267616,66.7475143575525,211.8));
#36476=CARTESIAN_POINT('Origin',(78.2602904267616,66.7475143575525,211.8));
#36477=CARTESIAN_POINT('',(77.6936068842878,65.44675886318,210.6));
#36478=CARTESIAN_POINT('',(78.2602904267616,66.7475143575525,210.6));
#36479=CARTESIAN_POINT('',(77.6936068842878,65.44675886318,211.8));
#36480=CARTESIAN_POINT('',(78.2602904267616,66.7475143575525,211.8));
#36481=CARTESIAN_POINT('',(77.6936068842878,65.44675886318,211.8));
#36482=CARTESIAN_POINT('Origin',(77.6936068842878,65.44675886318,211.8));
#36483=CARTESIAN_POINT('',(78.0017871095596,65.3168212044761,210.6));
#36484=CARTESIAN_POINT('',(77.6936068842878,65.44675886318,210.6));
#36485=CARTESIAN_POINT('',(78.0017871095596,65.3168212044761,211.8));
#36486=CARTESIAN_POINT('',(77.6936068842878,65.44675886318,211.8));
#36487=CARTESIAN_POINT('',(78.0017871095596,65.3168212044761,211.8));
#36488=CARTESIAN_POINT('Origin',(78.0017871095596,65.3168212044761,211.8));
#36489=CARTESIAN_POINT('',(80.3692179913253,65.8330680915469,210.6));
#36490=CARTESIAN_POINT('',(78.0017871095596,65.3168212044761,210.6));
#36491=CARTESIAN_POINT('',(80.3692179913253,65.8330680915469,211.8));
#36492=CARTESIAN_POINT('',(78.0017871095596,65.3168212044761,211.8));
#36493=CARTESIAN_POINT('',(80.3692179913253,65.8330680915469,211.8));
#36494=CARTESIAN_POINT('Origin',(80.3692179913253,65.8330680915469,211.8));
#36495=CARTESIAN_POINT('',(79.8025344488516,64.5323125971744,210.6));
#36496=CARTESIAN_POINT('',(80.3692179913253,65.8330680915469,210.6));
#36497=CARTESIAN_POINT('',(79.8025344488516,64.5323125971744,211.8));
#36498=CARTESIAN_POINT('',(80.3692179913253,65.8330680915469,211.8));
#36499=CARTESIAN_POINT('',(79.8025344488516,64.5323125971744,211.8));
#36500=CARTESIAN_POINT('Origin',(79.8025344488516,64.5323125971744,211.8));
#36501=CARTESIAN_POINT('',(80.1107146741234,64.4023749384704,210.6));
#36502=CARTESIAN_POINT('',(79.8025344488516,64.5323125971744,210.6));
#36503=CARTESIAN_POINT('',(80.1107146741234,64.4023749384704,211.8));
#36504=CARTESIAN_POINT('',(79.8025344488516,64.5323125971744,211.8));
#36505=CARTESIAN_POINT('',(80.1107146741234,64.4023749384704,211.8));
#36506=CARTESIAN_POINT('Origin',(80.1107146741234,64.4023749384704,211.8));
#36507=CARTESIAN_POINT('',(82.4781455558892,64.9186218255412,210.6));
#36508=CARTESIAN_POINT('',(80.1107146741234,64.4023749384704,210.6));
#36509=CARTESIAN_POINT('',(82.4781455558892,64.9186218255412,211.8));
#36510=CARTESIAN_POINT('',(80.1107146741234,64.4023749384704,211.8));
#36511=CARTESIAN_POINT('',(82.4781455558892,64.9186218255412,211.8));
#36512=CARTESIAN_POINT('Origin',(82.4781455558892,64.9186218255412,211.8));
#36513=CARTESIAN_POINT('',(81.9114620134154,63.6178663311687,210.6));
#36514=CARTESIAN_POINT('',(82.4781455558892,64.9186218255412,210.6));
#36515=CARTESIAN_POINT('',(81.9114620134154,63.6178663311687,211.8));
#36516=CARTESIAN_POINT('',(82.4781455558892,64.9186218255412,211.8));
#36517=CARTESIAN_POINT('',(81.9114620134154,63.6178663311687,211.8));
#36518=CARTESIAN_POINT('Origin',(81.9114620134154,63.6178663311687,211.8));
#36519=CARTESIAN_POINT('',(82.2196422386872,63.4879286724648,210.6));
#36520=CARTESIAN_POINT('',(81.9114620134154,63.6178663311687,210.6));
#36521=CARTESIAN_POINT('',(82.2196422386872,63.4879286724648,211.8));
#36522=CARTESIAN_POINT('',(81.9114620134154,63.6178663311687,211.8));
#36523=CARTESIAN_POINT('',(82.2196422386872,63.4879286724648,211.8));
#36524=CARTESIAN_POINT('Origin',(82.2196422386872,63.4879286724648,211.8));
#36525=CARTESIAN_POINT('',(84.5870731204529,64.0041755595356,210.6));
#36526=CARTESIAN_POINT('',(82.2196422386872,63.4879286724648,210.6));
#36527=CARTESIAN_POINT('',(84.5870731204529,64.0041755595356,211.8));
#36528=CARTESIAN_POINT('',(82.2196422386872,63.4879286724648,211.8));
#36529=CARTESIAN_POINT('',(84.5870731204529,64.0041755595356,211.8));
#36530=CARTESIAN_POINT('Origin',(84.5870731204529,64.0041755595356,211.8));
#36531=CARTESIAN_POINT('',(84.0203895779791,62.7034200651631,210.6));
#36532=CARTESIAN_POINT('',(84.5870731204529,64.0041755595356,210.6));
#36533=CARTESIAN_POINT('',(84.0203895779791,62.7034200651631,211.8));
#36534=CARTESIAN_POINT('',(84.5870731204529,64.0041755595356,211.8));
#36535=CARTESIAN_POINT('',(84.0203895779791,62.7034200651631,211.8));
#36536=CARTESIAN_POINT('Origin',(84.0203895779791,62.7034200651631,211.8));
#36537=CARTESIAN_POINT('',(84.983313171664,62.2363592862195,210.6));
#36538=CARTESIAN_POINT('',(84.0203895779791,62.7034200651631,210.6));
#36539=CARTESIAN_POINT('',(84.983313171664,62.2363592862195,211.8));
#36540=CARTESIAN_POINT('',(84.0203895779791,62.7034200651631,211.8));
#36541=CARTESIAN_POINT('',(84.983313171664,62.2363592862195,211.8));
#36542=CARTESIAN_POINT('Origin',(81.1139782547789,63.6271067952341,211.8));
#36543=CARTESIAN_POINT('',(79.6224513102927,59.7954911168644,210.6));
#36544=CARTESIAN_POINT('Origin',(81.1139782547789,63.6271067952341,210.6));
#36545=CARTESIAN_POINT('',(79.6224513102927,59.7954911168644,211.8));
#36546=CARTESIAN_POINT('Origin',(81.1139782547789,63.6271067952341,211.8));
#36547=CARTESIAN_POINT('',(79.6224513102927,59.7954911168644,211.8));
#36548=CARTESIAN_POINT('Origin',(79.6224513102927,59.7954911168644,211.8));
#36549=CARTESIAN_POINT('',(52.2391399600025,71.7252288329682,210.6));
#36550=CARTESIAN_POINT('',(79.6224513102927,59.7954911168644,210.6));
#36551=CARTESIAN_POINT('',(52.2391399600025,71.7252288329682,211.8));
#36552=CARTESIAN_POINT('',(79.6224513102927,59.7954911168644,211.8));
#36553=CARTESIAN_POINT('',(52.2391399600025,71.7252288329682,211.8));
#36554=CARTESIAN_POINT('Origin',(52.2391399600025,71.7252288329682,211.8));
#36555=CARTESIAN_POINT('',(52.2391399600025,71.7252288329682,210.6));
#36556=CARTESIAN_POINT('',(52.2391399600025,71.7252288329682,211.8));
#36557=CARTESIAN_POINT('Origin',(43.0811453810944,77.1117683798101,210.6));
#36558=CARTESIAN_POINT('Origin',(43.0811453810944,77.1117683798101,211.8));
#36559=CARTESIAN_POINT('Origin',(43.0811453810944,77.1117683798101,212.));
#36654=UNCERTAINTY_MEASURE_WITH_UNIT(LENGTH_MEASURE(0.01),#36669,
'DISTANCE_ACCURACY_VALUE',
'Maximum model space distance between geometric entities at asserted c
onnectivities');
#36656=UNCERTAINTY_MEASURE_WITH_UNIT(LENGTH_MEASURE(0.01),#36669,
'DISTANCE_ACCURACY_VALUE',
'Maximum model space distance between geometric entities at asserted c
onnectivities');
#36666=(
GEOMETRIC_REPRESENTATION_CONTEXT(3)
GLOBAL_UNCERTAINTY_ASSIGNED_CONTEXT((#36654))
GLOBAL_UNIT_ASSIGNED_CONTEXT((#36669,#36671,#36672))
REPRESENTATION_CONTEXT('','3D')
);
#36668=(
GEOMETRIC_REPRESENTATION_CONTEXT(3)
GLOBAL_UNCERTAINTY_ASSIGNED_CONTEXT((#36656))
GLOBAL_UNIT_ASSIGNED_CONTEXT((#36669,#36671,#36672))
REPRESENTATION_CONTEXT('','3D')
);
#36669=(
LENGTH_UNIT()
NAMED_UNIT(*)
SI_UNIT(.MILLI.,.METRE.)
);
#36671=(
NAMED_UNIT(*)
PLANE_ANGLE_UNIT()
SI_UNIT($,.RADIAN.)
);
#36672=(
NAMED_UNIT(*)
SI_UNIT($,.STERADIAN.)
SOLID_ANGLE_UNIT()
);
#36682=SHAPE_DEFINITION_REPRESENTATION(#36693,#36714);
#36693=PRODUCT_DEFINITION_SHAPE('',$,#36726);
#36714=SHAPE_REPRESENTATION('',(#19168),#36666);
#36716=PRODUCT_DEFINITION_CONTEXT('part definition',#36751,'design');
#36726=PRODUCT_DEFINITION('Tensioner Lever Arm','Tensioner Lever Arm',#36737,
#36716);
#36737=PRODUCT_DEFINITION_FORMATION('',$,#36762);
#36751=APPLICATION_CONTEXT(
'Core Data for Automotive Mechanical Design Process');
#36752=PRODUCT_CONTEXT('part definition',#36751,'mechanical');
#36762=PRODUCT('Tensioner Lever Arm','Tensioner Lever Arm',$,(#36752));
#36770=PRESENTATION_STYLE_ASSIGNMENT((#36777));
#36777=SURFACE_STYLE_USAGE(.BOTH.,#36784);
#36784=SURFACE_SIDE_STYLE('',(#36791));
#36791=SURFACE_STYLE_FILL_AREA(#36798);
#36798=FILL_AREA_STYLE('Opaque(169,212,242)',(#36805));
#36805=FILL_AREA_STYLE_COLOUR('Opaque(169,212,242)',#36812);
#36812=COLOUR_RGB('Opaque(169,212,242)',0.662745098039216,0.831372549019608,
0.949019607843137);
ENDSEC;
END-ISO-10303-21;
